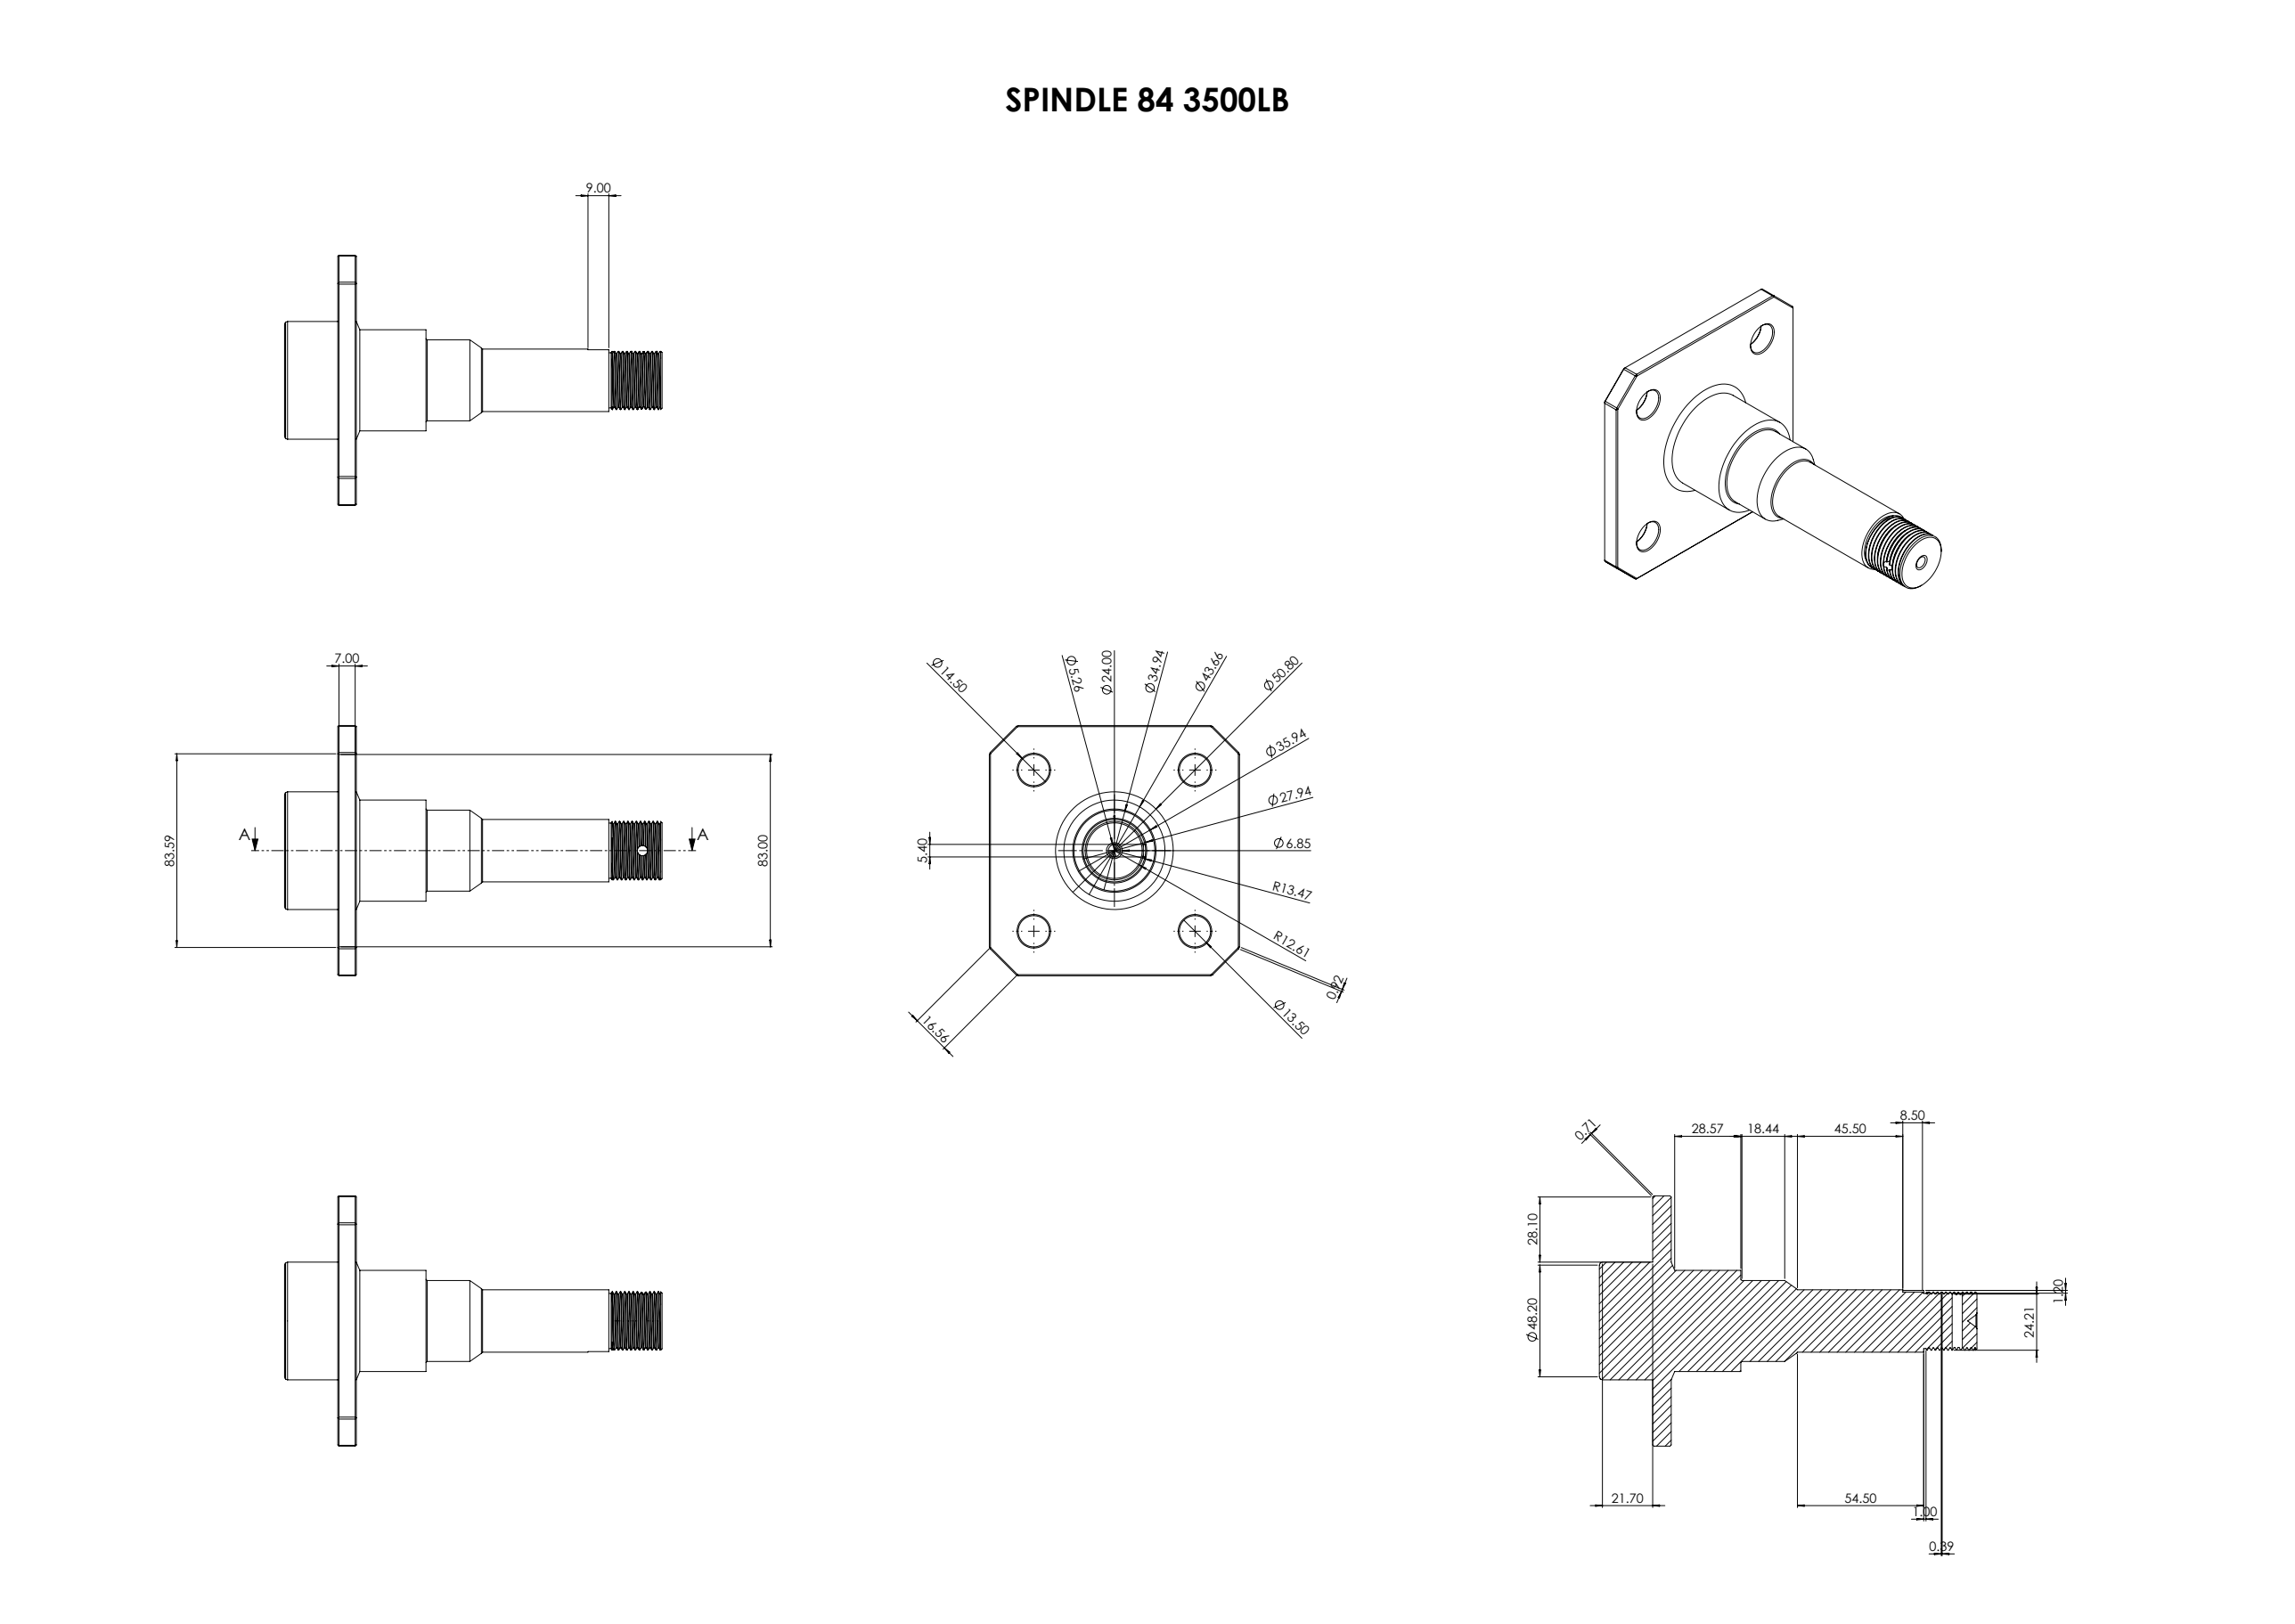
ISO-10303-21;
HEADER;
/* Generated by software containing ST-Developer
 * from STEP Tools, Inc. (www.steptools.com) 
 */

FILE_DESCRIPTION(
/* description */ (''),
/* implementation_level */ '2;1');

FILE_NAME(
/* name */ '10_Spindle_84_3500lb.step',
/* time_stamp */ '2026-10-25T01:26:34-07:00',
/* author */ (''),
/* organization */ (''),
/* preprocessor_version */ 'ST-DEVELOPER v20.2',
/* originating_system */ 'Autodesk Translation Framework v15.15.0.0',
/* authorisation */ '');

FILE_SCHEMA (('AUTOMOTIVE_DESIGN { 1 0 10303 214 3 1 1 }'));
ENDSEC;

DATA;
#10=MECHANICAL_DESIGN_GEOMETRIC_PRESENTATION_REPRESENTATION('',(#322),#71628);
#181=(
BOUNDED_CURVE()
B_SPLINE_CURVE(2,(#57816,#57817,#57818),.UNSPECIFIED.,.F.,.F.)
B_SPLINE_CURVE_WITH_KNOTS((3,3),(0.0552009552934231,0.395576151489963),
 .UNSPECIFIED.)
CURVE()
GEOMETRIC_REPRESENTATION_ITEM()
RATIONAL_B_SPLINE_CURVE((1.00343876873283,1.01256123126711,1.00343876873283))
REPRESENTATION_ITEM('')
);
#182=(
BOUNDED_CURVE()
B_SPLINE_CURVE(2,(#57942,#57943,#57944),.UNSPECIFIED.,.F.,.F.)
B_SPLINE_CURVE_WITH_KNOTS((3,3),(0.0550683626555145,0.394625977980432),
 .UNSPECIFIED.)
CURVE()
GEOMETRIC_REPRESENTATION_ITEM()
RATIONAL_B_SPLINE_CURVE((1.00343876873282,1.01256123126706,1.00343876873282))
REPRESENTATION_ITEM('')
);
#275=B_SPLINE_SURFACE_WITH_KNOTS('',3,3,((#53607,#53608,#53609,#53610,#53611,
#53612,#53613,#53614,#53615),(#53616,#53617,#53618,#53619,#53620,#53621,
#53622,#53623,#53624),(#53625,#53626,#53627,#53628,#53629,#53630,#53631,
#53632,#53633),(#53634,#53635,#53636,#53637,#53638,#53639,#53640,#53641,
#53642)),.UNSPECIFIED.,.F.,.F.,.F.,(4,4),(4,1,1,1,1,1,4),(0.,0.117317574699332),
(58.2563833255769,58.586820436873,59.2476946594652,59.5781317707613,60.2390059933534,
60.8998802159456,61.2303173272417),.UNSPECIFIED.);
#276=B_SPLINE_SURFACE_WITH_KNOTS('',3,3,((#53715,#53716,#53717,#53718,#53719,
#53720,#53721,#53722,#53723,#53724,#53725,#53726,#53727,#53728,#53729,#53730,
#53731,#53732,#53733,#53734,#53735,#53736,#53737,#53738,#53739,#53740,#53741,
#53742,#53743,#53744,#53745,#53746,#53747,#53748,#53749,#53750,#53751,#53752,
#53753,#53754,#53755,#53756,#53757,#53758,#53759,#53760,#53761),(#53762,
#53763,#53764,#53765,#53766,#53767,#53768,#53769,#53770,#53771,#53772,#53773,
#53774,#53775,#53776,#53777,#53778,#53779,#53780,#53781,#53782,#53783,#53784,
#53785,#53786,#53787,#53788,#53789,#53790,#53791,#53792,#53793,#53794,#53795,
#53796,#53797,#53798,#53799,#53800,#53801,#53802,#53803,#53804,#53805,#53806,
#53807,#53808),(#53809,#53810,#53811,#53812,#53813,#53814,#53815,#53816,
#53817,#53818,#53819,#53820,#53821,#53822,#53823,#53824,#53825,#53826,#53827,
#53828,#53829,#53830,#53831,#53832,#53833,#53834,#53835,#53836,#53837,#53838,
#53839,#53840,#53841,#53842,#53843,#53844,#53845,#53846,#53847,#53848,#53849,
#53850,#53851,#53852,#53853,#53854,#53855),(#53856,#53857,#53858,#53859,
#53860,#53861,#53862,#53863,#53864,#53865,#53866,#53867,#53868,#53869,#53870,
#53871,#53872,#53873,#53874,#53875,#53876,#53877,#53878,#53879,#53880,#53881,
#53882,#53883,#53884,#53885,#53886,#53887,#53888,#53889,#53890,#53891,#53892,
#53893,#53894,#53895,#53896,#53897,#53898,#53899,#53900,#53901,#53902)),
 .UNSPECIFIED.,.F.,.F.,.F.,(4,4),(4,1,1,1,1,1,1,1,1,1,1,1,1,1,1,1,1,1,1,
1,1,1,1,1,1,1,1,1,1,1,1,1,1,1,1,1,1,1,1,1,1,1,1,1,4),(0.,0.117317574699332),
(61.2845034392321,61.7747737335008,62.2650440277695,62.7553143220381,63.2455846163068,
63.7358549105755,64.2261252048442,64.7163954991129,65.2066657933815,65.6969360876502,
66.1872063819189,66.6774766761876,67.1677469704563,67.6580172647249,68.1482875589936,
68.6385578532623,69.128828147531,69.6190984417997,70.1093687360683,70.599639030337,
71.0899093246057,71.5801796188744,72.0704499131431,72.5607202074117,73.0509905016804,
73.5412607959491,74.0315310902178,74.5218013844865,75.0120716787551,75.5023419730238,
75.9926122672925,76.4828825615612,76.9731528558299,77.4634231500985,77.9536934443672,
78.4439637386359,78.9342340329046,79.4245043271733,79.9147746214419,80.4050449157106,
80.8953152099793,81.385585504248,81.8758557985167,82.3661260927854,82.856396387054),
 .UNSPECIFIED.);
#277=B_SPLINE_SURFACE_WITH_KNOTS('',3,3,((#54341,#54342,#54343,#54344,#54345,
#54346,#54347,#54348,#54349,#54350,#54351,#54352,#54353,#54354,#54355,#54356,
#54357,#54358,#54359,#54360,#54361,#54362,#54363,#54364,#54365,#54366,#54367,
#54368,#54369,#54370,#54371,#54372,#54373,#54374,#54375,#54376,#54377,#54378,
#54379,#54380,#54381,#54382,#54383,#54384,#54385,#54386,#54387,#54388,#54389,
#54390,#54391,#54392,#54393,#54394,#54395,#54396,#54397,#54398,#54399,#54400,
#54401,#54402,#54403,#54404,#54405,#54406,#54407,#54408,#54409,#54410,#54411,
#54412,#54413,#54414,#54415,#54416,#54417,#54418,#54419,#54420,#54421,#54422,
#54423,#54424,#54425),(#54426,#54427,#54428,#54429,#54430,#54431,#54432,
#54433,#54434,#54435,#54436,#54437,#54438,#54439,#54440,#54441,#54442,#54443,
#54444,#54445,#54446,#54447,#54448,#54449,#54450,#54451,#54452,#54453,#54454,
#54455,#54456,#54457,#54458,#54459,#54460,#54461,#54462,#54463,#54464,#54465,
#54466,#54467,#54468,#54469,#54470,#54471,#54472,#54473,#54474,#54475,#54476,
#54477,#54478,#54479,#54480,#54481,#54482,#54483,#54484,#54485,#54486,#54487,
#54488,#54489,#54490,#54491,#54492,#54493,#54494,#54495,#54496,#54497,#54498,
#54499,#54500,#54501,#54502,#54503,#54504,#54505,#54506,#54507,#54508,#54509,
#54510),(#54511,#54512,#54513,#54514,#54515,#54516,#54517,#54518,#54519,
#54520,#54521,#54522,#54523,#54524,#54525,#54526,#54527,#54528,#54529,#54530,
#54531,#54532,#54533,#54534,#54535,#54536,#54537,#54538,#54539,#54540,#54541,
#54542,#54543,#54544,#54545,#54546,#54547,#54548,#54549,#54550,#54551,#54552,
#54553,#54554,#54555,#54556,#54557,#54558,#54559,#54560,#54561,#54562,#54563,
#54564,#54565,#54566,#54567,#54568,#54569,#54570,#54571,#54572,#54573,#54574,
#54575,#54576,#54577,#54578,#54579,#54580,#54581,#54582,#54583,#54584,#54585,
#54586,#54587,#54588,#54589,#54590,#54591,#54592,#54593,#54594,#54595),
(#54596,#54597,#54598,#54599,#54600,#54601,#54602,#54603,#54604,#54605,
#54606,#54607,#54608,#54609,#54610,#54611,#54612,#54613,#54614,#54615,#54616,
#54617,#54618,#54619,#54620,#54621,#54622,#54623,#54624,#54625,#54626,#54627,
#54628,#54629,#54630,#54631,#54632,#54633,#54634,#54635,#54636,#54637,#54638,
#54639,#54640,#54641,#54642,#54643,#54644,#54645,#54646,#54647,#54648,#54649,
#54650,#54651,#54652,#54653,#54654,#54655,#54656,#54657,#54658,#54659,#54660,
#54661,#54662,#54663,#54664,#54665,#54666,#54667,#54668,#54669,#54670,#54671,
#54672,#54673,#54674,#54675,#54676,#54677,#54678,#54679,#54680)),
 .UNSPECIFIED.,.F.,.F.,.F.,(4,4),(4,1,1,1,1,1,1,1,1,1,1,1,1,1,1,1,1,1,1,
1,1,1,1,1,1,1,1,1,1,1,1,1,1,1,1,1,1,1,1,1,1,1,1,1,1,1,1,1,1,1,1,1,1,1,1,
1,1,1,1,1,1,1,1,1,1,1,1,1,1,1,1,1,1,1,1,1,1,1,1,1,1,1,4),(0.,0.117317574699332),
(8.304938233291,8.79653306474967,9.28812789620834,9.77972272766701,10.2713175591257,
10.7629123905843,11.254507222043,11.7461020535017,12.2376968849604,12.729291716419,
13.2208865478777,13.7124813793364,14.204076210795,14.6956710422537,15.1872658737124,
15.678860705171,16.1704555366297,16.6620503680884,17.153645199547,17.6452400310057,
18.1368348624644,18.628429693923,19.1200245253817,19.6116193568404,20.103214188299,
20.5948090197577,21.0864038512164,21.5779986826751,22.0695935141337,22.5611883455924,
23.0527831770511,23.5443780085097,24.0359728399684,24.5275676714271,25.0191625028857,
25.5107573343444,26.0023521658031,26.4939469972617,26.9855418287204,27.4771366601791,
27.9687314916377,28.4603263230964,28.9519211545551,29.4435159860138,29.9351108174724,
30.4267056489311,30.9183004803898,31.4098953118484,31.9014901433071,32.3930849747658,
32.8846798062244,33.3762746376831,33.8678694691418,34.3594643006004,34.8510591320591,
35.3426539635178,35.8342487949764,36.3258436264351,36.8174384578938,37.3090332893524,
37.8006281208111,38.2922229522698,38.7838177837285,39.2754126151871,39.7670074466458,
40.2586022781045,40.7501971095631,41.2417919410218,41.7333867724805,42.2249816039391,
42.7165764353978,43.2081712668565,43.6997660983151,44.1913609297738,44.6829557612325,
45.1745505926911,45.6661454241498,46.1577402556085,46.6493350870672,47.1409299185258,
47.6325247499845,48.1241195814432,48.6157144129018),.UNSPECIFIED.);
#278=B_SPLINE_SURFACE_WITH_KNOTS('',3,3,((#55387,#55388,#55389,#55390,#55391,
#55392,#55393,#55394,#55395),(#55396,#55397,#55398,#55399,#55400,#55401,
#55402,#55403,#55404),(#55405,#55406,#55407,#55408,#55409,#55410,#55411,
#55412,#55413),(#55414,#55415,#55416,#55417,#55418,#55419,#55420,#55421,
#55422)),.UNSPECIFIED.,.F.,.F.,.F.,(4,4),(4,1,1,1,1,1,4),(0.,0.117317574699332),
(48.7821842940486,49.4244050727166,49.7455154620506,50.0666258513846,50.7088466300525,
51.0299570193865,51.6721777980545),.UNSPECIFIED.);
#279=B_SPLINE_SURFACE_WITH_KNOTS('',3,3,((#55476,#55477,#55478,#55479,#55480,
#55481,#55482,#55483,#55484),(#55485,#55486,#55487,#55488,#55489,#55490,
#55491,#55492,#55493),(#55494,#55495,#55496,#55497,#55498,#55499,#55500,
#55501,#55502),(#55503,#55504,#55505,#55506,#55507,#55508,#55509,#55510,
#55511)),.UNSPECIFIED.,.F.,.F.,.F.,(4,4),(4,1,1,1,1,1,4),(0.,0.117317574699332),
(52.0050602882015,52.6272969542447,52.9384152872664,53.249533620288,53.8717702863312,
54.4940069523745,54.8051252853961),.UNSPECIFIED.);
#280=B_SPLINE_SURFACE_WITH_KNOTS('',3,3,((#55573,#55574,#55575,#55576,#55577,
#55578,#55579,#55580,#55581),(#55582,#55583,#55584,#55585,#55586,#55587,
#55588,#55589,#55590),(#55591,#55592,#55593,#55594,#55595,#55596,#55597,
#55598,#55599),(#55600,#55601,#55602,#55603,#55604,#55605,#55606,#55607,
#55608)),.UNSPECIFIED.,.F.,.F.,.F.,(4,4),(4,1,1,1,1,1,4),(0.,0.117317574699332),
(55.1490525302778,55.4633418551201,56.0919205048047,56.7204991544894,57.0347884793317,
57.349077804174,57.9776564538586),.UNSPECIFIED.);
#281=B_SPLINE_SURFACE_WITH_KNOTS('',3,3,((#55670,#55671,#55672,#55673,#55674,
#55675,#55676,#55677,#55678,#55679,#55680,#55681,#55682,#55683,#55684,#55685,
#55686,#55687,#55688,#55689,#55690,#55691,#55692,#55693,#55694,#55695,#55696,
#55697,#55698,#55699,#55700,#55701,#55702,#55703,#55704,#55705,#55706,#55707,
#55708,#55709,#55710,#55711,#55712,#55713,#55714,#55715,#55716),(#55717,
#55718,#55719,#55720,#55721,#55722,#55723,#55724,#55725,#55726,#55727,#55728,
#55729,#55730,#55731,#55732,#55733,#55734,#55735,#55736,#55737,#55738,#55739,
#55740,#55741,#55742,#55743,#55744,#55745,#55746,#55747,#55748,#55749,#55750,
#55751,#55752,#55753,#55754,#55755,#55756,#55757,#55758,#55759,#55760,#55761,
#55762,#55763),(#55764,#55765,#55766,#55767,#55768,#55769,#55770,#55771,
#55772,#55773,#55774,#55775,#55776,#55777,#55778,#55779,#55780,#55781,#55782,
#55783,#55784,#55785,#55786,#55787,#55788,#55789,#55790,#55791,#55792,#55793,
#55794,#55795,#55796,#55797,#55798,#55799,#55800,#55801,#55802,#55803,#55804,
#55805,#55806,#55807,#55808,#55809,#55810),(#55811,#55812,#55813,#55814,
#55815,#55816,#55817,#55818,#55819,#55820,#55821,#55822,#55823,#55824,#55825,
#55826,#55827,#55828,#55829,#55830,#55831,#55832,#55833,#55834,#55835,#55836,
#55837,#55838,#55839,#55840,#55841,#55842,#55843,#55844,#55845,#55846,#55847,
#55848,#55849,#55850,#55851,#55852,#55853,#55854,#55855,#55856,#55857)),
 .UNSPECIFIED.,.F.,.F.,.F.,(4,4),(4,1,1,1,1,1,1,1,1,1,1,1,1,1,1,1,1,1,1,
1,1,1,1,1,1,1,1,1,1,1,1,1,1,1,1,1,1,1,1,1,1,1,1,1,4),(0.,0.117317574699332),
(64.4256593907634,64.920671977511,65.4156845642586,65.9106971510062,66.4057097377538,
66.9007223245014,67.3957349112491,67.8907474979967,68.3857600847443,68.8807726714919,
69.3757852582395,69.8707978449871,70.3658104317347,70.8608230184823,71.3558356052299,
71.8508481919775,72.3458607787251,72.8408733654727,73.3358859522203,73.8308985389679,
74.3259111257155,74.8209237124631,75.3159362992107,75.8109488859583,76.3059614727059,
76.8009740594535,77.2959866462011,77.7909992329487,78.2860118196963,78.7810244064439,
79.2760369931915,79.7710495799391,80.2660621666867,80.7610747534343,81.2560873401819,
81.7510999269296,82.2461125136772,82.7411251004248,83.2361376871724,83.73115027392,
84.2261628606676,84.7211754474152,85.2161880341628,85.7112006209104,86.206213207658),
 .UNSPECIFIED.);
#282=B_SPLINE_SURFACE_WITH_KNOTS('',3,3,((#56291,#56292,#56293,#56294,#56295,
#56296,#56297,#56298,#56299),(#56300,#56301,#56302,#56303,#56304,#56305,
#56306,#56307,#56308),(#56309,#56310,#56311,#56312,#56313,#56314,#56315,
#56316,#56317),(#56318,#56319,#56320,#56321,#56322,#56323,#56324,#56325,
#56326)),.UNSPECIFIED.,.F.,.F.,.F.,(4,4),(4,1,1,1,1,1,4),(0.,0.117317574699332),
(61.413786866147,61.742287519182,62.399288825252,62.727789478287,63.384790784357,
64.041792090427,64.370292743462),.UNSPECIFIED.);
#283=B_SPLINE_SURFACE_WITH_KNOTS('',3,3,((#56383,#56384,#56385,#56386,#56387,
#56388,#56389,#56390,#56391),(#56392,#56393,#56394,#56395,#56396,#56397,
#56398,#56399,#56400),(#56401,#56402,#56403,#56404,#56405,#56406,#56407,
#56408,#56409),(#56410,#56411,#56412,#56413,#56414,#56415,#56416,#56417,
#56418)),.UNSPECIFIED.,.F.,.F.,.F.,(4,4),(4,1,1,1,1,1,4),(0.,0.117317574699332),
(58.294224706896,58.9183499948197,59.2304126387815,59.5424752827434,60.166600570667,
60.7907258585907,61.1027885025526),.UNSPECIFIED.);
#284=B_SPLINE_SURFACE_WITH_KNOTS('',3,3,((#56480,#56481,#56482,#56483,#56484,
#56485,#56486,#56487,#56488,#56489,#56490,#56491,#56492,#56493,#56494,#56495,
#56496,#56497,#56498,#56499,#56500,#56501,#56502,#56503,#56504,#56505,#56506,
#56507,#56508,#56509,#56510,#56511,#56512,#56513,#56514,#56515,#56516,#56517,
#56518,#56519,#56520,#56521,#56522,#56523,#56524,#56525,#56526,#56527,#56528,
#56529,#56530,#56531,#56532,#56533,#56534,#56535,#56536,#56537,#56538,#56539,
#56540,#56541,#56542,#56543,#56544,#56545,#56546,#56547,#56548,#56549,#56550,
#56551,#56552,#56553,#56554,#56555,#56556,#56557,#56558,#56559,#56560,#56561,
#56562,#56563,#56564),(#56565,#56566,#56567,#56568,#56569,#56570,#56571,
#56572,#56573,#56574,#56575,#56576,#56577,#56578,#56579,#56580,#56581,#56582,
#56583,#56584,#56585,#56586,#56587,#56588,#56589,#56590,#56591,#56592,#56593,
#56594,#56595,#56596,#56597,#56598,#56599,#56600,#56601,#56602,#56603,#56604,
#56605,#56606,#56607,#56608,#56609,#56610,#56611,#56612,#56613,#56614,#56615,
#56616,#56617,#56618,#56619,#56620,#56621,#56622,#56623,#56624,#56625,#56626,
#56627,#56628,#56629,#56630,#56631,#56632,#56633,#56634,#56635,#56636,#56637,
#56638,#56639,#56640,#56641,#56642,#56643,#56644,#56645,#56646,#56647,#56648,
#56649),(#56650,#56651,#56652,#56653,#56654,#56655,#56656,#56657,#56658,
#56659,#56660,#56661,#56662,#56663,#56664,#56665,#56666,#56667,#56668,#56669,
#56670,#56671,#56672,#56673,#56674,#56675,#56676,#56677,#56678,#56679,#56680,
#56681,#56682,#56683,#56684,#56685,#56686,#56687,#56688,#56689,#56690,#56691,
#56692,#56693,#56694,#56695,#56696,#56697,#56698,#56699,#56700,#56701,#56702,
#56703,#56704,#56705,#56706,#56707,#56708,#56709,#56710,#56711,#56712,#56713,
#56714,#56715,#56716,#56717,#56718,#56719,#56720,#56721,#56722,#56723,#56724,
#56725,#56726,#56727,#56728,#56729,#56730,#56731,#56732,#56733,#56734),
(#56735,#56736,#56737,#56738,#56739,#56740,#56741,#56742,#56743,#56744,
#56745,#56746,#56747,#56748,#56749,#56750,#56751,#56752,#56753,#56754,#56755,
#56756,#56757,#56758,#56759,#56760,#56761,#56762,#56763,#56764,#56765,#56766,
#56767,#56768,#56769,#56770,#56771,#56772,#56773,#56774,#56775,#56776,#56777,
#56778,#56779,#56780,#56781,#56782,#56783,#56784,#56785,#56786,#56787,#56788,
#56789,#56790,#56791,#56792,#56793,#56794,#56795,#56796,#56797,#56798,#56799,
#56800,#56801,#56802,#56803,#56804,#56805,#56806,#56807,#56808,#56809,#56810,
#56811,#56812,#56813,#56814,#56815,#56816,#56817,#56818,#56819)),
 .UNSPECIFIED.,.F.,.F.,.F.,(4,4),(4,1,1,1,1,1,1,1,1,1,1,1,1,1,1,1,1,1,1,
1,1,1,1,1,1,1,1,1,1,1,1,1,1,1,1,1,1,1,1,1,1,1,1,1,1,1,1,1,1,1,1,1,1,1,1,
1,1,1,1,1,1,1,1,1,1,1,1,1,1,1,1,1,1,1,1,1,1,1,1,1,1,1,4),(0.,0.117317574699332),
(11.654755053895,12.1440162165507,12.6332773792065,13.1225385418623,13.611799704518,
14.1010608671738,14.5903220298296,15.0795831924853,15.5688443551411,16.0581055177969,
16.5473666804527,17.0366278431084,17.5258890057642,18.01515016842,18.5044113310757,
18.9936724937315,19.4829336563873,19.972194819043,20.4614559816988,20.9507171443546,
21.4399783070103,21.9292394696661,22.4185006323219,22.9077617949777,23.3970229576334,
23.8862841202892,24.375545282945,24.8648064456007,25.3540676082565,25.8433287709123,
26.332589933568,26.8218510962238,27.3111122588796,27.8003734215353,28.2896345841911,
28.7788957468469,29.2681569095027,29.7574180721584,30.2466792348142,30.73594039747,
31.2252015601257,31.7144627227815,32.2037238854373,32.692985048093,33.1822462107488,
33.6715073734046,34.1607685360603,34.6500296987161,35.1392908613719,35.6285520240277,
36.1178131866834,36.6070743493392,37.096335511995,37.5855966746507,38.0748578373065,
38.5641189999623,39.053380162618,39.5426413252738,40.0319024879296,40.5211636505854,
41.0104248132411,41.4996859758969,41.9889471385527,42.4782083012084,42.9674694638642,
43.45673062652,43.9459917891757,44.4352529518315,44.9245141144873,45.413775277143,
45.9030364397988,46.3922976024546,46.8815587651103,47.3708199277661,47.8600810904219,
48.3493422530777,48.8386034157334,49.3278645783892,49.817125741045,50.3063869037007,
50.7956480663565,51.2849092290123,51.774170391668),.UNSPECIFIED.);
#285=B_SPLINE_SURFACE_WITH_KNOTS('',3,3,((#57528,#57529,#57530,#57531,#57532,
#57533,#57534,#57535,#57536),(#57537,#57538,#57539,#57540,#57541,#57542,
#57543,#57544,#57545),(#57546,#57547,#57548,#57549,#57550,#57551,#57552,
#57553,#57554),(#57555,#57556,#57557,#57558,#57559,#57560,#57561,#57562,
#57563)),.UNSPECIFIED.,.F.,.F.,.F.,(4,4),(4,1,1,1,1,1,4),(0.,0.117317574699332),
(51.9058023205642,52.230691972308,52.8804712757956,53.2053609275394,53.855140231027,
54.1800298827708,54.8298091862584),.UNSPECIFIED.);
#286=B_SPLINE_SURFACE_WITH_KNOTS('',3,3,((#57698,#57699,#57700,#57701,#57702,
#57703,#57704,#57705,#57706),(#57707,#57708,#57709,#57710,#57711,#57712,
#57713,#57714,#57715),(#57716,#57717,#57718,#57719,#57720,#57721,#57722,
#57723,#57724),(#57725,#57726,#57727,#57728,#57729,#57730,#57731,#57732,
#57733)),.UNSPECIFIED.,.F.,.F.,.F.,(4,4),(4,1,1,1,1,1,4),(0.,0.117317574699332),
(55.1300987113493,55.4429246232081,56.0685764469255,56.3814023587843,57.0070541825018,
57.3198800943605,57.945531918078),.UNSPECIFIED.);
#296=SHAPE_REPRESENTATION_RELATIONSHIP('SRR','None',#71684,#309);
#309=ADVANCED_BREP_SHAPE_REPRESENTATION('',(#335),#71616);
#322=STYLED_ITEM('',(#71804),#335);
#335=MANIFOLD_SOLID_BREP('Body1',#34209);
#357=B_SPLINE_CURVE_WITH_KNOTS('',3,(#52958,#52959,#52960,#52961,#52962,
#52963,#52964,#52965,#52966,#52967,#52968,#52969,#52970),.UNSPECIFIED.,
 .F.,.F.,(4,1,1,1,1,1,1,1,1,1,4),(47.1238898038469,47.3708199277661,47.8600810904219,
48.3493422530777,48.8386034157334,49.3278645783892,49.817125741045,50.3063869037007,
50.7956480663565,51.2849092290123,51.6964060964814),.UNSPECIFIED.);
#358=B_SPLINE_CURVE_WITH_KNOTS('',3,(#52972,#52973,#52974,#52975),
 .UNSPECIFIED.,.F.,.F.,(4,4),(0.11224113270863,0.157354351022216),
 .UNSPECIFIED.);
#359=B_SPLINE_CURVE_WITH_KNOTS('',3,(#52977,#52978,#52979,#52980,#52981,
#52982,#52983,#52984,#52985),.UNSPECIFIED.,.F.,.F.,(4,1,1,1,1,1,4),(48.7821842940486,
49.4244050727166,49.7455154620506,50.0666258513846,50.7088466300525,51.0299570193865,
51.6721777980545),.UNSPECIFIED.);
#360=B_SPLINE_CURVE_WITH_KNOTS('',3,(#52987,#52988,#52989,#52990,#52991,
#52992),.UNSPECIFIED.,.F.,.F.,(4,2,4),(0.997055295420078,1.08014136000988,
1.09793883659407),.UNSPECIFIED.);
#361=B_SPLINE_CURVE_WITH_KNOTS('',3,(#52994,#52995,#52996,#52997,#52998,
#52999),.UNSPECIFIED.,.F.,.F.,(4,2,4),(0.906540457062692,0.913969230830279,
0.997055295420078),.UNSPECIFIED.);
#362=B_SPLINE_CURVE_WITH_KNOTS('',3,(#53000,#53001,#53002,#53003,#53004,
#53005,#53006),.UNSPECIFIED.,.F.,.F.,(4,1,1,1,4),(47.1238898038469,47.1409299185258,
47.6325247499845,48.1241195814432,48.6157144129018),.UNSPECIFIED.);
#363=B_SPLINE_CURVE_WITH_KNOTS('',3,(#53011,#53012,#53013,#53014,#53015,
#53016,#53017,#53018,#53019,#53020,#53021,#53022,#53023,#53024,#53025,#53026,
#53027),.UNSPECIFIED.,.F.,.F.,(4,1,1,1,1,1,1,1,1,1,1,1,1,1,4),(40.8407044966673,
41.0104248132411,41.4996859758969,41.9889471385527,42.4782083012084,42.9674694638642,
43.45673062652,43.9459917891757,44.4352529518315,44.9245141144873,45.413775277143,
45.9030364397988,46.3922976024546,46.8815587651103,47.1238898038469),
 .UNSPECIFIED.);
#364=B_SPLINE_CURVE_WITH_KNOTS('',3,(#53028,#53029,#53030,#53031,#53032,
#53033,#53034,#53035,#53036,#53037,#53038,#53039,#53040,#53041,#53042,#53043),
 .UNSPECIFIED.,.F.,.F.,(4,1,1,1,1,1,1,1,1,1,1,1,1,4),(40.8407044966673,
41.2417919410218,41.7333867724805,42.2249816039391,42.7165764353978,43.2081712668565,
43.6997660983151,44.1913609297738,44.6829557612325,45.1745505926911,45.6661454241498,
46.1577402556085,46.6493350870672,47.1238898038469),.UNSPECIFIED.);
#365=B_SPLINE_CURVE_WITH_KNOTS('',3,(#53048,#53049,#53050,#53051,#53052,
#53053,#53054,#53055,#53056,#53057,#53058,#53059,#53060,#53061,#53062,#53063,
#53064),.UNSPECIFIED.,.F.,.F.,(4,1,1,1,1,1,1,1,1,1,1,1,1,1,4),(34.5575191894877,
34.6500296987161,35.1392908613719,35.6285520240277,36.1178131866834,36.6070743493392,
37.096335511995,37.5855966746507,38.0748578373065,38.5641189999623,39.053380162618,
39.5426413252738,40.0319024879296,40.5211636505854,40.8407044966673),
 .UNSPECIFIED.);
#366=B_SPLINE_CURVE_WITH_KNOTS('',3,(#53065,#53066,#53067,#53068,#53069,
#53070,#53071,#53072,#53073,#53074,#53075,#53076,#53077,#53078,#53079,#53080,
#53081),.UNSPECIFIED.,.F.,.F.,(4,1,1,1,1,1,1,1,1,1,1,1,1,1,4),(34.5575191894877,
34.8510591320591,35.3426539635178,35.8342487949764,36.3258436264351,36.8174384578938,
37.3090332893524,37.8006281208111,38.2922229522698,38.7838177837285,39.2754126151871,
39.7670074466458,40.2586022781045,40.7501971095631,40.8407044966673),
 .UNSPECIFIED.);
#367=B_SPLINE_CURVE_WITH_KNOTS('',3,(#53086,#53087,#53088,#53089,#53090,
#53091,#53092,#53093,#53094,#53095,#53096,#53097,#53098,#53099,#53100,#53101,
#53102),.UNSPECIFIED.,.F.,.F.,(4,1,1,1,1,1,1,1,1,1,1,1,1,1,4),(28.2743338823081,
28.2896345841911,28.7788957468469,29.2681569095027,29.7574180721584,30.2466792348142,
30.73594039747,31.2252015601257,31.7144627227815,32.2037238854373,32.692985048093,
33.1822462107488,33.6715073734046,34.1607685360603,34.5575191894877),
 .UNSPECIFIED.);
#368=B_SPLINE_CURVE_WITH_KNOTS('',3,(#53103,#53104,#53105,#53106,#53107,
#53108,#53109,#53110,#53111,#53112,#53113,#53114,#53115,#53116,#53117,#53118,
#53119),.UNSPECIFIED.,.F.,.F.,(4,1,1,1,1,1,1,1,1,1,1,1,1,1,4),(28.2743338823081,
28.4603263230964,28.9519211545551,29.4435159860138,29.9351108174724,30.4267056489311,
30.9183004803898,31.4098953118484,31.9014901433071,32.3930849747658,32.8846798062244,
33.3762746376831,33.8678694691418,34.3594643006004,34.5575191894877),
 .UNSPECIFIED.);
#369=B_SPLINE_CURVE_WITH_KNOTS('',3,(#53124,#53125,#53126,#53127,#53128,
#53129,#53130,#53131,#53132,#53133,#53134,#53135,#53136,#53137,#53138,#53139),
 .UNSPECIFIED.,.F.,.F.,(4,1,1,1,1,1,1,1,1,1,1,1,1,4),(21.9911485751285,
22.4185006323219,22.9077617949777,23.3970229576334,23.8862841202892,24.375545282945,
24.8648064456007,25.3540676082565,25.8433287709123,26.332589933568,26.8218510962238,
27.3111122588796,27.8003734215353,28.2743338823081),.UNSPECIFIED.);
#370=B_SPLINE_CURVE_WITH_KNOTS('',3,(#53140,#53141,#53142,#53143,#53144,
#53145,#53146,#53147,#53148,#53149,#53150,#53151,#53152,#53153,#53154,#53155,
#53156),.UNSPECIFIED.,.F.,.F.,(4,1,1,1,1,1,1,1,1,1,1,1,1,1,4),(21.9911485751285,
22.0695935141337,22.5611883455924,23.0527831770511,23.5443780085097,24.0359728399684,
24.5275676714271,25.0191625028857,25.5107573343444,26.0023521658031,26.4939469972617,
26.9855418287204,27.4771366601791,27.9687314916377,28.2743338823081),
 .UNSPECIFIED.);
#371=B_SPLINE_CURVE_WITH_KNOTS('',3,(#53161,#53162,#53163,#53164,#53165,
#53166,#53167,#53168,#53169,#53170,#53171,#53172,#53173,#53174,#53175,#53176,
#53177),.UNSPECIFIED.,.F.,.F.,(4,1,1,1,1,1,1,1,1,1,1,1,1,1,4),(15.707963267949,
16.0581055177969,16.5473666804527,17.0366278431084,17.5258890057642,18.01515016842,
18.5044113310757,18.9936724937315,19.4829336563873,19.972194819043,20.4614559816988,
20.9507171443546,21.4399783070103,21.9292394696661,21.9911485751285),
 .UNSPECIFIED.);
#372=B_SPLINE_CURVE_WITH_KNOTS('',3,(#53178,#53179,#53180,#53181,#53182,
#53183,#53184,#53185,#53186,#53187,#53188,#53189,#53190,#53191,#53192,#53193),
 .UNSPECIFIED.,.F.,.F.,(4,1,1,1,1,1,1,1,1,1,1,1,1,4),(15.7079632679489,
16.1704555366297,16.6620503680884,17.153645199547,17.6452400310057,18.1368348624644,
18.628429693923,19.1200245253817,19.6116193568404,20.103214188299,20.5948090197577,
21.0864038512164,21.5779986826751,21.9911485751285),.UNSPECIFIED.);
#373=B_SPLINE_CURVE_WITH_KNOTS('',3,(#53199,#53200,#53201,#53202,#53203,
#53204,#53205,#53206,#53207,#53208,#53209,#53210,#53211,#53212,#53213),
 .UNSPECIFIED.,.F.,.F.,(4,1,1,1,1,1,1,1,1,1,1,1,4),(78.5398163397448,78.7810244064439,
79.2760369931915,79.7710495799391,80.2660621666867,80.7610747534343,81.2560873401819,
81.7510999269296,82.2461125136772,82.7411251004248,83.2361376871724,83.73115027392,
84.1747579197157),.UNSPECIFIED.);
#374=B_SPLINE_CURVE_WITH_KNOTS('',3,(#53216,#53217,#53218,#53219,#53220,
#53221,#53222,#53223,#53224,#53225,#53226,#53227),.UNSPECIFIED.,.F.,.F.,
(4,1,1,1,1,1,1,1,1,4),(78.5398163397448,78.9342340329046,79.4245043271733,
79.9147746214419,80.4050449157106,80.8953152099793,81.385585504248,81.8758557985167,
82.3661260927854,82.856396387054),.UNSPECIFIED.);
#375=B_SPLINE_CURVE_WITH_KNOTS('',3,(#53232,#53233,#53234,#53235,#53236,
#53237,#53238,#53239,#53240,#53241,#53242,#53243,#53244,#53245,#53246,#53247,
#53248),.UNSPECIFIED.,.F.,.F.,(4,1,1,1,1,1,1,1,1,1,1,1,1,1,4),(72.2566310325653,
72.3458607787251,72.8408733654727,73.3358859522203,73.8308985389679,74.3259111257155,
74.8209237124631,75.3159362992107,75.8109488859583,76.3059614727059,76.8009740594535,
77.2959866462011,77.7909992329487,78.2860118196963,78.5398163397448),
 .UNSPECIFIED.);
#376=B_SPLINE_CURVE_WITH_KNOTS('',3,(#53249,#53250,#53251,#53252,#53253,
#53254,#53255,#53256,#53257,#53258,#53259,#53260,#53261,#53262,#53263,#53264,
#53265),.UNSPECIFIED.,.F.,.F.,(4,1,1,1,1,1,1,1,1,1,1,1,1,1,4),(72.2566310325653,
72.5607202074117,73.0509905016804,73.5412607959491,74.0315310902178,74.5218013844865,
75.0120716787551,75.5023419730238,75.9926122672925,76.4828825615612,76.9731528558299,
77.4634231500985,77.9536934443672,78.4439637386359,78.5398163397448),
 .UNSPECIFIED.);
#377=B_SPLINE_CURVE_WITH_KNOTS('',3,(#53270,#53271,#53272,#53273,#53274,
#53275,#53276,#53277,#53278,#53279,#53280,#53281,#53282,#53283,#53284,#53285),
 .UNSPECIFIED.,.F.,.F.,(4,1,1,1,1,1,1,1,1,1,1,1,1,4),(65.9734457253856,
66.4057097377538,66.9007223245014,67.3957349112491,67.8907474979967,68.3857600847443,
68.8807726714919,69.3757852582395,69.8707978449871,70.3658104317347,70.8608230184823,
71.3558356052299,71.8508481919775,72.2566310325653),.UNSPECIFIED.);
#378=B_SPLINE_CURVE_WITH_KNOTS('',3,(#53286,#53287,#53288,#53289,#53290,
#53291,#53292,#53293,#53294,#53295,#53296,#53297,#53298,#53299,#53300,#53301,
#53302),.UNSPECIFIED.,.F.,.F.,(4,1,1,1,1,1,1,1,1,1,1,1,1,1,4),(65.9734457253856,
66.1872063819189,66.6774766761876,67.1677469704563,67.6580172647249,68.1482875589936,
68.6385578532623,69.128828147531,69.6190984417997,70.1093687360683,70.599639030337,
71.0899093246057,71.5801796188744,72.0704499131431,72.2566310325653),
 .UNSPECIFIED.);
#379=B_SPLINE_CURVE_WITH_KNOTS('',3,(#53645,#53646,#53647,#53648,#53649,
#53650,#53651,#53652,#53653,#53654,#53655,#53656,#53657,#53658,#53659,#53660),
 .UNSPECIFIED.,.F.,.F.,(4,3,3,3,3,4),(0.,0.000595938657993939,0.0422635503527143,
0.0630916558022166,0.101044021572731,0.126729429815141),.UNSPECIFIED.);
#380=B_SPLINE_CURVE_WITH_KNOTS('',3,(#53662,#53663,#53664,#53665,#53666,
#53667,#53668,#53669,#53670),.UNSPECIFIED.,.F.,.F.,(4,1,1,1,1,1,4),(58.2972797775322,
58.586820436873,59.2476946594652,59.5781317707613,60.2390059933534,60.8998802159456,
61.1317270633727),.UNSPECIFIED.);
#381=B_SPLINE_CURVE_WITH_KNOTS('',3,(#53672,#53673,#53674,#53675,#53676,
#53677,#53678,#53679,#53680,#53681),.UNSPECIFIED.,.F.,.F.,(4,2,2,2,4),(0.000574071133364476,
0.000967589686564383,0.0339148109550191,0.0832234192490246,0.162484616113956),
 .UNSPECIFIED.);
#382=B_SPLINE_CURVE_WITH_KNOTS('',3,(#53683,#53684,#53685,#53686,#53687,
#53688,#53689,#53690,#53691,#53692,#53693,#53694,#53695),.UNSPECIFIED.,
 .F.,.F.,(4,3,3,3,4),(0.,0.00275985983460007,0.0770052601636086,0.109906700875405,
0.130628524523904),.UNSPECIFIED.);
#383=B_SPLINE_CURVE_WITH_KNOTS('',3,(#53696,#53697,#53698,#53699,#53700,
#53701,#53702,#53703,#53704,#53705,#53706,#53707,#53708,#53709,#53710,#53711,
#53712,#53713,#53714),.UNSPECIFIED.,.F.,.F.,(4,3,3,3,3,3,4),(49.9514450922859,
50.281882203582,50.9427564261742,51.2731935374703,51.9340677600624,52.5949419826546,
52.8217841885201),.UNSPECIFIED.);
#384=B_SPLINE_CURVE_WITH_KNOTS('',3,(#53905,#53906,#53907,#53908,#53909,
#53910,#53911,#53912,#53913,#53914,#53915,#53916,#53917,#53918,#53919,#53920,
#53921,#53922,#53923,#53924,#53925,#53926,#53927,#53928,#53929,#53930,#53931,
#53932,#53933,#53934,#53935,#53936,#53937,#53938,#53939,#53940,#53941,#53942,
#53943,#53944,#53945,#53946,#53947,#53948,#53949,#53950),.UNSPECIFIED.,
 .F.,.F.,(4,3,3,3,3,3,3,3,3,3,3,3,3,3,3,4),(0.,0.00275985982614405,0.0773717195497823,
0.109906700365477,0.16313770113851,0.167106859846252,0.168197417803669,
0.168838059532748,0.169391172021586,0.170064784109231,0.171335649429611,
0.178574548147706,0.187829968841971,0.233407245541387,0.305551783846953,
0.338436359320456),.UNSPECIFIED.);
#385=B_SPLINE_CURVE_WITH_KNOTS('',3,(#53952,#53953,#53954,#53955,#53956,
#53957,#53958,#53959,#53960,#53961,#53962,#53963,#53964,#53965,#53966,#53967,
#53968,#53969,#53970,#53971,#53972,#53973,#53974,#53975,#53976,#53977,#53978,
#53979,#53980,#53981,#53982,#53983,#53984,#53985,#53986,#53987,#53988,#53989,
#53990,#53991,#53992,#53993,#53994),.UNSPECIFIED.,.F.,.F.,(4,3,3,3,3,3,
3,3,3,3,3,3,3,3,4),(65.6568234492589,65.7265928569268,66.2168631511955,
66.7071334454641,67.1974037397328,67.6876740340015,68.1779443282702,68.6682146225388,
69.1584849168075,69.6487552110762,70.1390255053449,70.6292957996136,71.1195660938823,
71.6098363881509,71.6713401100588),.UNSPECIFIED.);
#386=B_SPLINE_CURVE_WITH_KNOTS('',3,(#53996,#53997,#53998,#53999,#54000,
#54001,#54002,#54003,#54004,#54005,#54006,#54007,#54008,#54009,#54010,#54011,
#54012,#54013,#54014,#54015,#54016,#54017,#54018,#54019,#54020,#54021,#54022,
#54023,#54024,#54025,#54026,#54027,#54028,#54029,#54030,#54031,#54032,#54033,
#54034,#54035,#54036,#54037,#54038,#54039,#54040,#54041),.UNSPECIFIED.,
 .F.,.F.,(4,3,3,3,3,3,3,3,3,3,3,3,3,3,3,4),(0.,0.00275985982151374,0.0771562456781327,
0.109906700101125,0.163137700733035,0.1671068594303,0.168197417389794,0.168838059129582,
0.169391171634666,0.170064783742003,0.17133564910631,0.178574548151433,
0.187829969232375,0.233407247858854,0.305703464500967,0.338436366447218),
 .UNSPECIFIED.);
#387=B_SPLINE_CURVE_WITH_KNOTS('',3,(#54043,#54044,#54045,#54046,#54047,
#54048,#54049,#54050,#54051,#54052,#54053,#54054,#54055,#54056,#54057,#54058,
#54059,#54060,#54061,#54062,#54063,#54064,#54065,#54066,#54067,#54068,#54069,
#54070,#54071,#54072,#54073,#54074,#54075,#54076,#54077,#54078,#54079,#54080,
#54081,#54082),.UNSPECIFIED.,.F.,.F.,(4,3,3,3,3,3,3,3,3,3,3,3,3,4),(59.3736381420792,
59.8433493257026,60.3336196199713,60.82388991424,61.3141602085087,61.8044305027773,
62.294700797046,62.7849710913147,63.2752413855834,63.7655116798521,64.2557819741207,
64.7460522683894,65.2363225626581,65.3881548028793),.UNSPECIFIED.);
#388=B_SPLINE_CURVE_WITH_KNOTS('',3,(#54084,#54085,#54086,#54087,#54088,
#54089,#54090,#54091,#54092,#54093,#54094,#54095,#54096,#54097,#54098,#54099,
#54100,#54101,#54102,#54103,#54104,#54105,#54106,#54107,#54108,#54109,#54110,
#54111,#54112,#54113,#54114,#54115,#54116,#54117,#54118,#54119,#54120,#54121,
#54122,#54123,#54124,#54125,#54126,#54127,#54128,#54129,#54130,#54131,#54132),
 .UNSPECIFIED.,.F.,.F.,(4,3,3,3,3,3,3,3,3,3,3,3,3,3,3,3,4),(0.,0.00275985983466315,
0.0768512497472772,0.109906700870624,0.163137701889579,0.167106860614449,
0.168197418582742,0.168838060333893,0.169391172850375,0.170064784950834,
0.171335650271267,0.178574549075021,0.187829969490077,0.233407245213584,
0.306223710050725,0.312212167181286,0.338436362006313),.UNSPECIFIED.);
#389=B_SPLINE_CURVE_WITH_KNOTS('',3,(#54134,#54135,#54136,#54137,#54138,
#54139,#54140,#54141,#54142,#54143,#54144,#54145,#54146,#54147,#54148,#54149,
#54150,#54151,#54152,#54153,#54154,#54155,#54156,#54157,#54158,#54159,#54160,
#54161,#54162,#54163,#54164,#54165,#54166,#54167,#54168,#54169,#54170,#54171,
#54172,#54173),.UNSPECIFIED.,.F.,.F.,(4,3,3,3,3,3,3,3,3,3,3,3,3,4),(53.0904528348997,
53.4698355002098,53.9601057944785,54.4503760887471,54.9406463830158,55.4309166772845,
55.9211869715532,56.4114572658219,56.9017275600905,57.3919978543592,57.8822681486279,
58.3725384428966,58.8628087371653,59.1049694956997),.UNSPECIFIED.);
#390=B_SPLINE_CURVE_WITH_KNOTS('',3,(#54175,#54176,#54177,#54178,#54179,
#54180,#54181,#54182,#54183,#54184),.UNSPECIFIED.,.F.,.F.,(4,3,3,4),(0.198401836072916,
0.23340724983945,0.304766656516156,0.338436371365031),.UNSPECIFIED.);
#391=B_SPLINE_CURVE_WITH_KNOTS('',3,(#54186,#54187,#54188,#54189,#54190,
#54191,#54192,#54193,#54194,#54195),.UNSPECIFIED.,.F.,.F.,(4,2,2,2,4),(0.,
0.00656666019327175,0.0703003168502551,0.107768285611947,0.160871499936812),
 .UNSPECIFIED.);
#392=B_SPLINE_CURVE_WITH_KNOTS('',3,(#54196,#54197,#54198,#54199,#54200,
#54201,#54202,#54203,#54204,#54205,#54206,#54207,#54208),.UNSPECIFIED.,
 .F.,.F.,(4,1,1,1,1,1,1,1,1,1,4),(61.3832284283791,61.7747737335008,62.2650440277695,
62.7553143220381,63.2455846163068,63.7358549105755,64.2261252048442,64.7163954991129,
65.2066657933815,65.6969360876502,65.9734457253856),.UNSPECIFIED.);
#393=B_SPLINE_CURVE_WITH_KNOTS('',3,(#54210,#54211,#54212,#54213,#54214,
#54215,#54216,#54217,#54218,#54219,#54220,#54221,#54222,#54223,#54224,#54225,
#54226,#54227,#54228,#54229,#54230,#54231,#54232,#54233,#54234,#54235,#54236,
#54237,#54238,#54239,#54240,#54241,#54242,#54243,#54244,#54245,#54246,#54247,
#54248,#54249,#54250,#54251,#54252,#54253,#54254,#54255,#54256,#54257,#54258,
#54259,#54260,#54261,#54262,#54263,#54264,#54265,#54266,#54267,#54268,#54269,
#54270,#54271,#54272,#54273,#54274,#54275,#54276,#54277,#54278,#54279,#54280,
#54281,#54282,#54283,#54284,#54285,#54286,#54287,#54288,#54289,#54290,#54291,
#54292,#54293,#54294,#54295,#54296,#54297,#54298,#54299,#54300,#54301,#54302,
#54303,#54304,#54305,#54306,#54307,#54308,#54309,#54310,#54311,#54312,#54313,
#54314,#54315,#54316,#54317,#54318,#54319,#54320,#54321,#54322,#54323,#54324,
#54325,#54326,#54327,#54328,#54329,#54330,#54331,#54332,#54333),
 .UNSPECIFIED.,.F.,.F.,(4,3,3,3,3,3,3,3,3,3,3,3,3,3,3,3,3,3,3,3,3,3,3,3,
3,3,3,3,3,3,3,3,3,3,3,3,3,3,3,3,3,4),(-2.4657711816956,-2.37711779550954,
-2.28851752377278,-2.22320398650821,-2.18602278417013,-2.17028473161443,
-2.15866200237192,-2.07068230873769,-1.98294419157819,-1.89589333530891,
-1.87402539857354,-1.86347823865937,-1.77633674922564,-1.76600922565624,
-1.67904910353692,-1.591716101066,-1.50460771625274,-1.41982386317424,-1.39830915580724,
-1.38520554468227,-1.29903699636726,-1.21307297743482,-1.16547230393873,
-1.07917498089865,-0.993139567163436,-0.941084428724779,-0.925274659028494,
-0.913998245978635,-0.828843082626024,-0.743624729749914,-0.659209653948047,
-0.576698459654186,-0.504611152197413,-0.473072955185075,-0.459906411912699,
-0.450573022198668,-0.366966623021441,-0.282778978986007,-0.198778607846025,
-0.115420401362767,-0.0335266982944923,0.),.UNSPECIFIED.);
#394=B_SPLINE_CURVE_WITH_KNOTS('',3,(#54334,#54335,#54336,#54337,#54338,
#54339,#54340),.UNSPECIFIED.,.F.,.F.,(4,3,4),(71.9400087564384,72.1001066824196,
72.5200028658207),.UNSPECIFIED.);
#395=B_SPLINE_CURVE_WITH_KNOTS('',3,(#54683,#54684,#54685,#54686,#54687,
#54688,#54689,#54690,#54691,#54692,#54693,#54694,#54695,#54696,#54697,#54698,
#54699,#54700,#54701,#54702,#54703,#54704,#54705,#54706,#54707,#54708,#54709,
#54710,#54711,#54712,#54713,#54714,#54715,#54716,#54717,#54718,#54719,#54720,
#54721,#54722,#54723,#54724,#54725,#54726,#54727,#54728),.UNSPECIFIED.,
 .F.,.F.,(4,3,3,3,3,3,3,3,3,3,3,3,3,3,3,4),(0.,0.00275985982436321,0.0772952705909694,
0.109906700261339,0.163137700981914,0.167106859688835,0.168197417644868,
0.168838059371253,0.169391171859311,0.170064783946173,0.171335649280755,
0.178574548125793,0.187829969035857,0.233407246747053,0.305622875587664,
0.338436362095157),.UNSPECIFIED.);
#396=B_SPLINE_CURVE_WITH_KNOTS('',3,(#54730,#54731,#54732,#54733,#54734,
#54735,#54736,#54737,#54738,#54739,#54740,#54741,#54742,#54743,#54744,#54745,
#54746,#54747,#54748),.UNSPECIFIED.,.F.,.F.,(4,3,3,3,3,3,4),(0.,0.491594831458664,
0.983189662917332,1.474784494376,1.96637932583467,2.45797415729334,2.55630173108341),
 .UNSPECIFIED.);
#397=B_SPLINE_CURVE_WITH_KNOTS('',3,(#54750,#54751,#54752,#54753,#54754,
#54755,#54756,#54757,#54758,#54759,#54760,#54761,#54762,#54763,#54764,#54765,
#54766,#54767,#54768,#54769,#54770,#54771,#54772,#54773,#54774,#54775,#54776,
#54777,#54778,#54779,#54780,#54781,#54782,#54783,#54784,#54785,#54786,#54787,
#54788,#54789,#54790,#54791,#54792,#54793,#54794,#54795,#54796,#54797,#54798,
#54799,#54800,#54801,#54802,#54803,#54804,#54805,#54806,#54807,#54808,#54809,
#54810,#54811,#54812,#54813,#54814,#54815,#54816,#54817,#54818,#54819,#54820,
#54821,#54822,#54823,#54824,#54825,#54826,#54827,#54828,#54829,#54830,#54831,
#54832,#54833,#54834,#54835,#54836,#54837,#54838,#54839,#54840,#54841,#54842,
#54843,#54844,#54845,#54846,#54847,#54848,#54849,#54850,#54851,#54852,#54853,
#54854,#54855,#54856,#54857,#54858,#54859,#54860,#54861,#54862,#54863,#54864,
#54865,#54866,#54867,#54868,#54869,#54870),.UNSPECIFIED.,.F.,.F.,(4,3,3,
3,3,3,3,3,3,3,3,3,3,3,3,3,3,3,3,3,3,3,3,3,3,3,3,3,3,3,3,3,3,3,3,3,3,3,3,
3,4),(-2.47011828786777,-2.39429498938945,-2.31085421816921,-2.2487987703988,
-2.21702958300785,-2.19665005734925,-2.18345847963518,-2.09925341052227,
-2.01449221995017,-1.92999116531367,-1.91521693514107,-1.90306118528872,
-1.81441063600599,-1.72993839179506,-1.64463244122103,-1.55899127324955,
-1.47459368269514,-1.44567397692449,-1.43778803581126,-1.35160714559026,
-1.264927968677,-1.22140091103189,-1.13509194280059,-1.04848479472449,-0.994484091434478,
-0.978663130413089,-0.969072712221302,-0.880924326267074,-0.793336817843973,
-0.704907993124182,-0.616479168404391,-0.539419272353842,-0.505705567831727,
-0.490288007695899,-0.482050594893607,-0.394957153060787,-0.306838265627068,
-0.218098308664458,-0.129586226722169,-0.0421749412600055,0.),
 .UNSPECIFIED.);
#398=B_SPLINE_CURVE_WITH_KNOTS('',3,(#54871,#54872,#54873,#54874,#54875,
#54876,#54877,#54878,#54879,#54880,#54881,#54882,#54883,#54884,#54885),
 .UNSPECIFIED.,.F.,.F.,(4,1,1,1,1,1,1,1,1,1,1,1,4),(10.3363935212333,10.7629123905843,
11.254507222043,11.7461020535017,12.2376968849604,12.729291716419,13.2208865478777,
13.7124813793364,14.204076210795,14.6956710422537,15.1872658737124,15.678860705171,
15.7079632679489),.UNSPECIFIED.);
#399=B_SPLINE_CURVE_WITH_KNOTS('',3,(#54887,#54888,#54889,#54890,#54891,
#54892),.UNSPECIFIED.,.F.,.F.,(4,2,4),(0.000204756358194638,0.0248404679347799,
0.148913229629469),.UNSPECIFIED.);
#400=B_SPLINE_CURVE_WITH_KNOTS('',3,(#54894,#54895,#54896,#54897),
 .UNSPECIFIED.,.F.,.F.,(4,4),(0.,0.00184861559299079),.UNSPECIFIED.);
#401=B_SPLINE_CURVE_WITH_KNOTS('',3,(#54899,#54900,#54901,#54902,#54903,
#54904,#54905,#54906,#54907,#54908,#54909,#54910,#54911,#54912,#54913,#54914,
#54915,#54916,#54917,#54918,#54919,#54920,#54921,#54922,#54923,#54924,#54925,
#54926,#54927,#54928,#54929,#54930,#54931,#54932,#54933,#54934,#54935,#54936,
#54937,#54938),.UNSPECIFIED.,.F.,.F.,(4,3,3,3,3,3,3,3,3,3,3,3,3,4),(34.240896913361,
34.4116382021068,34.9032330335655,35.3948278650241,35.8864226964828,36.3780175279415,
36.8696123594001,37.3612071908588,37.8528020223175,38.3443968537762,38.8359916852348,
39.3275865166935,39.8191813481521,40.255413574161),.UNSPECIFIED.);
#402=B_SPLINE_CURVE_WITH_KNOTS('',3,(#54940,#54941,#54942,#54943,#54944,
#54945,#54946,#54947,#54948,#54949,#54950,#54951,#54952,#54953,#54954,#54955,
#54956,#54957,#54958,#54959,#54960,#54961,#54962,#54963,#54964,#54965,#54966,
#54967,#54968,#54969,#54970,#54971,#54972,#54973,#54974,#54975,#54976,#54977,
#54978,#54979,#54980,#54981,#54982,#54983,#54984,#54985),.UNSPECIFIED.,
 .F.,.F.,(4,3,3,3,3,3,3,3,3,3,3,3,3,3,3,4),(0.,0.00275985982611835,0.0773912087755722,
0.109906700382361,0.163137701138107,0.167106859845295,0.168197417801363,
0.168838059529032,0.169391172014476,0.170064784081102,0.171335649356011,
0.178574547909555,0.187829967619597,0.233407240256718,0.305530899139838,
0.33843635522598),.UNSPECIFIED.);
#403=B_SPLINE_CURVE_WITH_KNOTS('',3,(#54987,#54988,#54989,#54990,#54991,
#54992,#54993,#54994,#54995,#54996,#54997,#54998,#54999,#55000,#55001,#55002,
#55003,#55004,#55005,#55006,#55007,#55008,#55009,#55010,#55011,#55012,#55013,
#55014,#55015,#55016,#55017,#55018,#55019,#55020,#55021,#55022,#55023,#55024,
#55025,#55026,#55027,#55028,#55029),.UNSPECIFIED.,.F.,.F.,(4,3,3,3,3,3,
3,3,3,3,3,3,3,3,4),(27.9577116061813,28.0209053931441,28.5125002246028,
29.0040950560614,29.4956898875201,29.9872847189788,30.4788795504374,30.9704743818961,
31.4620692133548,31.9536640448135,32.4452588762721,32.9368537077308,33.4284485391895,
33.9200433706481,33.9722282669813),.UNSPECIFIED.);
#404=B_SPLINE_CURVE_WITH_KNOTS('',3,(#55031,#55032,#55033,#55034,#55035,
#55036,#55037,#55038,#55039,#55040,#55041,#55042,#55043,#55044,#55045,#55046,
#55047,#55048,#55049,#55050,#55051,#55052,#55053,#55054,#55055,#55056,#55057,
#55058,#55059,#55060,#55061,#55062,#55063,#55064,#55065,#55066,#55067,#55068,
#55069,#55070,#55071,#55072,#55073,#55074,#55075,#55076),.UNSPECIFIED.,
 .F.,.F.,(4,3,3,3,3,3,3,3,3,3,3,3,3,3,3,4),(0.,0.00275985983231624,0.0771358287561839,
0.109906700741802,0.163137701683987,0.167106860406336,0.168197418376005,
0.168838060124296,0.169391172636416,0.170064784747918,0.171335650104608,
0.178574549108691,0.187829970005815,0.233407247867916,0.30571251857187,
0.338436366489491),.UNSPECIFIED.);
#405=B_SPLINE_CURVE_WITH_KNOTS('',3,(#55078,#55079,#55080,#55081,#55082,
#55083,#55084,#55085,#55086,#55087,#55088,#55089,#55090,#55091,#55092,#55093,
#55094,#55095,#55096,#55097,#55098,#55099,#55100,#55101,#55102,#55103,#55104,
#55105,#55106,#55107,#55108,#55109,#55110,#55111,#55112,#55113,#55114,#55115,
#55116,#55117),.UNSPECIFIED.,.F.,.F.,(4,3,3,3,3,3,3,3,3,3,3,3,3,4),(21.6745262990017,
22.1217674156401,22.6133622470988,23.1049570785574,23.5965519100161,24.0881467414748,
24.5797415729334,25.0713364043921,25.5629312358508,26.0545260673094,26.5461208987681,
27.0377157302268,27.5293105616854,27.6890429598018),.UNSPECIFIED.);
#406=B_SPLINE_CURVE_WITH_KNOTS('',3,(#55119,#55120,#55121,#55122,#55123,
#55124,#55125,#55126,#55127,#55128,#55129,#55130,#55131,#55132,#55133,#55134,
#55135,#55136,#55137,#55138,#55139,#55140,#55141,#55142,#55143,#55144,#55145,
#55146,#55147,#55148,#55149,#55150,#55151,#55152,#55153,#55154,#55155,#55156,
#55157,#55158,#55159,#55160,#55161,#55162,#55163,#55164),.UNSPECIFIED.,
 .F.,.F.,(4,3,3,3,3,3,3,3,3,3,3,3,3,3,3,4),(0.,0.00275985982612918,0.0767519898615825,
0.109906700366968,0.16313770113734,0.167106859849563,0.168197417798545,
0.168838059528161,0.169391172050885,0.170064784160668,0.171335649470964,
0.178574548234285,0.187829968981913,0.233407245948613,0.282033220718275,
0.338436360379489),.UNSPECIFIED.);
#407=B_SPLINE_CURVE_WITH_KNOTS('',3,(#55166,#55167,#55168,#55169,#55170,
#55171,#55172,#55173,#55174,#55175,#55176,#55177,#55178,#55179,#55180,#55181,
#55182,#55183,#55184,#55185,#55186,#55187,#55188,#55189,#55190,#55191,#55192,
#55193,#55194,#55195,#55196,#55197,#55198,#55199,#55200,#55201,#55202,#55203,
#55204,#55205),.UNSPECIFIED.,.F.,.F.,(4,3,3,3,3,3,3,3,3,3,3,3,3,4),(15.3913409918222,
15.7310346066774,16.2226294381361,16.7142242695947,17.2058191010534,17.6974139325121,
18.1890087639707,18.6806035954294,19.1721984268881,19.6637932583467,20.1553880898054,
20.6469829212641,21.1385777527227,21.4058576526223),.UNSPECIFIED.);
#408=B_SPLINE_CURVE_WITH_KNOTS('',3,(#55207,#55208,#55209,#55210,#55211,
#55212,#55213,#55214,#55215,#55216,#55217,#55218,#55219,#55220,#55221,#55222,
#55223,#55224,#55225,#55226,#55227,#55228,#55229,#55230,#55231,#55232,#55233,
#55234,#55235,#55236,#55237,#55238,#55239,#55240,#55241,#55242,#55243,#55244,
#55245,#55246,#55247,#55248,#55249,#55250,#55251,#55252,#55253,#55254,#55255),
 .UNSPECIFIED.,.F.,.F.,(4,3,3,3,3,3,3,3,3,3,3,3,3,3,3,3,4),(0.,0.00275985983348124,
0.0762148369746939,0.109906700802838,0.147108383127543,0.163137701785669,
0.167106860511849,0.168197418475418,0.168838060209463,0.169391172706176,
0.170064784805486,0.17133565015834,0.178574549091358,0.187829970095521,
0.233407248291307,0.304987043084035,0.338436364998264),.UNSPECIFIED.);
#409=B_SPLINE_CURVE_WITH_KNOTS('',3,(#55257,#55258,#55259,#55260,#55261,
#55262,#55263,#55264,#55265,#55266,#55267,#55268,#55269,#55270,#55271,#55272,
#55273,#55274,#55275,#55276,#55277,#55278,#55279,#55280,#55281,#55282,#55283,
#55284,#55285,#55286,#55287,#55288,#55289,#55290,#55291,#55292,#55293,#55294,
#55295,#55296),.UNSPECIFIED.,.F.,.F.,(4,3,3,3,3,3,3,3,3,3,3,3,3,4),(9.10815568464253,
9.3403017977147,9.83189662917337,10.323491460632,10.8150862920907,11.3066811235494,
11.798275955008,12.2898707864667,12.7814656179254,13.273060449384,13.7646552808427,
14.2562501123014,14.7478449437601,15.1226723454426),.UNSPECIFIED.);
#410=B_SPLINE_CURVE_WITH_KNOTS('',3,(#55298,#55299,#55300,#55301,#55302,
#55303,#55304,#55305,#55306,#55307,#55308,#55309,#55310,#55311,#55312,#55313,
#55314,#55315,#55316,#55317,#55318,#55319,#55320,#55321,#55322,#55323,#55324,
#55325,#55326,#55327,#55328,#55329,#55330,#55331,#55332,#55333,#55334,#55335,
#55336,#55337,#55338,#55339,#55340,#55341,#55342,#55343,#55344,#55345,#55346),
 .UNSPECIFIED.,.F.,.F.,(4,3,3,3,3,3,3,3,3,3,3,3,3,3,3,3,4),(0.,0.00275985982495649,
0.0117382940614391,0.0866092230060178,0.10990670029821,0.163137701034397,
0.167106859741717,0.168197417701499,0.16883805943631,0.169391171934133,
0.170064784030677,0.171335649369872,0.178574548176285,0.187829968961567,
0.233407246130877,0.305372769891771,0.338436361290398),.UNSPECIFIED.);
#411=B_SPLINE_CURVE_WITH_KNOTS('',3,(#55347,#55348,#55349,#55350,#55351,
#55352,#55353,#55354,#55355,#55356,#55357,#55358,#55359,#55360,#55361,#55362,
#55363,#55364,#55365,#55366,#55367,#55368,#55369,#55370,#55371,#55372,#55373,
#55374,#55375,#55376,#55377,#55378,#55379,#55380,#55381,#55382,#55383,#55384,
#55385,#55386),.UNSPECIFIED.,.F.,.F.,(4,3,3,3,3,3,3,3,3,3,3,3,3,4),(2.82497037746304,
2.94956898875201,3.44116382021067,3.93275865166934,4.42435348312801,4.91594831458668,
5.40754314604535,5.89913797750402,6.39073280896269,6.88232764042136,7.37392247188002,
7.86551730333869,8.35711213479736,8.8394870382631),.UNSPECIFIED.);
#412=B_SPLINE_CURVE_WITH_KNOTS('',3,(#55424,#55425,#55426,#55427,#55428,
#55429,#55430,#55431,#55432,#55433,#55434,#55435,#55436),.UNSPECIFIED.,
 .F.,.F.,(4,3,3,3,4),(0.,0.037446429103661,0.0586081614907165,0.0940217092267908,
0.11745568348674),.UNSPECIFIED.);
#413=B_SPLINE_CURVE_WITH_KNOTS('',3,(#55438,#55439,#55440,#55441,#55442,
#55443,#55444,#55445,#55446,#55447,#55448,#55449,#55450,#55451,#55452,#55453,
#55454,#55455,#55456),.UNSPECIFIED.,.F.,.F.,(4,3,3,3,3,3,4),(40.5278112792784,
41.1194668394256,41.4405772287596,41.7616876180936,42.4039083967615,42.7250187860955,
43.3613098903777),.UNSPECIFIED.);
#414=B_SPLINE_CURVE_WITH_KNOTS('',3,(#55457,#55458,#55459,#55460,#55461,
#55462,#55463,#55464,#55465,#55466,#55467,#55468,#55469,#55470,#55471,#55472,
#55473,#55474,#55475),.UNSPECIFIED.,.F.,.F.,(4,3,3,3,3,3,4),(0.,0.00617385261260148,
0.0296247466034154,0.0555909177237707,0.0757825634092935,0.10848938045471,
0.133283104059319),.UNSPECIFIED.);
#415=B_SPLINE_CURVE_WITH_KNOTS('',3,(#55514,#55515,#55516,#55517,#55518,
#55519,#55520,#55521,#55522,#55523,#55524,#55525,#55526),.UNSPECIFIED.,
 .F.,.F.,(4,3,3,3,4),(0.,0.0429420950889889,0.0600161086838339,0.10053591690027,
0.119365066230604),.UNSPECIFIED.);
#416=B_SPLINE_CURVE_WITH_KNOTS('',3,(#55528,#55529,#55530,#55531,#55532,
#55533,#55534,#55535,#55536,#55537,#55538,#55539,#55540,#55541,#55542,#55543,
#55544,#55545,#55546),.UNSPECIFIED.,.F.,.F.,(4,3,3,3,3,3,4),(43.7031624395564,
44.3223587209537,44.6334770539754,44.944595386997,45.5668320530402,46.1890687190835,
46.5001870521051),.UNSPECIFIED.);
#417=B_SPLINE_CURVE_WITH_KNOTS('',3,(#55548,#55549,#55550,#55551,#55552,
#55553,#55554,#55555,#55556,#55557,#55558,#55559,#55560,#55561,#55562,#55563),
 .UNSPECIFIED.,.F.,.F.,(4,3,3,3,3,4),(0.,0.000528350741057718,0.0356313944030074,
0.05930235574727,0.0966015584375564,0.117357984280487),.UNSPECIFIED.);
#418=B_SPLINE_CURVE_WITH_KNOTS('',3,(#55564,#55565,#55566,#55567,#55568,
#55569,#55570,#55571,#55572),.UNSPECIFIED.,.F.,.F.,(4,1,1,1,1,1,4),(52.0050602882015,
52.6272969542447,52.9384152872664,53.249533620288,53.8717702863312,54.4940069523745,
54.7879760688686),.UNSPECIFIED.);
#419=B_SPLINE_CURVE_WITH_KNOTS('',3,(#55611,#55612,#55613,#55614,#55615,
#55616,#55617,#55618,#55619,#55620,#55621,#55622,#55623,#55624,#55625,#55626),
 .UNSPECIFIED.,.F.,.F.,(4,3,3,3,3,4),(0.,0.000603782874981952,0.0414065099753013,
0.0599624018758385,0.103177307014501,0.119350753234639),.UNSPECIFIED.);
#420=B_SPLINE_CURVE_WITH_KNOTS('',3,(#55628,#55629,#55630,#55631,#55632,
#55633,#55634,#55635,#55636),.UNSPECIFIED.,.F.,.F.,(4,1,1,1,1,1,4),(55.168486169442,
55.4633418551201,56.0919205048047,56.7204991544894,57.0347884793317,57.349077804174,
57.9383886020288),.UNSPECIFIED.);
#421=B_SPLINE_CURVE_WITH_KNOTS('',3,(#55638,#55639,#55640,#55641,#55642,
#55643,#55644,#55645,#55646,#55647,#55648,#55649,#55650),.UNSPECIFIED.,
 .F.,.F.,(4,3,3,3,4),(0.,0.0383618973007027,0.0643956823821936,0.106213551033925,
0.126965609850118),.UNSPECIFIED.);
#422=B_SPLINE_CURVE_WITH_KNOTS('',3,(#55651,#55652,#55653,#55654,#55655,
#55656,#55657,#55658,#55659,#55660,#55661,#55662,#55663,#55664,#55665,#55666,
#55667,#55668,#55669),.UNSPECIFIED.,.F.,.F.,(4,3,3,3,3,3,4),(46.8441142969868,
47.1584036218291,47.7869822715137,48.4155609211983,48.7298502460407,49.044139570883,
49.6727182205676),.UNSPECIFIED.);
#423=B_SPLINE_CURVE_WITH_KNOTS('',3,(#55860,#55861,#55862,#55863,#55864,
#55865,#55866,#55867,#55868,#55869,#55870,#55871,#55872,#55873,#55874,#55875,
#55876,#55877,#55878,#55879,#55880,#55881,#55882,#55883,#55884,#55885,#55886,
#55887,#55888,#55889,#55890,#55891,#55892,#55893,#55894,#55895,#55896,#55897,
#55898,#55899,#55900,#55901,#55902,#55903,#55904,#55905),.UNSPECIFIED.,
 .F.,.F.,(4,3,3,3,3,3,3,3,3,3,3,3,3,3,3,4),(0.,0.00275985982602131,0.0774481870978171,
0.109906700355626,0.163137701127091,0.167106859837268,0.168197417788825,
0.168838059519517,0.169391172034677,0.170064784150426,0.171335649507718,
0.178574548452424,0.187829969840206,0.233407249547609,0.305452969896819,
0.338436364727379),.UNSPECIFIED.);
#424=B_SPLINE_CURVE_WITH_KNOTS('',3,(#55907,#55908,#55909,#55910,#55911,
#55912,#55913,#55914,#55915,#55916,#55917,#55918,#55919,#55920,#55921,#55922,
#55923,#55924,#55925,#55926,#55927,#55928,#55929,#55930,#55931,#55932,#55933,
#55934,#55935,#55936,#55937,#55938,#55939,#55940,#55941,#55942,#55943,#55944,
#55945,#55946),.UNSPECIFIED.,.F.,.F.,(4,3,3,3,3,3,3,3,3,3,3,3,3,4),(-74.551458153763,
-74.0564455670154,-73.5614329802678,-73.0664203935202,-72.5714078067726,
-72.076395220025,-71.5813826332774,-71.0863700465298,-70.5913574597822,
-70.0963448730346,-69.601332286287,-69.1063196995394,-68.6113071127918,
-68.5901919358345),.UNSPECIFIED.);
#425=B_SPLINE_CURVE_WITH_KNOTS('',3,(#55947,#55948,#55949,#55950,#55951,
#55952,#55953,#55954,#55955,#55956,#55957,#55958,#55959,#55960,#55961,#55962,
#55963,#55964,#55965,#55966,#55967,#55968,#55969,#55970,#55971,#55972,#55973,
#55974,#55975,#55976,#55977,#55978,#55979,#55980,#55981,#55982,#55983,#55984,
#55985,#55986,#55987,#55988,#55989,#55990,#55991,#55992,#55993,#55994,#55995,
#55996,#55997,#55998,#55999,#56000,#56001,#56002,#56003,#56004,#56005,#56006,
#56007,#56008,#56009,#56010,#56011,#56012,#56013,#56014,#56015,#56016,#56017,
#56018,#56019,#56020,#56021,#56022,#56023,#56024,#56025,#56026,#56027,#56028,
#56029,#56030,#56031,#56032,#56033,#56034,#56035,#56036,#56037,#56038,#56039,
#56040,#56041,#56042,#56043,#56044,#56045,#56046,#56047,#56048,#56049,#56050,
#56051,#56052,#56053,#56054,#56055,#56056,#56057,#56058,#56059,#56060,#56061,
#56062,#56063,#56064,#56065,#56066,#56067,#56068,#56069,#56070),
 .UNSPECIFIED.,.F.,.F.,(4,3,3,3,3,3,3,3,3,3,3,3,3,3,3,3,3,3,3,3,3,3,3,3,
3,3,3,3,3,3,3,3,3,3,3,3,3,3,3,3,3,4),(-2.47011828786777,-2.41024950183313,
-2.32691774162747,-2.2429717964809,-2.20769641248666,-2.19373056076968,
-2.18265358177193,-2.09840120325056,-2.0136380142207,-1.92915370148376,
-1.91349624184333,-1.90340003136624,-1.82664733476972,-1.74228691319791,
-1.65704413290003,-1.57140550422496,-1.48598895300347,-1.45395774629541,
-1.44439537040528,-1.43517678553118,-1.34896088996718,-1.2622812294094,
-1.22973929933899,-1.1434685919942,-1.05685735056476,-1.00234107811919,
-0.97705394199646,-0.963473476685488,-0.876380514947321,-0.788767505252353,
-0.701239870826566,-0.620727171000232,-0.543136274625203,-0.509190257461128,
-0.49537754808107,-0.482348253819253,-0.395240424237199,-0.307110366650991,
-0.21836748424028,-0.129858392843112,-0.0424592967429643,0.),
 .UNSPECIFIED.);
#426=B_SPLINE_CURVE_WITH_KNOTS('',3,(#56072,#56073,#56074,#56075,#56076,
#56077,#56078),.UNSPECIFIED.,.F.,.F.,(4,1,1,1,4),(64.4256593907634,64.920671977511,
65.4156845642586,65.9106971510062,65.9734457253856),.UNSPECIFIED.);
#427=B_SPLINE_CURVE_WITH_KNOTS('',3,(#56080,#56081,#56082,#56083,#56084,
#56085,#56086,#56087,#56088,#56089),.UNSPECIFIED.,.F.,.F.,(4,2,2,2,4),(0.,
0.000413391377648547,0.0678668660539045,0.107676089687835,0.167694447832979),
 .UNSPECIFIED.);
#428=B_SPLINE_CURVE_WITH_KNOTS('',3,(#56091,#56092,#56093,#56094,#56095,
#56096,#56097,#56098,#56099,#56100,#56101,#56102,#56103,#56104,#56105,#56106,
#56107,#56108,#56109,#56110,#56111,#56112),.UNSPECIFIED.,.F.,.F.,(4,3,3,
3,3,3,3,4),(-55.7551526750958,-55.7409798573541,-55.2459672706065,-54.7509546838589,
-54.2559420971113,-53.7609295103637,-53.2659169236161,-52.8657784087353),
 .UNSPECIFIED.);
#429=B_SPLINE_CURVE_WITH_KNOTS('',3,(#56114,#56115,#56116,#56117,#56118,
#56119,#56120,#56121,#56122,#56123,#56124,#56125,#56126,#56127,#56128,#56129,
#56130,#56131,#56132,#56133,#56134,#56135,#56136,#56137,#56138,#56139,#56140,
#56141,#56142,#56143,#56144,#56145,#56146,#56147,#56148,#56149,#56150,#56151,
#56152,#56153,#56154,#56155,#56156,#56157,#56158,#56159),.UNSPECIFIED.,
 .F.,.F.,(4,3,3,3,3,3,3,3,3,3,3,3,3,3,3,4),(0.,0.00275985982145796,0.0769740122567431,
0.109906700085914,0.163137700726612,0.167106859425189,0.168197417377174,
0.168838059113662,0.16939117163383,0.170064783759705,0.171335649155779,
0.178574548370381,0.187829970155368,0.233407251759405,0.305760949417455,
0.338436370550636),.UNSPECIFIED.);
#430=B_SPLINE_CURVE_WITH_KNOTS('',3,(#56161,#56162,#56163,#56164,#56165,
#56166,#56167,#56168,#56169,#56170,#56171,#56172,#56173,#56174,#56175,#56176,
#56177,#56178,#56179,#56180,#56181,#56182,#56183,#56184,#56185,#56186,#56187,
#56188,#56189,#56190,#56191,#56192,#56193,#56194,#56195,#56196,#56197,#56198,
#56199,#56200),.UNSPECIFIED.,.F.,.F.,(4,3,3,3,3,3,3,3,3,3,3,3,3,4),(-62.0383379822753,
-61.6811308983253,-61.1861183115777,-60.6911057248301,-60.1960931380825,
-59.7010805513349,-59.2060679645873,-58.7110553778397,-58.2160427910921,
-57.7210302043445,-57.2260176175969,-56.7310050308493,-56.2359924441017,
-56.0238213214754),.UNSPECIFIED.);
#431=B_SPLINE_CURVE_WITH_KNOTS('',3,(#56202,#56203,#56204,#56205,#56206,
#56207,#56208,#56209,#56210,#56211,#56212,#56213,#56214,#56215,#56216,#56217,
#56218,#56219,#56220,#56221,#56222,#56223,#56224,#56225,#56226,#56227,#56228,
#56229,#56230,#56231,#56232,#56233,#56234,#56235,#56236,#56237,#56238,#56239,
#56240,#56241,#56242,#56243,#56244,#56245,#56246,#56247,#56248,#56249,#56250),
 .UNSPECIFIED.,.F.,.F.,(4,3,3,3,3,3,3,3,3,3,3,3,3,3,3,3,4),(0.,0.00275985982151005,
0.0762872625369273,0.109906700097837,0.163137700732282,0.164734489152777,
0.167106859431402,0.168197417392199,0.168838059132773,0.169391171638563,
0.170064783750812,0.17133564913502,0.178574548241108,0.187829969458916,
0.233407248703376,0.304919373849625,0.338436367941764),.UNSPECIFIED.);
#432=B_SPLINE_CURVE_WITH_KNOTS('',3,(#56251,#56252,#56253,#56254,#56255,
#56256,#56257,#56258,#56259,#56260,#56261,#56262,#56263,#56264,#56265,#56266,
#56267,#56268,#56269,#56270,#56271,#56272,#56273,#56274,#56275,#56276,#56277,
#56278,#56279,#56280,#56281,#56282,#56283,#56284,#56285,#56286,#56287,#56288,
#56289,#56290),.UNSPECIFIED.,.F.,.F.,(4,3,3,3,3,3,3,3,3,3,3,3,3,4),(-68.321523289455,
-68.1162945260442,-67.6212819392966,-67.126269352549,-66.6312567658014,
-66.1362441790538,-65.6412315923062,-65.1462190055586,-64.651206418811,
-64.1561938320634,-63.6611812453157,-63.1661686585681,-62.6711560718205,
-62.3070066286549),.UNSPECIFIED.);
#433=B_SPLINE_CURVE_WITH_KNOTS('',3,(#56329,#56330,#56331,#56332,#56333,
#56334,#56335,#56336,#56337,#56338,#56339,#56340,#56341,#56342,#56343,#56344),
 .UNSPECIFIED.,.F.,.F.,(4,3,3,3,3,4),(0.,0.000524175925068961,0.0370091730147864,
0.0592526903266393,0.094159836272508,0.118128821372448),.UNSPECIFIED.);
#434=B_SPLINE_CURVE_WITH_KNOTS('',3,(#56346,#56347,#56348,#56349,#56350,
#56351,#56352,#56353,#56354,#56355,#56356,#56357,#56358,#56359,#56360,#56361,
#56362,#56363,#56364),.UNSPECIFIED.,.F.,.F.,(4,3,3,3,3,3,4),(-52.6241835979417,
-52.387037036532,-51.730035730462,-51.073034424392,-50.744533771357,-50.087532465287,
-49.7715547347365),.UNSPECIFIED.);
#435=B_SPLINE_CURVE_WITH_KNOTS('',3,(#56366,#56367,#56368,#56369,#56370,
#56371,#56372,#56373),.UNSPECIFIED.,.F.,.F.,(4,2,2,4),(0.,0.0343081782947535,
0.0828883632862996,0.165726765447382),.UNSPECIFIED.);
#436=B_SPLINE_CURVE_WITH_KNOTS('',3,(#56374,#56375,#56376,#56377,#56378,
#56379,#56380,#56381,#56382),.UNSPECIFIED.,.F.,.F.,(4,1,1,1,1,1,4),(61.413786866147,
61.742287519182,62.399288825252,62.727789478287,63.384790784357,64.041792090427,
64.370292743462),.UNSPECIFIED.);
#437=B_SPLINE_CURVE_WITH_KNOTS('',3,(#56421,#56422,#56423,#56424,#56425,
#56426,#56427,#56428,#56429,#56430,#56431,#56432,#56433,#56434,#56435,#56436),
 .UNSPECIFIED.,.F.,.F.,(4,3,3,3,3,4),(0.,0.000559897176802773,0.042322412952373,
0.0600025715731581,0.0991684809679751,0.118377563451883),.UNSPECIFIED.);
#438=B_SPLINE_CURVE_WITH_KNOTS('',3,(#56438,#56439,#56440,#56441,#56442,
#56443,#56444,#56445,#56446,#56447,#56448,#56449,#56450,#56451,#56452,#56453,
#56454,#56455,#56456),.UNSPECIFIED.,.F.,.F.,(4,3,3,3,3,3,4),(-49.4385230424123,
-49.1359708046958,-48.5118455167721,-47.8877202288484,-47.5756575848866,
-47.2635949409247,-46.639469653001),.UNSPECIFIED.);
#439=B_SPLINE_CURVE_WITH_KNOTS('',3,(#56458,#56459,#56460,#56461,#56462,
#56463,#56464,#56465,#56466,#56467,#56468,#56469,#56470),.UNSPECIFIED.,
 .F.,.F.,(4,3,3,3,4),(0.,0.0344844180980609,0.0592774715655555,0.0955221408315289,
0.117941444539697),.UNSPECIFIED.);
#440=B_SPLINE_CURVE_WITH_KNOTS('',3,(#56471,#56472,#56473,#56474,#56475,
#56476,#56477,#56478,#56479),.UNSPECIFIED.,.F.,.F.,(4,1,1,1,1,1,4),(58.3068143978534,
58.9183499948197,59.2304126387815,59.5424752827434,60.166600570667,60.7907258585907,
61.1027885025526),.UNSPECIFIED.);
#441=B_SPLINE_CURVE_WITH_KNOTS('',3,(#56822,#56823,#56824,#56825,#56826,
#56827,#56828,#56829,#56830,#56831,#56832,#56833,#56834,#56835,#56836,#56837,
#56838,#56839,#56840,#56841,#56842,#56843,#56844,#56845,#56846,#56847,#56848,
#56849,#56850,#56851,#56852,#56853,#56854,#56855,#56856,#56857,#56858,#56859,
#56860,#56861,#56862,#56863,#56864,#56865,#56866,#56867),.UNSPECIFIED.,
 .F.,.F.,(4,3,3,3,3,3,3,3,3,3,3,3,3,3,3,4),(0.,0.00275985983228642,0.077257938139478,
0.109906700732534,0.163137701680564,0.167106860403426,0.168197418365421,
0.168838060104028,0.169391172613466,0.170064784717482,0.171335650058926,
0.178574549011496,0.187829969760767,0.233407246964211,0.305648570218663,
0.338436365203866),.UNSPECIFIED.);
#442=B_SPLINE_CURVE_WITH_KNOTS('',3,(#56869,#56870,#56871,#56872,#56873,
#56874,#56875,#56876,#56877,#56878,#56879,#56880,#56881,#56882,#56883,#56884,
#56885,#56886,#56887,#56888,#56889,#56890,#56891,#56892,#56893,#56894,#56895,
#56896,#56897,#56898,#56899,#56900,#56901,#56902,#56903,#56904,#56905,#56906,
#56907,#56908,#56909,#56910,#56911),.UNSPECIFIED.,.F.,.F.,(4,3,3,3,3,3,
3,3,3,3,3,3,3,3,4),(-11.7728555248387,-11.7422679037385,-11.2530067410827,
-10.7637455784269,-10.2744844157712,-9.78522325311539,-9.29596209045961,
-8.80670092780385,-8.31743976514808,-7.82817860249231,-7.33891743983654,
-6.84965627718077,-6.360395114525,-5.87113395186923,-5.75833886403865),
 .UNSPECIFIED.);
#443=B_SPLINE_CURVE_WITH_KNOTS('',3,(#56913,#56914,#56915,#56916,#56917,
#56918,#56919,#56920,#56921,#56922,#56923,#56924,#56925,#56926,#56927,#56928,
#56929,#56930,#56931,#56932,#56933,#56934,#56935,#56936,#56937,#56938,#56939,
#56940,#56941,#56942,#56943,#56944,#56945,#56946,#56947,#56948,#56949,#56950,
#56951,#56952,#56953,#56954,#56955,#56956,#56957,#56958),.UNSPECIFIED.,
 .F.,.F.,(4,3,3,3,3,3,3,3,3,3,3,3,3,3,3,4),(0.,0.00275985982376174,0.0770370771830512,
0.109906700228133,0.163137700929448,0.167106859635108,0.168197417591288,
0.168838059324371,0.169391171829,0.170064783926107,0.171335649248441,0.178574548066871,
0.187829968616436,0.233407244865315,0.30574397986754,0.338436361285487),
 .UNSPECIFIED.);
#444=B_SPLINE_CURVE_WITH_KNOTS('',3,(#56960,#56961,#56962,#56963,#56964,
#56965,#56966,#56967,#56968,#56969,#56970,#56971,#56972,#56973,#56974,#56975,
#56976,#56977,#56978,#56979,#56980,#56981,#56982,#56983,#56984,#56985,#56986,
#56987,#56988,#56989,#56990,#56991,#56992,#56993,#56994,#56995,#56996,#56997,
#56998,#56999),.UNSPECIFIED.,.F.,.F.,(4,3,3,3,3,3,3,3,3,3,3,3,3,4),(-18.0560408320183,
-17.6134018556077,-17.1241406929519,-16.6348795302962,-16.1456183676404,
-15.6563572049846,-15.1670960423288,-14.6778348796731,-14.1885737170173,
-13.6993125543615,-13.2100513917058,-12.72079022905,-12.2315290663942,-12.0415241712181),
 .UNSPECIFIED.);
#445=B_SPLINE_CURVE_WITH_KNOTS('',3,(#57001,#57002,#57003,#57004,#57005,
#57006,#57007,#57008,#57009,#57010,#57011,#57012,#57013,#57014,#57015,#57016,
#57017,#57018,#57019,#57020,#57021,#57022,#57023,#57024,#57025,#57026,#57027,
#57028,#57029,#57030,#57031,#57032,#57033,#57034,#57035,#57036,#57037,#57038,
#57039,#57040,#57041,#57042,#57043,#57044,#57045,#57046),.UNSPECIFIED.,
 .F.,.F.,(4,3,3,3,3,3,3,3,3,3,3,3,3,3,3,4),(0.,0.00275985983113353,0.0767461432217819,
0.10990670066103,0.163137701579206,0.167106860299809,0.168197418254294,
0.168838059995389,0.169391172533029,0.17006478467472,0.171335650088616,
0.178574549335223,0.187829970571773,0.233407250081592,0.279164911505272,
0.338436372145432),.UNSPECIFIED.);
#446=B_SPLINE_CURVE_WITH_KNOTS('',3,(#57048,#57049,#57050,#57051,#57052,
#57053,#57054,#57055,#57056,#57057,#57058,#57059,#57060,#57061,#57062,#57063,
#57064,#57065,#57066,#57067,#57068,#57069,#57070,#57071,#57072,#57073,#57074,
#57075,#57076,#57077,#57078,#57079,#57080,#57081,#57082,#57083,#57084,#57085,
#57086,#57087),.UNSPECIFIED.,.F.,.F.,(4,3,3,3,3,3,3,3,3,3,3,3,3,4),(-24.3392261391979,
-23.9737969701327,-23.4845358074769,-22.9952746448212,-22.5060134821654,
-22.0167523195096,-21.5274911568539,-21.0382299941981,-20.5489688315423,
-20.0597076688865,-19.5704465062308,-19.081185343575,-18.5919241809192,
-18.3247094783978),.UNSPECIFIED.);
#447=B_SPLINE_CURVE_WITH_KNOTS('',3,(#57089,#57090,#57091,#57092,#57093,
#57094,#57095,#57096,#57097,#57098,#57099,#57100,#57101,#57102,#57103,#57104,
#57105,#57106,#57107,#57108,#57109,#57110,#57111,#57112,#57113,#57114,#57115,
#57116,#57117,#57118,#57119,#57120,#57121,#57122,#57123,#57124,#57125,#57126,
#57127,#57128,#57129,#57130,#57131,#57132,#57133,#57134,#57135,#57136,#57137),
 .UNSPECIFIED.,.F.,.F.,(4,3,3,3,3,3,3,3,3,3,3,3,3,3,3,3,4),(0.,0.00275985982375089,
0.0763759506442948,0.109906700228139,0.163137700928605,0.167106859632871,
0.168197417593916,0.168838059333146,0.169391171837645,0.170064783944139,
0.171335649305587,0.17857454832124,0.182207199497083,0.18782996934018,0.233407247686735,
0.304865724045757,0.338436365949266),.UNSPECIFIED.);
#448=B_SPLINE_CURVE_WITH_KNOTS('',3,(#57139,#57140,#57141,#57142,#57143,
#57144,#57145,#57146,#57147,#57148,#57149,#57150,#57151,#57152,#57153,#57154,
#57155,#57156,#57157,#57158,#57159,#57160,#57161,#57162,#57163,#57164,#57165,
#57166,#57167,#57168,#57169,#57170,#57171,#57172,#57173,#57174,#57175,#57176,
#57177,#57178),.UNSPECIFIED.,.F.,.F.,(4,3,3,3,3,3,3,3,3,3,3,3,3,4),(-30.6224114463774,
-30.3341920846577,-29.8449309220019,-29.3556697593462,-28.8664085966904,
-28.3771474340346,-27.8878862713788,-27.3986251087231,-26.9093639460673,
-26.4201027834115,-25.9308416207558,-25.4415804581,-24.9523192954442,-24.6078947855774),
 .UNSPECIFIED.);
#449=B_SPLINE_CURVE_WITH_KNOTS('',3,(#57180,#57181,#57182,#57183,#57184,
#57185,#57186,#57187,#57188,#57189,#57190,#57191,#57192,#57193,#57194,#57195,
#57196,#57197,#57198,#57199,#57200,#57201,#57202,#57203,#57204,#57205,#57206,
#57207,#57208,#57209,#57210,#57211,#57212,#57213,#57214,#57215,#57216,#57217,
#57218,#57219,#57220,#57221,#57222,#57223,#57224,#57225,#57226,#57227,#57228),
 .UNSPECIFIED.,.F.,.F.,(4,3,3,3,3,3,3,3,3,3,3,3,3,3,3,3,4),(0.,0.00275985982375613,
0.0756134546611658,0.0855438259912015,0.10990670022032,0.163137700928118,
0.167106859633686,0.168197417590077,0.168838059326623,0.169391171839922,
0.170064783940488,0.171335649227684,0.178574547859423,0.187829968945836,
0.233407247069485,0.305184663799026,0.338436357196743),.UNSPECIFIED.);
#450=B_SPLINE_CURVE_WITH_KNOTS('',3,(#57230,#57231,#57232,#57233,#57234,
#57235,#57236,#57237,#57238,#57239,#57240,#57241,#57242,#57243,#57244,#57245,
#57246,#57247,#57248,#57249,#57250,#57251,#57252,#57253,#57254,#57255,#57256,
#57257,#57258,#57259,#57260,#57261,#57262,#57263,#57264,#57265,#57266,#57267,
#57268,#57269),.UNSPECIFIED.,.F.,.F.,(4,3,3,3,3,3,3,3,3,3,3,3,3,4),(-36.905596753557,
-36.6945871991827,-36.2053260365269,-35.7160648738711,-35.2268037112154,
-34.7375425485596,-34.2482813859039,-33.7590202232481,-33.2697590605923,
-32.7804978979365,-32.2912367352808,-31.801975572625,-31.3127144099692,
-30.8910800927569),.UNSPECIFIED.);
#451=B_SPLINE_CURVE_WITH_KNOTS('',3,(#57271,#57272,#57273,#57274,#57275,
#57276,#57277,#57278,#57279,#57280,#57281,#57282,#57283,#57284,#57285,#57286,
#57287,#57288,#57289,#57290,#57291,#57292,#57293,#57294,#57295,#57296,#57297,
#57298,#57299,#57300,#57301,#57302,#57303,#57304,#57305,#57306,#57307,#57308,
#57309,#57310,#57311,#57312,#57313,#57314,#57315,#57316),.UNSPECIFIED.,
 .F.,.F.,(4,3,3,3,3,3,3,3,3,3,3,3,3,3,3,4),(0.,0.00275985982374703,0.0774602223847068,
0.109906700228556,0.163137700928317,0.167106859634754,0.168197417583678,
0.168838059317443,0.169391171848623,0.170064783974852,0.171335649325392,
0.178574548289135,0.187829969380545,0.233407247950148,0.305428214865697,
0.338436364853883),.UNSPECIFIED.);
#452=B_SPLINE_CURVE_WITH_KNOTS('',3,(#57318,#57319,#57320,#57321,#57322,
#57323,#57324,#57325,#57326,#57327,#57328,#57329,#57330,#57331,#57332,#57333,
#57334,#57335,#57336,#57337,#57338,#57339),.UNSPECIFIED.,.F.,.F.,(4,3,3,
3,3,3,3,4),(-40.1194153377731,-39.6301541751173,-39.1408930124615,-38.6516318498058,
-38.16237068715,-37.6731095244942,-37.1838483618385,-37.1742653999366),
 .UNSPECIFIED.);
#453=B_SPLINE_CURVE_WITH_KNOTS('',3,(#57340,#57341,#57342,#57343,#57344,
#57345,#57346,#57347,#57348,#57349,#57350,#57351,#57352,#57353,#57354,#57355,
#57356,#57357,#57358,#57359,#57360,#57361),.UNSPECIFIED.,.F.,.F.,(4,3,3,
3,3,3,3,4),(0.,0.0298454239823248,0.0587107917683048,0.0694364850727102,
0.0931059490162252,0.116200547796362,0.13859691269707,0.149774774907473),
 .UNSPECIFIED.);
#454=B_SPLINE_CURVE_WITH_KNOTS('',3,(#57363,#57364,#57365,#57366,#57367,
#57368,#57369,#57370,#57371,#57372,#57373,#57374),.UNSPECIFIED.,.F.,.F.,
(4,1,1,1,1,1,1,1,1,4),(11.654755053895,12.1440162165507,12.6332773792065,
13.1225385418623,13.611799704518,14.1010608671738,14.5903220298296,15.0795831924853,
15.5688443551411,15.707963267949),.UNSPECIFIED.);
#455=B_SPLINE_CURVE_WITH_KNOTS('',3,(#57376,#57377,#57378,#57379,#57380,
#57381,#57382,#57383,#57384,#57385,#57386,#57387,#57388,#57389,#57390,#57391,
#57392,#57393,#57394,#57395,#57396,#57397,#57398,#57399,#57400,#57401,#57402,
#57403,#57404,#57405,#57406,#57407,#57408,#57409,#57410,#57411,#57412,#57413,
#57414,#57415,#57416,#57417,#57418,#57419,#57420,#57421,#57422,#57423,#57424,
#57425,#57426,#57427,#57428,#57429,#57430,#57431,#57432,#57433,#57434,#57435,
#57436,#57437,#57438,#57439,#57440,#57441,#57442,#57443,#57444,#57445,#57446,
#57447,#57448,#57449,#57450,#57451,#57452,#57453,#57454,#57455,#57456,#57457,
#57458,#57459,#57460,#57461,#57462,#57463,#57464,#57465,#57466,#57467,#57468,
#57469,#57470,#57471,#57472,#57473,#57474,#57475,#57476,#57477,#57478,#57479,
#57480,#57481,#57482,#57483,#57484,#57485,#57486,#57487,#57488,#57489,#57490,
#57491,#57492,#57493,#57494,#57495,#57496,#57497,#57498,#57499,#57500,#57501,
#57502),.UNSPECIFIED.,.F.,.F.,(4,3,3,3,3,3,3,3,3,3,3,3,3,3,3,3,3,3,3,3,
3,3,3,3,3,3,3,3,3,3,3,3,3,3,3,3,3,3,3,3,3,3,4),(-2.4657711816956,-2.37742988198504,
-2.37203686248739,-2.2834262203604,-2.21828108582746,-2.18798524934555,
-2.16783026643965,-2.15520023029036,-2.06721376735589,-1.9794908344413,
-1.8924658234541,-1.87064293008793,-1.86055558238173,-1.77341354772103,
-1.76226514409688,-1.67528516349454,-1.58795101178645,-1.50086017635826,
-1.4164004091096,-1.3970664196555,-1.385204327045,-1.29903625463541,-1.21307140372724,
-1.16302110736361,-1.07672492900881,-0.990705158543006,-0.938804325301365,
-0.925019860062695,-0.913972265813138,-0.828818892685938,-0.743601294890201,
-0.659189663034413,-0.575498492609885,-0.503561181033649,-0.472088607219046,
-0.460708940919763,-0.450070986721853,-0.366465695615636,-0.282278701507383,
-0.198277355611721,-0.114917112729238,-0.0330178077316585,0.),
 .UNSPECIFIED.);
#456=B_SPLINE_CURVE_WITH_KNOTS('',3,(#57503,#57504,#57505,#57506,#57507,
#57508,#57509,#57510,#57511,#57512,#57513,#57514,#57515,#57516,#57517,#57518,
#57519,#57520,#57521,#57522,#57523,#57524,#57525,#57526,#57527),
 .UNSPECIFIED.,.F.,.F.,(4,3,3,3,3,3,3,3,4),(-5.48967021765908,-5.38187278921346,
-4.89261162655769,-4.40335046390192,-3.91408930124615,-3.42482813859038,
-2.93556697593462,-2.44630581327885,-2.03145528794232),.UNSPECIFIED.);
#457=B_SPLINE_CURVE_WITH_KNOTS('',3,(#57566,#57567,#57568,#57569,#57570,
#57571,#57572,#57573,#57574,#57575,#57576,#57577,#57578),.UNSPECIFIED.,
 .F.,.F.,(4,3,3,3,4),(0.,0.0431803782595757,0.0615400944013658,0.102677518916927,
0.124427909767835),.UNSPECIFIED.);
#458=B_SPLINE_CURVE_WITH_KNOTS('',3,(#57580,#57581,#57582,#57583,#57584,
#57585,#57586,#57587,#57588),.UNSPECIFIED.,.F.,.F.,(4,1,1,1,1,1,4),(51.9824652652652,
52.230691972308,52.8804712757956,53.2053609275394,53.855140231027,54.1800298827708,
54.7942738648993),.UNSPECIFIED.);
#459=B_SPLINE_CURVE_WITH_KNOTS('',3,(#57590,#57591,#57592,#57593,#57594,
#57595,#57596,#57597,#57598,#57599,#57600,#57601,#57602,#57603,#57604,#57605,
#57606,#57607,#57608,#57609,#57610,#57611),.UNSPECIFIED.,.F.,.F.,(4,3,3,
3,3,3,3,4),(0.,0.000338425381540912,0.0224866539540187,0.045452247155042,
0.0654166068739022,0.0935951529420607,0.122883934914188,0.150189106809355),
 .UNSPECIFIED.);
#460=B_SPLINE_CURVE_WITH_KNOTS('',3,(#57612,#57613,#57614,#57615,#57616,
#57617,#57618,#57619,#57620,#57621,#57622,#57623,#57624,#57625,#57626,#57627,
#57628,#57629,#57630),.UNSPECIFIED.,.F.,.F.,(4,3,3,3,3,3,4),(-43.1750541323635,
-42.5252748288759,-42.2003851771321,-41.5506058736444,-41.2257162219006,
-40.575936918413,-40.2510472666692),.UNSPECIFIED.);
#461=B_SPLINE_CURVE_WITH_KNOTS('',3,(#57632,#57633,#57634,#57635,#57636,
#57637),.UNSPECIFIED.,.F.,.F.,(4,2,4),(0.134768241793669,0.16617963596043,
0.185292243031058),.UNSPECIFIED.);
#462=B_SPLINE_CURVE_WITH_KNOTS('',3,(#57638,#57639,#57640,#57641,#57642,
#57643),.UNSPECIFIED.,.F.,.F.,(4,2,4),(0.970784459515729,0.997055295420078,
1.03386954271643),.UNSPECIFIED.);
#463=B_SPLINE_CURVE_WITH_KNOTS('',3,(#57647,#57648,#57649,#57650),
 .UNSPECIFIED.,.F.,.F.,(4,4),(0.705578480917695,0.742911382707452),
 .UNSPECIFIED.);
#464=B_SPLINE_CURVE_WITH_KNOTS('',3,(#57651,#57652,#57653,#57654,#57655,
#57656),.UNSPECIFIED.,.F.,.F.,(4,2,4),(0.490224693667975,0.498523894319622,
0.54050457124268),.UNSPECIFIED.);
#465=B_SPLINE_CURVE_WITH_KNOTS('',3,(#57658,#57659,#57660,#57661),
 .UNSPECIFIED.,.F.,.F.,(4,4),(0.686256720735745,0.723216288120665),
 .UNSPECIFIED.);
#466=B_SPLINE_CURVE_WITH_KNOTS('',3,(#57662,#57663,#57664,#57665),
 .UNSPECIFIED.,.F.,.F.,(4,4),(0.518163743605581,0.562900565143627),
 .UNSPECIFIED.);
#467=B_SPLINE_CURVE_WITH_KNOTS('',3,(#57668,#57669,#57670,#57671),
 .UNSPECIFIED.,.F.,.F.,(4,4),(1.28135134421279,1.31862990715387),
 .UNSPECIFIED.);
#468=B_SPLINE_CURVE_WITH_KNOTS('',3,(#57673,#57674,#57675,#57676,#57677,
#57678,#57679,#57680,#57681),.UNSPECIFIED.,.F.,.F.,(4,1,1,1,1,1,4),(55.1638586060211,
55.4429246232081,56.0685764469255,56.3814023587843,57.0070541825018,57.3198800943605,
57.9305195965772),.UNSPECIFIED.);
#469=B_SPLINE_CURVE_WITH_KNOTS('',3,(#57682,#57683,#57684,#57685),
 .UNSPECIFIED.,.F.,.F.,(4,4),(1.26160163394232,1.29910180138512),
 .UNSPECIFIED.);
#470=B_SPLINE_CURVE_WITH_KNOTS('',3,(#57735,#57736,#57737,#57738,#57739,
#57740,#57741,#57742,#57743,#57744,#57745,#57746,#57747,#57748,#57749,#57750),
 .UNSPECIFIED.,.F.,.F.,(4,3,3,3,3,4),(0.,0.000515694897373992,0.0418024345464061,
0.0635027671358636,0.106468605792955,0.124601478701958),.UNSPECIFIED.);
#471=B_SPLINE_CURVE_WITH_KNOTS('',3,(#57752,#57753,#57754,#57755,#57756,
#57757,#57758,#57759,#57760,#57761,#57762,#57763,#57764,#57765,#57766,#57767,
#57768,#57769,#57770),.UNSPECIFIED.,.F.,.F.,(4,3,3,3,3,3,4),(-46.290776864183,
-45.6651250404655,-45.3522991286068,-44.7266473048893,-44.4138213930306,
-43.7881695693131,-43.4753436574544),.UNSPECIFIED.);
#472=B_SPLINE_CURVE_WITH_KNOTS('',3,(#57771,#57772,#57773,#57774,#57775,
#57776,#57777,#57778,#57779,#57780,#57781,#57782,#57783),.UNSPECIFIED.,
 .F.,.F.,(4,3,3,3,4),(0.,0.0393665545192843,0.0589812601558904,0.101040205845147,
0.118470175365851),.UNSPECIFIED.);
#473=B_SPLINE_CURVE_WITH_KNOTS('',3,(#57826,#57827,#57828,#57829,#57830,
#57831),.UNSPECIFIED.,.F.,.F.,(4,2,4),(0.805938743676149,0.830541752976356,
0.840481356535727),.UNSPECIFIED.);
#474=B_SPLINE_CURVE_WITH_KNOTS('',3,(#57838,#57839,#57840,#57841),
 .UNSPECIFIED.,.F.,.F.,(4,4),(1.16287000320261,1.19712104343039),
 .UNSPECIFIED.);
#475=B_SPLINE_CURVE_WITH_KNOTS('',3,(#57842,#57843,#57844,#57845),
 .UNSPECIFIED.,.F.,.F.,(4,4),(-0.0717727639817645,-0.0462671248394357),
 .UNSPECIFIED.);
#476=B_SPLINE_CURVE_WITH_KNOTS('',3,(#57855,#57856,#57857,#57858,#57859,
#57860),.UNSPECIFIED.,.F.,.F.,(4,2,4),(0.332215634323022,0.415268209319378,
0.418708545872871),.UNSPECIFIED.);
#477=B_SPLINE_CURVE_WITH_KNOTS('',3,(#57861,#57862,#57863,#57864),
 .UNSPECIFIED.,.F.,.F.,(4,4),(0.255235312149345,0.332215634323022),
 .UNSPECIFIED.);
#478=B_SPLINE_CURVE_WITH_KNOTS('',3,(#57865,#57866,#57867,#57868),
 .UNSPECIFIED.,.F.,.F.,(4,4),(0.517942109132407,0.546042694596367),
 .UNSPECIFIED.);
#479=B_SPLINE_CURVE_WITH_KNOTS('',3,(#57870,#57871,#57872,#57873),
 .UNSPECIFIED.,.F.,.F.,(4,4),(0.701030951378668,0.726642077695294),
 .UNSPECIFIED.);
#480=B_SPLINE_CURVE_WITH_KNOTS('',3,(#57874,#57875,#57876,#57877),
 .UNSPECIFIED.,.F.,.F.,(4,4),(0.621839088202796,0.647297338681728),
 .UNSPECIFIED.);
#481=B_SPLINE_CURVE_WITH_KNOTS('',3,(#57879,#57880,#57881,#57882),
 .UNSPECIFIED.,.F.,.F.,(4,4),(0.0269607932098941,0.052218921738027),
 .UNSPECIFIED.);
#482=B_SPLINE_CURVE_WITH_KNOTS('',3,(#57884,#57885,#57886,#57887),
 .UNSPECIFIED.,.F.,.F.,(4,4),(0.108777077446072,0.139263533037876),
 .UNSPECIFIED.);
#1221=FACE_BOUND('',#6593,.T.);
#1222=FACE_BOUND('',#6631,.T.);
#1223=FACE_BOUND('',#6632,.T.);
#1224=FACE_BOUND('',#6633,.T.);
#1225=FACE_BOUND('',#6634,.T.);
#1226=FACE_BOUND('',#6635,.T.);
#1227=FACE_BOUND('',#6645,.T.);
#1228=FACE_BOUND('',#6646,.T.);
#1229=FACE_BOUND('',#6647,.T.);
#1230=FACE_BOUND('',#6648,.T.);
#1231=FACE_BOUND('',#6649,.T.);
#1232=FACE_BOUND('',#6712,.T.);
#1233=FACE_BOUND('',#6722,.T.);
#2527=PLANE('',#36181);
#2528=PLANE('',#36183);
#2529=PLANE('',#36184);
#2530=PLANE('',#36185);
#2531=PLANE('',#36186);
#2532=PLANE('',#36187);
#2533=PLANE('',#36188);
#2534=PLANE('',#36189);
#2535=PLANE('',#36190);
#2536=PLANE('',#36191);
#2537=PLANE('',#36192);
#2538=PLANE('',#36193);
#2539=PLANE('',#36194);
#2540=PLANE('',#36195);
#2541=PLANE('',#36196);
#2542=PLANE('',#36197);
#2543=PLANE('',#36198);
#2544=PLANE('',#36199);
#2545=PLANE('',#36200);
#2546=PLANE('',#36201);
#2547=PLANE('',#36202);
#2548=PLANE('',#36203);
#2549=PLANE('',#36204);
#2550=PLANE('',#36205);
#2551=PLANE('',#36206);
#2552=PLANE('',#36207);
#2553=PLANE('',#36208);
#2554=PLANE('',#36209);
#2555=PLANE('',#36210);
#2556=PLANE('',#36211);
#2557=PLANE('',#36212);
#2558=PLANE('',#36213);
#2559=PLANE('',#36214);
#2560=PLANE('',#36215);
#2561=PLANE('',#36216);
#2562=PLANE('',#36217);
#2563=PLANE('',#36221);
#2564=PLANE('',#36242);
#2565=PLANE('',#36250);
#2566=PLANE('',#36251);
#2567=PLANE('',#36252);
#2568=PLANE('',#36253);
#2569=PLANE('',#36254);
#2570=PLANE('',#36255);
#2571=PLANE('',#36267);
#2572=PLANE('',#36274);
#2573=PLANE('',#36277);
#2574=PLANE('',#36281);
#2575=PLANE('',#36283);
#2576=PLANE('',#36284);
#2577=PLANE('',#36285);
#2578=PLANE('',#36286);
#2579=PLANE('',#36287);
#2580=PLANE('',#36288);
#2581=PLANE('',#36289);
#2582=PLANE('',#36290);
#2583=PLANE('',#36291);
#2584=PLANE('',#36292);
#2585=PLANE('',#36316);
#2586=PLANE('',#36326);
#2587=PLANE('',#36328);
#2588=PLANE('',#36332);
#2589=PLANE('',#36333);
#2590=PLANE('',#36339);
#3017=CYLINDRICAL_SURFACE('',#36167,11.59764);
#3018=CYLINDRICAL_SURFACE('',#36168,11.59764);
#3019=CYLINDRICAL_SURFACE('',#36169,11.59764);
#3020=CYLINDRICAL_SURFACE('',#36170,11.59764);
#3021=CYLINDRICAL_SURFACE('',#36171,11.59764);
#3022=CYLINDRICAL_SURFACE('',#36172,11.59764);
#3023=CYLINDRICAL_SURFACE('',#36173,11.59764);
#3024=CYLINDRICAL_SURFACE('',#36175,11.59764);
#3025=CYLINDRICAL_SURFACE('',#36176,11.59764);
#3026=CYLINDRICAL_SURFACE('',#36226,6.75);
#3027=CYLINDRICAL_SURFACE('',#36230,6.75);
#3028=CYLINDRICAL_SURFACE('',#36234,6.75);
#3029=CYLINDRICAL_SURFACE('',#36238,6.75);
#3030=CYLINDRICAL_SURFACE('',#36264,25.4);
#3031=CYLINDRICAL_SURFACE('',#36268,11.59764);
#3032=CYLINDRICAL_SURFACE('',#36269,11.59764);
#3033=CYLINDRICAL_SURFACE('',#36271,11.59764);
#3034=CYLINDRICAL_SURFACE('',#36272,11.59764);
#3035=CYLINDRICAL_SURFACE('',#36273,11.59764);
#3036=CYLINDRICAL_SURFACE('',#36294,12.61364);
#3037=CYLINDRICAL_SURFACE('',#36295,12.61364);
#3038=CYLINDRICAL_SURFACE('',#36296,12.61364);
#3039=CYLINDRICAL_SURFACE('',#36297,12.61364);
#3040=CYLINDRICAL_SURFACE('',#36299,12.61364);
#3041=CYLINDRICAL_SURFACE('',#36301,12.61364);
#3042=CYLINDRICAL_SURFACE('',#36302,12.61364);
#3043=CYLINDRICAL_SURFACE('',#36303,12.61364);
#3044=CYLINDRICAL_SURFACE('',#36304,12.61364);
#3045=CYLINDRICAL_SURFACE('',#36305,12.61364);
#3046=CYLINDRICAL_SURFACE('',#36306,12.61364);
#3047=CYLINDRICAL_SURFACE('',#36307,12.61364);
#3048=CYLINDRICAL_SURFACE('',#36309,12.61364);
#3049=CYLINDRICAL_SURFACE('',#36310,12.61364);
#3050=CYLINDRICAL_SURFACE('',#36311,2.20000000000001);
#3051=CYLINDRICAL_SURFACE('',#36314,21.8313);
#3052=CYLINDRICAL_SURFACE('',#36320,17.47);
#3053=CYLINDRICAL_SURFACE('',#36329,13.47);
#3054=CYLINDRICAL_SURFACE('',#36335,11.9);
#3055=CYLINDRICAL_SURFACE('',#36340,12.61364);
#4395=FACE_OUTER_BOUND('',#6581,.T.);
#4396=FACE_OUTER_BOUND('',#6582,.T.);
#4397=FACE_OUTER_BOUND('',#6583,.T.);
#4398=FACE_OUTER_BOUND('',#6584,.T.);
#4399=FACE_OUTER_BOUND('',#6585,.T.);
#4400=FACE_OUTER_BOUND('',#6586,.T.);
#4401=FACE_OUTER_BOUND('',#6587,.T.);
#4402=FACE_OUTER_BOUND('',#6588,.T.);
#4403=FACE_OUTER_BOUND('',#6589,.T.);
#4404=FACE_OUTER_BOUND('',#6590,.T.);
#4405=FACE_OUTER_BOUND('',#6591,.T.);
#4406=FACE_OUTER_BOUND('',#6592,.T.);
#4407=FACE_OUTER_BOUND('',#6594,.T.);
#4408=FACE_OUTER_BOUND('',#6595,.T.);
#4409=FACE_OUTER_BOUND('',#6596,.T.);
#4410=FACE_OUTER_BOUND('',#6597,.T.);
#4411=FACE_OUTER_BOUND('',#6598,.T.);
#4412=FACE_OUTER_BOUND('',#6599,.T.);
#4413=FACE_OUTER_BOUND('',#6600,.T.);
#4414=FACE_OUTER_BOUND('',#6601,.T.);
#4415=FACE_OUTER_BOUND('',#6602,.T.);
#4416=FACE_OUTER_BOUND('',#6603,.T.);
#4417=FACE_OUTER_BOUND('',#6604,.T.);
#4418=FACE_OUTER_BOUND('',#6605,.T.);
#4419=FACE_OUTER_BOUND('',#6606,.T.);
#4420=FACE_OUTER_BOUND('',#6607,.T.);
#4421=FACE_OUTER_BOUND('',#6608,.T.);
#4422=FACE_OUTER_BOUND('',#6609,.T.);
#4423=FACE_OUTER_BOUND('',#6610,.T.);
#4424=FACE_OUTER_BOUND('',#6611,.T.);
#4425=FACE_OUTER_BOUND('',#6612,.T.);
#4426=FACE_OUTER_BOUND('',#6613,.T.);
#4427=FACE_OUTER_BOUND('',#6614,.T.);
#4428=FACE_OUTER_BOUND('',#6615,.T.);
#4429=FACE_OUTER_BOUND('',#6616,.T.);
#4430=FACE_OUTER_BOUND('',#6617,.T.);
#4431=FACE_OUTER_BOUND('',#6618,.T.);
#4432=FACE_OUTER_BOUND('',#6619,.T.);
#4433=FACE_OUTER_BOUND('',#6620,.T.);
#4434=FACE_OUTER_BOUND('',#6621,.T.);
#4435=FACE_OUTER_BOUND('',#6622,.T.);
#4436=FACE_OUTER_BOUND('',#6623,.T.);
#4437=FACE_OUTER_BOUND('',#6624,.T.);
#4438=FACE_OUTER_BOUND('',#6625,.T.);
#4439=FACE_OUTER_BOUND('',#6626,.T.);
#4440=FACE_OUTER_BOUND('',#6627,.T.);
#4441=FACE_OUTER_BOUND('',#6628,.T.);
#4442=FACE_OUTER_BOUND('',#6629,.T.);
#4443=FACE_OUTER_BOUND('',#6630,.T.);
#4444=FACE_OUTER_BOUND('',#6636,.T.);
#4445=FACE_OUTER_BOUND('',#6637,.T.);
#4446=FACE_OUTER_BOUND('',#6638,.T.);
#4447=FACE_OUTER_BOUND('',#6639,.T.);
#4448=FACE_OUTER_BOUND('',#6640,.T.);
#4449=FACE_OUTER_BOUND('',#6641,.T.);
#4450=FACE_OUTER_BOUND('',#6642,.T.);
#4451=FACE_OUTER_BOUND('',#6643,.T.);
#4452=FACE_OUTER_BOUND('',#6644,.T.);
#4453=FACE_OUTER_BOUND('',#6650,.T.);
#4454=FACE_OUTER_BOUND('',#6651,.T.);
#4455=FACE_OUTER_BOUND('',#6652,.T.);
#4456=FACE_OUTER_BOUND('',#6653,.T.);
#4457=FACE_OUTER_BOUND('',#6654,.T.);
#4458=FACE_OUTER_BOUND('',#6655,.T.);
#4459=FACE_OUTER_BOUND('',#6656,.T.);
#4460=FACE_OUTER_BOUND('',#6657,.T.);
#4461=FACE_OUTER_BOUND('',#6658,.T.);
#4462=FACE_OUTER_BOUND('',#6659,.T.);
#4463=FACE_OUTER_BOUND('',#6660,.T.);
#4464=FACE_OUTER_BOUND('',#6661,.T.);
#4465=FACE_OUTER_BOUND('',#6662,.T.);
#4466=FACE_OUTER_BOUND('',#6663,.T.);
#4467=FACE_OUTER_BOUND('',#6664,.T.);
#4468=FACE_OUTER_BOUND('',#6665,.T.);
#4469=FACE_OUTER_BOUND('',#6666,.T.);
#4470=FACE_OUTER_BOUND('',#6667,.T.);
#4471=FACE_OUTER_BOUND('',#6668,.T.);
#4472=FACE_OUTER_BOUND('',#6669,.T.);
#4473=FACE_OUTER_BOUND('',#6670,.T.);
#4474=FACE_OUTER_BOUND('',#6671,.T.);
#4475=FACE_OUTER_BOUND('',#6672,.T.);
#4476=FACE_OUTER_BOUND('',#6673,.T.);
#4477=FACE_OUTER_BOUND('',#6674,.T.);
#4478=FACE_OUTER_BOUND('',#6675,.T.);
#4479=FACE_OUTER_BOUND('',#6676,.T.);
#4480=FACE_OUTER_BOUND('',#6677,.T.);
#4481=FACE_OUTER_BOUND('',#6678,.T.);
#4482=FACE_OUTER_BOUND('',#6679,.T.);
#4483=FACE_OUTER_BOUND('',#6680,.T.);
#4484=FACE_OUTER_BOUND('',#6681,.T.);
#4485=FACE_OUTER_BOUND('',#6682,.T.);
#4486=FACE_OUTER_BOUND('',#6683,.T.);
#4487=FACE_OUTER_BOUND('',#6684,.T.);
#4488=FACE_OUTER_BOUND('',#6685,.T.);
#4489=FACE_OUTER_BOUND('',#6686,.T.);
#4490=FACE_OUTER_BOUND('',#6687,.T.);
#4491=FACE_OUTER_BOUND('',#6688,.T.);
#4492=FACE_OUTER_BOUND('',#6689,.T.);
#4493=FACE_OUTER_BOUND('',#6690,.T.);
#4494=FACE_OUTER_BOUND('',#6691,.T.);
#4495=FACE_OUTER_BOUND('',#6692,.T.);
#4496=FACE_OUTER_BOUND('',#6693,.T.);
#4497=FACE_OUTER_BOUND('',#6694,.T.);
#4498=FACE_OUTER_BOUND('',#6695,.T.);
#4499=FACE_OUTER_BOUND('',#6696,.T.);
#4500=FACE_OUTER_BOUND('',#6697,.T.);
#4501=FACE_OUTER_BOUND('',#6698,.T.);
#4502=FACE_OUTER_BOUND('',#6699,.T.);
#4503=FACE_OUTER_BOUND('',#6700,.T.);
#4504=FACE_OUTER_BOUND('',#6701,.T.);
#4505=FACE_OUTER_BOUND('',#6702,.T.);
#4506=FACE_OUTER_BOUND('',#6703,.T.);
#4507=FACE_OUTER_BOUND('',#6704,.T.);
#4508=FACE_OUTER_BOUND('',#6705,.T.);
#4509=FACE_OUTER_BOUND('',#6706,.T.);
#4510=FACE_OUTER_BOUND('',#6707,.T.);
#4511=FACE_OUTER_BOUND('',#6708,.T.);
#4512=FACE_OUTER_BOUND('',#6709,.T.);
#4513=FACE_OUTER_BOUND('',#6710,.T.);
#4514=FACE_OUTER_BOUND('',#6711,.T.);
#4515=FACE_OUTER_BOUND('',#6713,.T.);
#4516=FACE_OUTER_BOUND('',#6714,.T.);
#4517=FACE_OUTER_BOUND('',#6715,.T.);
#4518=FACE_OUTER_BOUND('',#6716,.T.);
#4519=FACE_OUTER_BOUND('',#6717,.T.);
#4520=FACE_OUTER_BOUND('',#6718,.T.);
#4521=FACE_OUTER_BOUND('',#6719,.T.);
#4522=FACE_OUTER_BOUND('',#6720,.T.);
#4523=FACE_OUTER_BOUND('',#6721,.T.);
#4524=FACE_OUTER_BOUND('',#6723,.T.);
#4525=FACE_OUTER_BOUND('',#6724,.T.);
#4526=FACE_OUTER_BOUND('',#6725,.T.);
#4527=FACE_OUTER_BOUND('',#6726,.T.);
#4528=FACE_OUTER_BOUND('',#6727,.T.);
#6581=EDGE_LOOP('',(#27814,#27815,#27816,#27817,#27818,#27819,#27820));
#6582=EDGE_LOOP('',(#27821,#27822,#27823,#27824));
#6583=EDGE_LOOP('',(#27825,#27826,#27827,#27828));
#6584=EDGE_LOOP('',(#27829,#27830,#27831,#27832));
#6585=EDGE_LOOP('',(#27833,#27834,#27835,#27836));
#6586=EDGE_LOOP('',(#27837,#27838,#27839,#27840));
#6587=EDGE_LOOP('',(#27841,#27842,#27843,#27844));
#6588=EDGE_LOOP('',(#27845,#27846,#27847,#27848));
#6589=EDGE_LOOP('',(#27849,#27850,#27851,#27852));
#6590=EDGE_LOOP('',(#27853,#27854,#27855,#27856));
#6591=EDGE_LOOP('',(#27857,#27858,#27859));
#6592=EDGE_LOOP('',(#27860));
#6593=EDGE_LOOP('',(#27861));
#6594=EDGE_LOOP('',(#27862,#27863,#27864,#27865));
#6595=EDGE_LOOP('',(#27866,#27867,#27868,#27869));
#6596=EDGE_LOOP('',(#27870,#27871,#27872,#27873,#27874,#27875));
#6597=EDGE_LOOP('',(#27876,#27877,#27878,#27879));
#6598=EDGE_LOOP('',(#27880,#27881,#27882,#27883,#27884));
#6599=EDGE_LOOP('',(#27885,#27886,#27887,#27888,#27889,#27890));
#6600=EDGE_LOOP('',(#27891,#27892,#27893));
#6601=EDGE_LOOP('',(#27894,#27895,#27896,#27897,#27898));
#6602=EDGE_LOOP('',(#27899,#27900,#27901,#27902,#27903));
#6603=EDGE_LOOP('',(#27904,#27905,#27906));
#6604=EDGE_LOOP('',(#27907,#27908,#27909,#27910,#27911));
#6605=EDGE_LOOP('',(#27912,#27913,#27914,#27915));
#6606=EDGE_LOOP('',(#27916,#27917,#27918));
#6607=EDGE_LOOP('',(#27919,#27920,#27921,#27922,#27923));
#6608=EDGE_LOOP('',(#27924,#27925,#27926,#27927));
#6609=EDGE_LOOP('',(#27928,#27929,#27930));
#6610=EDGE_LOOP('',(#27931,#27932,#27933,#27934,#27935));
#6611=EDGE_LOOP('',(#27936,#27937,#27938,#27939));
#6612=EDGE_LOOP('',(#27940,#27941,#27942));
#6613=EDGE_LOOP('',(#27943,#27944,#27945,#27946,#27947));
#6614=EDGE_LOOP('',(#27948,#27949,#27950,#27951));
#6615=EDGE_LOOP('',(#27952,#27953,#27954));
#6616=EDGE_LOOP('',(#27955,#27956,#27957,#27958,#27959));
#6617=EDGE_LOOP('',(#27960,#27961,#27962,#27963));
#6618=EDGE_LOOP('',(#27964,#27965,#27966,#27967,#27968));
#6619=EDGE_LOOP('',(#27969,#27970,#27971,#27972,#27973,#27974));
#6620=EDGE_LOOP('',(#27975,#27976,#27977,#27978));
#6621=EDGE_LOOP('',(#27979,#27980,#27981,#27982,#27983,#27984));
#6622=EDGE_LOOP('',(#27985,#27986,#27987,#27988));
#6623=EDGE_LOOP('',(#27989,#27990,#27991,#27992,#27993,#27994));
#6624=EDGE_LOOP('',(#27995,#27996,#27997,#27998));
#6625=EDGE_LOOP('',(#27999,#28000,#28001,#28002,#28003,#28004));
#6626=EDGE_LOOP('',(#28005,#28006,#28007,#28008,#28009));
#6627=EDGE_LOOP('',(#28010,#28011,#28012,#28013));
#6628=EDGE_LOOP('',(#28014,#28015,#28016,#28017,#28018));
#6629=EDGE_LOOP('',(#28019,#28020,#28021,#28022));
#6630=EDGE_LOOP('',(#28023,#28024,#28025,#28026,#28027,#28028,#28029,#28030));
#6631=EDGE_LOOP('',(#28031));
#6632=EDGE_LOOP('',(#28032));
#6633=EDGE_LOOP('',(#28033));
#6634=EDGE_LOOP('',(#28034));
#6635=EDGE_LOOP('',(#28035));
#6636=EDGE_LOOP('',(#28036,#28037,#28038,#28039));
#6637=EDGE_LOOP('',(#28040,#28041,#28042,#28043));
#6638=EDGE_LOOP('',(#28044,#28045,#28046,#28047));
#6639=EDGE_LOOP('',(#28048,#28049,#28050,#28051));
#6640=EDGE_LOOP('',(#28052,#28053,#28054,#28055));
#6641=EDGE_LOOP('',(#28056,#28057,#28058,#28059));
#6642=EDGE_LOOP('',(#28060,#28061,#28062,#28063));
#6643=EDGE_LOOP('',(#28064,#28065,#28066,#28067));
#6644=EDGE_LOOP('',(#28068,#28069,#28070,#28071,#28072,#28073,#28074,#28075));
#6645=EDGE_LOOP('',(#28076));
#6646=EDGE_LOOP('',(#28077));
#6647=EDGE_LOOP('',(#28078));
#6648=EDGE_LOOP('',(#28079));
#6649=EDGE_LOOP('',(#28080));
#6650=EDGE_LOOP('',(#28081,#28082,#28083,#28084));
#6651=EDGE_LOOP('',(#28085,#28086,#28087,#28088));
#6652=EDGE_LOOP('',(#28089,#28090,#28091,#28092));
#6653=EDGE_LOOP('',(#28093,#28094,#28095,#28096,#28097,#28098));
#6654=EDGE_LOOP('',(#28099,#28100,#28101));
#6655=EDGE_LOOP('',(#28102,#28103,#28104,#28105,#28106,#28107));
#6656=EDGE_LOOP('',(#28108,#28109,#28110,#28111));
#6657=EDGE_LOOP('',(#28112,#28113,#28114,#28115));
#6658=EDGE_LOOP('',(#28116,#28117,#28118,#28119));
#6659=EDGE_LOOP('',(#28120,#28121,#28122,#28123,#28124,#28125));
#6660=EDGE_LOOP('',(#28126,#28127,#28128,#28129,#28130,#28131));
#6661=EDGE_LOOP('',(#28132,#28133,#28134,#28135,#28136));
#6662=EDGE_LOOP('',(#28137,#28138,#28139,#28140,#28141));
#6663=EDGE_LOOP('',(#28142));
#6664=EDGE_LOOP('',(#28143,#28144,#28145,#28146,#28147));
#6665=EDGE_LOOP('',(#28148,#28149,#28150,#28151,#28152,#28153,#28154,#28155,
#28156,#28157,#28158,#28159,#28160,#28161));
#6666=EDGE_LOOP('',(#28162,#28163,#28164,#28165,#28166,#28167,#28168,#28169,
#28170,#28171,#28172,#28173,#28174,#28175,#28176,#28177,#28178,#28179,#28180,
#28181,#28182,#28183,#28184));
#6667=EDGE_LOOP('',(#28185,#28186,#28187,#28188));
#6668=EDGE_LOOP('',(#28189,#28190,#28191,#28192));
#6669=EDGE_LOOP('',(#28193,#28194,#28195,#28196));
#6670=EDGE_LOOP('',(#28197,#28198,#28199,#28200,#28201,#28202,#28203,#28204,
#28205,#28206,#28207,#28208,#28209));
#6671=EDGE_LOOP('',(#28210,#28211,#28212,#28213));
#6672=EDGE_LOOP('',(#28214,#28215,#28216,#28217));
#6673=EDGE_LOOP('',(#28218,#28219,#28220,#28221,#28222,#28223,#28224,#28225,
#28226,#28227,#28228,#28229,#28230,#28231,#28232,#28233,#28234,#28235,#28236,
#28237,#28238,#28239));
#6674=EDGE_LOOP('',(#28240,#28241,#28242,#28243));
#6675=EDGE_LOOP('',(#28244,#28245,#28246,#28247,#28248,#28249));
#6676=EDGE_LOOP('',(#28250,#28251,#28252,#28253));
#6677=EDGE_LOOP('',(#28254,#28255,#28256,#28257));
#6678=EDGE_LOOP('',(#28258,#28259,#28260,#28261));
#6679=EDGE_LOOP('',(#28262,#28263,#28264,#28265));
#6680=EDGE_LOOP('',(#28266,#28267,#28268,#28269,#28270));
#6681=EDGE_LOOP('',(#28271,#28272,#28273,#28274,#28275,#28276,#28277));
#6682=EDGE_LOOP('',(#28278,#28279,#28280,#28281));
#6683=EDGE_LOOP('',(#28282,#28283,#28284));
#6684=EDGE_LOOP('',(#28285,#28286,#28287,#28288));
#6685=EDGE_LOOP('',(#28289,#28290,#28291,#28292));
#6686=EDGE_LOOP('',(#28293,#28294,#28295,#28296));
#6687=EDGE_LOOP('',(#28297,#28298,#28299,#28300));
#6688=EDGE_LOOP('',(#28301,#28302,#28303,#28304));
#6689=EDGE_LOOP('',(#28305,#28306,#28307,#28308));
#6690=EDGE_LOOP('',(#28309,#28310,#28311,#28312));
#6691=EDGE_LOOP('',(#28313,#28314,#28315,#28316));
#6692=EDGE_LOOP('',(#28317,#28318,#28319,#28320));
#6693=EDGE_LOOP('',(#28321,#28322,#28323,#28324,#28325,#28326));
#6694=EDGE_LOOP('',(#28327,#28328,#28329,#28330));
#6695=EDGE_LOOP('',(#28331,#28332,#28333,#28334));
#6696=EDGE_LOOP('',(#28335,#28336,#28337,#28338));
#6697=EDGE_LOOP('',(#28339,#28340,#28341,#28342,#28343));
#6698=EDGE_LOOP('',(#28344,#28345,#28346));
#6699=EDGE_LOOP('',(#28347,#28348,#28349,#28350));
#6700=EDGE_LOOP('',(#28351,#28352,#28353,#28354));
#6701=EDGE_LOOP('',(#28355,#28356,#28357,#28358));
#6702=EDGE_LOOP('',(#28359,#28360,#28361,#28362));
#6703=EDGE_LOOP('',(#28363,#28364,#28365,#28366));
#6704=EDGE_LOOP('',(#28367,#28368,#28369,#28370));
#6705=EDGE_LOOP('',(#28371,#28372,#28373,#28374));
#6706=EDGE_LOOP('',(#28375,#28376,#28377,#28378,#28379,#28380,#28381,#28382));
#6707=EDGE_LOOP('',(#28383,#28384,#28385,#28386));
#6708=EDGE_LOOP('',(#28387,#28388,#28389,#28390,#28391,#28392,#28393,#28394,
#28395,#28396,#28397,#28398,#28399,#28400,#28401,#28402,#28403,#28404,#28405,
#28406,#28407,#28408,#28409,#28410,#28411,#28412,#28413,#28414,#28415,#28416,
#28417,#28418,#28419,#28420,#28421,#28422,#28423,#28424,#28425,#28426,#28427,
#28428,#28429,#28430,#28431));
#6709=EDGE_LOOP('',(#28432,#28433,#28434,#28435));
#6710=EDGE_LOOP('',(#28436,#28437,#28438,#28439));
#6711=EDGE_LOOP('',(#28440));
#6712=EDGE_LOOP('',(#28441));
#6713=EDGE_LOOP('',(#28442,#28443,#28444,#28445));
#6714=EDGE_LOOP('',(#28446,#28447,#28448,#28449));
#6715=EDGE_LOOP('',(#28450,#28451,#28452,#28453));
#6716=EDGE_LOOP('',(#28454,#28455,#28456,#28457));
#6717=EDGE_LOOP('',(#28458,#28459,#28460,#28461));
#6718=EDGE_LOOP('',(#28462,#28463,#28464,#28465,#28466));
#6719=EDGE_LOOP('',(#28467,#28468,#28469,#28470,#28471,#28472,#28473,#28474));
#6720=EDGE_LOOP('',(#28475,#28476,#28477,#28478,#28479));
#6721=EDGE_LOOP('',(#28480,#28481,#28482,#28483,#28484));
#6722=EDGE_LOOP('',(#28485));
#6723=EDGE_LOOP('',(#28486,#28487,#28488,#28489));
#6724=EDGE_LOOP('',(#28490,#28491,#28492,#28493,#28494,#28495,#28496,#28497));
#6725=EDGE_LOOP('',(#28498,#28499,#28500,#28501,#28502,#28503,#28504,#28505));
#6726=EDGE_LOOP('',(#28506,#28507));
#6727=EDGE_LOOP('',(#28508,#28509,#28510,#28511));
#9749=LINE('',#52956,#12799);
#9750=LINE('',#53010,#12800);
#9751=LINE('',#53047,#12801);
#9752=LINE('',#53085,#12802);
#9753=LINE('',#53123,#12803);
#9754=LINE('',#53160,#12804);
#9755=LINE('',#53197,#12805);
#9756=LINE('',#53231,#12806);
#9757=LINE('',#53269,#12807);
#9758=LINE('',#53307,#12808);
#9759=LINE('',#53311,#12809);
#9760=LINE('',#53318,#12810);
#9761=LINE('',#53320,#12811);
#9762=LINE('',#53322,#12812);
#9763=LINE('',#53323,#12813);
#9764=LINE('',#53326,#12814);
#9765=LINE('',#53328,#12815);
#9766=LINE('',#53329,#12816);
#9767=LINE('',#53333,#12817);
#9768=LINE('',#53335,#12818);
#9769=LINE('',#53337,#12819);
#9770=LINE('',#53339,#12820);
#9771=LINE('',#53341,#12821);
#9772=LINE('',#53342,#12822);
#9773=LINE('',#53345,#12823);
#9774=LINE('',#53347,#12824);
#9775=LINE('',#53348,#12825);
#9776=LINE('',#53351,#12826);
#9777=LINE('',#53353,#12827);
#9778=LINE('',#53354,#12828);
#9779=LINE('',#53357,#12829);
#9780=LINE('',#53359,#12830);
#9781=LINE('',#53361,#12831);
#9782=LINE('',#53362,#12832);
#9783=LINE('',#53366,#12833);
#9784=LINE('',#53368,#12834);
#9785=LINE('',#53369,#12835);
#9786=LINE('',#53371,#12836);
#9787=LINE('',#53373,#12837);
#9788=LINE('',#53374,#12838);
#9789=LINE('',#53377,#12839);
#9790=LINE('',#53378,#12840);
#9791=LINE('',#53379,#12841);
#9792=LINE('',#53383,#12842);
#9793=LINE('',#53385,#12843);
#9794=LINE('',#53386,#12844);
#9795=LINE('',#53390,#12845);
#9796=LINE('',#53391,#12846);
#9797=LINE('',#53393,#12847);
#9798=LINE('',#53394,#12848);
#9799=LINE('',#53396,#12849);
#9800=LINE('',#53397,#12850);
#9801=LINE('',#53401,#12851);
#9802=LINE('',#53403,#12852);
#9803=LINE('',#53404,#12853);
#9804=LINE('',#53408,#12854);
#9805=LINE('',#53409,#12855);
#9806=LINE('',#53411,#12856);
#9807=LINE('',#53412,#12857);
#9808=LINE('',#53414,#12858);
#9809=LINE('',#53415,#12859);
#9810=LINE('',#53419,#12860);
#9811=LINE('',#53421,#12861);
#9812=LINE('',#53422,#12862);
#9813=LINE('',#53426,#12863);
#9814=LINE('',#53427,#12864);
#9815=LINE('',#53429,#12865);
#9816=LINE('',#53430,#12866);
#9817=LINE('',#53432,#12867);
#9818=LINE('',#53433,#12868);
#9819=LINE('',#53437,#12869);
#9820=LINE('',#53439,#12870);
#9821=LINE('',#53440,#12871);
#9822=LINE('',#53444,#12872);
#9823=LINE('',#53445,#12873);
#9824=LINE('',#53447,#12874);
#9825=LINE('',#53448,#12875);
#9826=LINE('',#53450,#12876);
#9827=LINE('',#53451,#12877);
#9828=LINE('',#53455,#12878);
#9829=LINE('',#53457,#12879);
#9830=LINE('',#53458,#12880);
#9831=LINE('',#53462,#12881);
#9832=LINE('',#53463,#12882);
#9833=LINE('',#53465,#12883);
#9834=LINE('',#53466,#12884);
#9835=LINE('',#53468,#12885);
#9836=LINE('',#53469,#12886);
#9837=LINE('',#53473,#12887);
#9838=LINE('',#53474,#12888);
#9839=LINE('',#53476,#12889);
#9840=LINE('',#53477,#12890);
#9841=LINE('',#53480,#12891);
#9842=LINE('',#53482,#12892);
#9843=LINE('',#53483,#12893);
#9844=LINE('',#53484,#12894);
#9845=LINE('',#53486,#12895);
#9846=LINE('',#53489,#12896);
#9847=LINE('',#53490,#12897);
#9848=LINE('',#53492,#12898);
#9849=LINE('',#53495,#12899);
#9850=LINE('',#53496,#12900);
#9851=LINE('',#53498,#12901);
#9852=LINE('',#53501,#12902);
#9853=LINE('',#53502,#12903);
#9854=LINE('',#53505,#12904);
#9855=LINE('',#53506,#12905);
#9856=LINE('',#53507,#12906);
#9857=LINE('',#53509,#12907);
#9858=LINE('',#53511,#12908);
#9859=LINE('',#53512,#12909);
#9860=LINE('',#53517,#12910);
#9861=LINE('',#53520,#12911);
#9862=LINE('',#53532,#12912);
#9863=LINE('',#53535,#12913);
#9864=LINE('',#53540,#12914);
#9865=LINE('',#53543,#12915);
#9866=LINE('',#53548,#12916);
#9867=LINE('',#53551,#12917);
#9868=LINE('',#53556,#12918);
#9869=LINE('',#53560,#12919);
#9870=LINE('',#53562,#12920);
#9871=LINE('',#53572,#12921);
#9872=LINE('',#53574,#12922);
#9873=LINE('',#53576,#12923);
#9874=LINE('',#53578,#12924);
#9875=LINE('',#53590,#12925);
#9876=LINE('',#53596,#12926);
#9877=LINE('',#53601,#12927);
#9878=LINE('',#53604,#12928);
#9879=LINE('',#57693,#12929);
#9880=LINE('',#57787,#12930);
#9881=LINE('',#57789,#12931);
#9882=LINE('',#57790,#12932);
#9883=LINE('',#57792,#12933);
#9884=LINE('',#57793,#12934);
#9885=LINE('',#57795,#12935);
#9886=LINE('',#57796,#12936);
#9887=LINE('',#57798,#12937);
#9888=LINE('',#57799,#12938);
#9889=LINE('',#57801,#12939);
#9890=LINE('',#57802,#12940);
#9891=LINE('',#57804,#12941);
#9892=LINE('',#57805,#12942);
#9893=LINE('',#57807,#12943);
#9894=LINE('',#57808,#12944);
#9895=LINE('',#57810,#12945);
#9896=LINE('',#57811,#12946);
#9897=LINE('',#57814,#12947);
#9898=LINE('',#57819,#12948);
#9899=LINE('',#57822,#12949);
#9900=LINE('',#57823,#12950);
#9901=LINE('',#57883,#12951);
#9902=LINE('',#57891,#12952);
#9903=LINE('',#57895,#12953);
#9904=LINE('',#57902,#12954);
#9905=LINE('',#57906,#12955);
#9906=LINE('',#57910,#12956);
#9907=LINE('',#57914,#12957);
#9908=LINE('',#57919,#12958);
#9909=LINE('',#57920,#12959);
#9910=LINE('',#57923,#12960);
#9911=LINE('',#57924,#12961);
#9912=LINE('',#57927,#12962);
#9913=LINE('',#57930,#12963);
#9914=LINE('',#57933,#12964);
#9915=LINE('',#57940,#12965);
#9916=LINE('',#57945,#12966);
#9917=LINE('',#57947,#12967);
#12799=VECTOR('',#43482,11.59764);
#12800=VECTOR('',#43485,11.59764);
#12801=VECTOR('',#43488,11.59764);
#12802=VECTOR('',#43491,11.59764);
#12803=VECTOR('',#43494,11.59764);
#12804=VECTOR('',#43497,11.59764);
#12805=VECTOR('',#43500,11.59764);
#12806=VECTOR('',#43505,11.59764);
#12807=VECTOR('',#43508,11.59764);
#12808=VECTOR('',#43513,3.02920176969664);
#12809=VECTOR('',#43518,1.5);
#12810=VECTOR('',#43525,10.);
#12811=VECTOR('',#43526,10.);
#12812=VECTOR('',#43527,10.);
#12813=VECTOR('',#43528,10.);
#12814=VECTOR('',#43531,10.);
#12815=VECTOR('',#43532,10.);
#12816=VECTOR('',#43533,10.);
#12817=VECTOR('',#43536,10.);
#12818=VECTOR('',#43537,10.);
#12819=VECTOR('',#43538,10.);
#12820=VECTOR('',#43539,10.);
#12821=VECTOR('',#43540,10.);
#12822=VECTOR('',#43541,10.);
#12823=VECTOR('',#43544,10.);
#12824=VECTOR('',#43545,10.);
#12825=VECTOR('',#43546,10.);
#12826=VECTOR('',#43549,10.);
#12827=VECTOR('',#43550,10.);
#12828=VECTOR('',#43551,10.);
#12829=VECTOR('',#43554,10.);
#12830=VECTOR('',#43555,10.);
#12831=VECTOR('',#43556,10.);
#12832=VECTOR('',#43557,10.);
#12833=VECTOR('',#43560,10.);
#12834=VECTOR('',#43561,10.);
#12835=VECTOR('',#43562,10.);
#12836=VECTOR('',#43565,10.);
#12837=VECTOR('',#43566,10.);
#12838=VECTOR('',#43567,10.);
#12839=VECTOR('',#43570,10.);
#12840=VECTOR('',#43571,10.);
#12841=VECTOR('',#43572,10.);
#12842=VECTOR('',#43575,10.);
#12843=VECTOR('',#43576,10.);
#12844=VECTOR('',#43577,10.);
#12845=VECTOR('',#43580,10.);
#12846=VECTOR('',#43581,10.);
#12847=VECTOR('',#43582,10.);
#12848=VECTOR('',#43583,10.);
#12849=VECTOR('',#43586,10.);
#12850=VECTOR('',#43587,10.);
#12851=VECTOR('',#43590,10.);
#12852=VECTOR('',#43591,10.);
#12853=VECTOR('',#43592,10.);
#12854=VECTOR('',#43595,10.);
#12855=VECTOR('',#43596,10.);
#12856=VECTOR('',#43597,10.);
#12857=VECTOR('',#43598,10.);
#12858=VECTOR('',#43601,10.);
#12859=VECTOR('',#43602,10.);
#12860=VECTOR('',#43605,10.);
#12861=VECTOR('',#43606,10.);
#12862=VECTOR('',#43607,10.);
#12863=VECTOR('',#43610,10.);
#12864=VECTOR('',#43611,10.);
#12865=VECTOR('',#43612,10.);
#12866=VECTOR('',#43613,10.);
#12867=VECTOR('',#43616,10.);
#12868=VECTOR('',#43617,10.);
#12869=VECTOR('',#43620,10.);
#12870=VECTOR('',#43621,10.);
#12871=VECTOR('',#43622,10.);
#12872=VECTOR('',#43625,10.);
#12873=VECTOR('',#43626,10.);
#12874=VECTOR('',#43627,10.);
#12875=VECTOR('',#43628,10.);
#12876=VECTOR('',#43631,10.);
#12877=VECTOR('',#43632,10.);
#12878=VECTOR('',#43635,10.);
#12879=VECTOR('',#43636,10.);
#12880=VECTOR('',#43637,10.);
#12881=VECTOR('',#43640,10.);
#12882=VECTOR('',#43641,10.);
#12883=VECTOR('',#43642,10.);
#12884=VECTOR('',#43643,10.);
#12885=VECTOR('',#43646,10.);
#12886=VECTOR('',#43647,10.);
#12887=VECTOR('',#43650,10.);
#12888=VECTOR('',#43651,10.);
#12889=VECTOR('',#43652,10.);
#12890=VECTOR('',#43653,10.);
#12891=VECTOR('',#43656,10.);
#12892=VECTOR('',#43657,10.);
#12893=VECTOR('',#43658,10.);
#12894=VECTOR('',#43659,10.);
#12895=VECTOR('',#43662,10.);
#12896=VECTOR('',#43665,10.);
#12897=VECTOR('',#43666,10.);
#12898=VECTOR('',#43669,10.);
#12899=VECTOR('',#43672,10.);
#12900=VECTOR('',#43673,10.);
#12901=VECTOR('',#43676,10.);
#12902=VECTOR('',#43679,10.);
#12903=VECTOR('',#43680,10.);
#12904=VECTOR('',#43683,10.);
#12905=VECTOR('',#43684,10.);
#12906=VECTOR('',#43685,10.);
#12907=VECTOR('',#43688,10.);
#12908=VECTOR('',#43691,10.);
#12909=VECTOR('',#43692,10.);
#12910=VECTOR('',#43697,7.);
#12911=VECTOR('',#43702,10.);
#12912=VECTOR('',#43715,6.75);
#12913=VECTOR('',#43718,7.);
#12914=VECTOR('',#43725,6.75);
#12915=VECTOR('',#43728,7.);
#12916=VECTOR('',#43735,6.75);
#12917=VECTOR('',#43738,7.);
#12918=VECTOR('',#43745,6.75);
#12919=VECTOR('',#43750,7.);
#12920=VECTOR('',#43753,10.);
#12921=VECTOR('',#43764,7.);
#12922=VECTOR('',#43767,7.);
#12923=VECTOR('',#43770,7.);
#12924=VECTOR('',#43773,10.);
#12925=VECTOR('',#43790,25.2232233047034);
#12926=VECTOR('',#43797,25.);
#12927=VECTOR('',#43804,25.4);
#12928=VECTOR('',#43807,24.5267766952966);
#12929=VECTOR('',#43832,10.);
#12930=VECTOR('',#43843,10.);
#12931=VECTOR('',#43846,10.);
#12932=VECTOR('',#43847,10.);
#12933=VECTOR('',#43850,10.);
#12934=VECTOR('',#43851,10.);
#12935=VECTOR('',#43854,10.);
#12936=VECTOR('',#43855,10.);
#12937=VECTOR('',#43858,10.);
#12938=VECTOR('',#43859,10.);
#12939=VECTOR('',#43862,10.);
#12940=VECTOR('',#43863,10.);
#12941=VECTOR('',#43866,10.);
#12942=VECTOR('',#43867,10.);
#12943=VECTOR('',#43870,10.);
#12944=VECTOR('',#43871,10.);
#12945=VECTOR('',#43874,10.);
#12946=VECTOR('',#43875,10.);
#12947=VECTOR('',#43878,10.);
#12948=VECTOR('',#43879,10.);
#12949=VECTOR('',#43884,10.);
#12950=VECTOR('',#43885,10.);
#12951=VECTOR('',#43922,2.20000000000001);
#12952=VECTOR('',#43927,23.61565);
#12953=VECTOR('',#43932,21.8313);
#12954=VECTOR('',#43941,17.72);
#12955=VECTOR('',#43946,17.47);
#12956=VECTOR('',#43951,15.72);
#12957=VECTOR('',#43956,13.72);
#12958=VECTOR('',#43961,10.);
#12959=VECTOR('',#43962,10.);
#12960=VECTOR('',#43965,10.);
#12961=VECTOR('',#43966,10.);
#12962=VECTOR('',#43969,10.);
#12963=VECTOR('',#43972,13.47);
#12964=VECTOR('',#43977,10.);
#12965=VECTOR('',#43986,11.9);
#12966=VECTOR('',#43989,12.3);
#12967=VECTOR('',#43992,12.35);
#13889=CIRCLE('',#36174,11.59764);
#13890=CIRCLE('',#36178,3.4268292682927);
#13891=CIRCLE('',#36179,2.63157427110059);
#13892=CIRCLE('',#36182,12.);
#13893=CIRCLE('',#36219,7.25);
#13894=CIRCLE('',#36220,6.75);
#13895=CIRCLE('',#36222,7.25);
#13896=CIRCLE('',#36223,7.25);
#13897=CIRCLE('',#36224,25.4);
#13898=CIRCLE('',#36225,7.25);
#13899=CIRCLE('',#36227,6.75);
#13900=CIRCLE('',#36229,6.75);
#13901=CIRCLE('',#36231,6.75);
#13902=CIRCLE('',#36233,6.75);
#13903=CIRCLE('',#36235,6.75);
#13904=CIRCLE('',#36237,6.75);
#13905=CIRCLE('',#36239,6.75);
#13906=CIRCLE('',#36241,7.25);
#13907=CIRCLE('',#36243,7.25);
#13908=CIRCLE('',#36244,7.25);
#13909=CIRCLE('',#36245,25.4);
#13910=CIRCLE('',#36246,7.25);
#13911=CIRCLE('',#36257,25.4);
#13912=CIRCLE('',#36258,25.4);
#13913=CIRCLE('',#36259,25.0464466094067);
#13914=CIRCLE('',#36260,25.0464466094067);
#13915=CIRCLE('',#36262,24.9535533905933);
#13916=CIRCLE('',#36263,24.9535533905933);
#13917=CIRCLE('',#36266,24.1);
#13918=CIRCLE('',#36270,11.59764);
#13919=CIRCLE('',#36275,12.61364);
#13920=CIRCLE('',#36276,12.61364);
#13921=CIRCLE('',#36278,12.61364);
#13922=CIRCLE('',#36279,12.61364);
#13923=CIRCLE('',#36280,12.61364);
#13924=CIRCLE('',#36282,2.20000000000001);
#13925=CIRCLE('',#36293,2.20000000000001);
#13926=CIRCLE('',#36298,12.61364);
#13927=CIRCLE('',#36300,12.61364);
#13928=CIRCLE('',#36308,12.61364);
#13929=CIRCLE('',#36313,21.8313);
#13930=CIRCLE('',#36315,21.8313);
#13931=CIRCLE('',#36317,17.97);
#13932=CIRCLE('',#36319,17.47);
#13933=CIRCLE('',#36321,17.47);
#13934=CIRCLE('',#36323,13.97);
#13935=CIRCLE('',#36325,13.47);
#13936=CIRCLE('',#36327,13.47);
#13937=CIRCLE('',#36330,13.47);
#13938=CIRCLE('',#36331,13.47);
#13939=CIRCLE('',#36334,11.9);
#13940=CIRCLE('',#36336,11.9);
#16125=VERTEX_POINT('',#52954);
#16126=VERTEX_POINT('',#52955);
#16127=VERTEX_POINT('',#52957);
#16128=VERTEX_POINT('',#52971);
#16129=VERTEX_POINT('',#52976);
#16130=VERTEX_POINT('',#52986);
#16131=VERTEX_POINT('',#52993);
#16132=VERTEX_POINT('',#53008);
#16133=VERTEX_POINT('',#53009);
#16134=VERTEX_POINT('',#53045);
#16135=VERTEX_POINT('',#53046);
#16136=VERTEX_POINT('',#53083);
#16137=VERTEX_POINT('',#53084);
#16138=VERTEX_POINT('',#53121);
#16139=VERTEX_POINT('',#53122);
#16140=VERTEX_POINT('',#53158);
#16141=VERTEX_POINT('',#53159);
#16142=VERTEX_POINT('',#53195);
#16143=VERTEX_POINT('',#53196);
#16144=VERTEX_POINT('',#53198);
#16145=VERTEX_POINT('',#53214);
#16146=VERTEX_POINT('',#53229);
#16147=VERTEX_POINT('',#53230);
#16148=VERTEX_POINT('',#53267);
#16149=VERTEX_POINT('',#53268);
#16150=VERTEX_POINT('',#53304);
#16151=VERTEX_POINT('',#53306);
#16152=VERTEX_POINT('',#53310);
#16153=VERTEX_POINT('',#53313);
#16154=VERTEX_POINT('',#53316);
#16155=VERTEX_POINT('',#53317);
#16156=VERTEX_POINT('',#53319);
#16157=VERTEX_POINT('',#53321);
#16158=VERTEX_POINT('',#53325);
#16159=VERTEX_POINT('',#53327);
#16160=VERTEX_POINT('',#53331);
#16161=VERTEX_POINT('',#53332);
#16162=VERTEX_POINT('',#53334);
#16163=VERTEX_POINT('',#53336);
#16164=VERTEX_POINT('',#53338);
#16165=VERTEX_POINT('',#53340);
#16166=VERTEX_POINT('',#53344);
#16167=VERTEX_POINT('',#53346);
#16168=VERTEX_POINT('',#53350);
#16169=VERTEX_POINT('',#53352);
#16170=VERTEX_POINT('',#53356);
#16171=VERTEX_POINT('',#53358);
#16172=VERTEX_POINT('',#53360);
#16173=VERTEX_POINT('',#53364);
#16174=VERTEX_POINT('',#53365);
#16175=VERTEX_POINT('',#53367);
#16176=VERTEX_POINT('',#53372);
#16177=VERTEX_POINT('',#53376);
#16178=VERTEX_POINT('',#53381);
#16179=VERTEX_POINT('',#53382);
#16180=VERTEX_POINT('',#53384);
#16181=VERTEX_POINT('',#53388);
#16182=VERTEX_POINT('',#53389);
#16183=VERTEX_POINT('',#53392);
#16184=VERTEX_POINT('',#53399);
#16185=VERTEX_POINT('',#53400);
#16186=VERTEX_POINT('',#53402);
#16187=VERTEX_POINT('',#53406);
#16188=VERTEX_POINT('',#53407);
#16189=VERTEX_POINT('',#53410);
#16190=VERTEX_POINT('',#53417);
#16191=VERTEX_POINT('',#53418);
#16192=VERTEX_POINT('',#53420);
#16193=VERTEX_POINT('',#53424);
#16194=VERTEX_POINT('',#53425);
#16195=VERTEX_POINT('',#53428);
#16196=VERTEX_POINT('',#53435);
#16197=VERTEX_POINT('',#53436);
#16198=VERTEX_POINT('',#53438);
#16199=VERTEX_POINT('',#53442);
#16200=VERTEX_POINT('',#53443);
#16201=VERTEX_POINT('',#53446);
#16202=VERTEX_POINT('',#53453);
#16203=VERTEX_POINT('',#53454);
#16204=VERTEX_POINT('',#53456);
#16205=VERTEX_POINT('',#53460);
#16206=VERTEX_POINT('',#53461);
#16207=VERTEX_POINT('',#53464);
#16208=VERTEX_POINT('',#53471);
#16209=VERTEX_POINT('',#53472);
#16210=VERTEX_POINT('',#53475);
#16211=VERTEX_POINT('',#53479);
#16212=VERTEX_POINT('',#53481);
#16213=VERTEX_POINT('',#53488);
#16214=VERTEX_POINT('',#53494);
#16215=VERTEX_POINT('',#53500);
#16216=VERTEX_POINT('',#53504);
#16217=VERTEX_POINT('',#53514);
#16218=VERTEX_POINT('',#53516);
#16219=VERTEX_POINT('',#53521);
#16220=VERTEX_POINT('',#53523);
#16221=VERTEX_POINT('',#53525);
#16222=VERTEX_POINT('',#53527);
#16223=VERTEX_POINT('',#53530);
#16224=VERTEX_POINT('',#53534);
#16225=VERTEX_POINT('',#53538);
#16226=VERTEX_POINT('',#53542);
#16227=VERTEX_POINT('',#53546);
#16228=VERTEX_POINT('',#53550);
#16229=VERTEX_POINT('',#53554);
#16230=VERTEX_POINT('',#53558);
#16231=VERTEX_POINT('',#53563);
#16232=VERTEX_POINT('',#53565);
#16233=VERTEX_POINT('',#53567);
#16234=VERTEX_POINT('',#53569);
#16235=VERTEX_POINT('',#53585);
#16236=VERTEX_POINT('',#53586);
#16237=VERTEX_POINT('',#53589);
#16238=VERTEX_POINT('',#53591);
#16239=VERTEX_POINT('',#53595);
#16240=VERTEX_POINT('',#53597);
#16241=VERTEX_POINT('',#53603);
#16242=VERTEX_POINT('',#53643);
#16243=VERTEX_POINT('',#53644);
#16244=VERTEX_POINT('',#53661);
#16245=VERTEX_POINT('',#53671);
#16246=VERTEX_POINT('',#53682);
#16247=VERTEX_POINT('',#53903);
#16248=VERTEX_POINT('',#53904);
#16249=VERTEX_POINT('',#53951);
#16250=VERTEX_POINT('',#53995);
#16251=VERTEX_POINT('',#54042);
#16252=VERTEX_POINT('',#54083);
#16253=VERTEX_POINT('',#54133);
#16254=VERTEX_POINT('',#54174);
#16255=VERTEX_POINT('',#54185);
#16256=VERTEX_POINT('',#54209);
#16257=VERTEX_POINT('',#54681);
#16258=VERTEX_POINT('',#54682);
#16259=VERTEX_POINT('',#54729);
#16260=VERTEX_POINT('',#54749);
#16261=VERTEX_POINT('',#54886);
#16262=VERTEX_POINT('',#54893);
#16263=VERTEX_POINT('',#54898);
#16264=VERTEX_POINT('',#54939);
#16265=VERTEX_POINT('',#54986);
#16266=VERTEX_POINT('',#55030);
#16267=VERTEX_POINT('',#55077);
#16268=VERTEX_POINT('',#55118);
#16269=VERTEX_POINT('',#55165);
#16270=VERTEX_POINT('',#55206);
#16271=VERTEX_POINT('',#55256);
#16272=VERTEX_POINT('',#55297);
#16273=VERTEX_POINT('',#55423);
#16274=VERTEX_POINT('',#55437);
#16275=VERTEX_POINT('',#55512);
#16276=VERTEX_POINT('',#55513);
#16277=VERTEX_POINT('',#55527);
#16278=VERTEX_POINT('',#55547);
#16279=VERTEX_POINT('',#55609);
#16280=VERTEX_POINT('',#55610);
#16281=VERTEX_POINT('',#55627);
#16282=VERTEX_POINT('',#55637);
#16283=VERTEX_POINT('',#55858);
#16284=VERTEX_POINT('',#55859);
#16285=VERTEX_POINT('',#55906);
#16286=VERTEX_POINT('',#56071);
#16287=VERTEX_POINT('',#56079);
#16288=VERTEX_POINT('',#56090);
#16289=VERTEX_POINT('',#56113);
#16290=VERTEX_POINT('',#56160);
#16291=VERTEX_POINT('',#56201);
#16292=VERTEX_POINT('',#56327);
#16293=VERTEX_POINT('',#56328);
#16294=VERTEX_POINT('',#56345);
#16295=VERTEX_POINT('',#56365);
#16296=VERTEX_POINT('',#56419);
#16297=VERTEX_POINT('',#56420);
#16298=VERTEX_POINT('',#56437);
#16299=VERTEX_POINT('',#56457);
#16300=VERTEX_POINT('',#56820);
#16301=VERTEX_POINT('',#56821);
#16302=VERTEX_POINT('',#56868);
#16303=VERTEX_POINT('',#56912);
#16304=VERTEX_POINT('',#56959);
#16305=VERTEX_POINT('',#57000);
#16306=VERTEX_POINT('',#57047);
#16307=VERTEX_POINT('',#57088);
#16308=VERTEX_POINT('',#57138);
#16309=VERTEX_POINT('',#57179);
#16310=VERTEX_POINT('',#57229);
#16311=VERTEX_POINT('',#57270);
#16312=VERTEX_POINT('',#57317);
#16313=VERTEX_POINT('',#57362);
#16314=VERTEX_POINT('',#57375);
#16315=VERTEX_POINT('',#57564);
#16316=VERTEX_POINT('',#57565);
#16317=VERTEX_POINT('',#57579);
#16318=VERTEX_POINT('',#57589);
#16319=VERTEX_POINT('',#57667);
#16320=VERTEX_POINT('',#57672);
#16321=VERTEX_POINT('',#57687);
#16322=VERTEX_POINT('',#57691);
#16323=VERTEX_POINT('',#57692);
#16324=VERTEX_POINT('',#57695);
#16325=VERTEX_POINT('',#57734);
#16326=VERTEX_POINT('',#57751);
#16327=VERTEX_POINT('',#57785);
#16328=VERTEX_POINT('',#57813);
#16329=VERTEX_POINT('',#57815);
#16330=VERTEX_POINT('',#57854);
#16331=VERTEX_POINT('',#57889);
#16332=VERTEX_POINT('',#57893);
#16333=VERTEX_POINT('',#57897);
#16334=VERTEX_POINT('',#57900);
#16335=VERTEX_POINT('',#57904);
#16336=VERTEX_POINT('',#57908);
#16337=VERTEX_POINT('',#57912);
#16338=VERTEX_POINT('',#57916);
#16339=VERTEX_POINT('',#57917);
#16340=VERTEX_POINT('',#57922);
#16341=VERTEX_POINT('',#57926);
#16342=VERTEX_POINT('',#57928);
#16343=VERTEX_POINT('',#57935);
#16344=VERTEX_POINT('',#57938);
#20221=EDGE_CURVE('',#16125,#16126,#9749,.T.);
#20222=EDGE_CURVE('',#16125,#16127,#357,.T.);
#20223=EDGE_CURVE('',#16128,#16127,#358,.T.);
#20224=EDGE_CURVE('',#16129,#16128,#359,.T.);
#20225=EDGE_CURVE('',#16130,#16129,#360,.T.);
#20226=EDGE_CURVE('',#16131,#16130,#361,.T.);
#20227=EDGE_CURVE('',#16126,#16131,#362,.T.);
#20228=EDGE_CURVE('',#16132,#16133,#9750,.T.);
#20229=EDGE_CURVE('',#16132,#16125,#363,.T.);
#20230=EDGE_CURVE('',#16133,#16126,#364,.T.);
#20231=EDGE_CURVE('',#16134,#16135,#9751,.T.);
#20232=EDGE_CURVE('',#16134,#16132,#365,.T.);
#20233=EDGE_CURVE('',#16135,#16133,#366,.T.);
#20234=EDGE_CURVE('',#16136,#16137,#9752,.T.);
#20235=EDGE_CURVE('',#16136,#16134,#367,.T.);
#20236=EDGE_CURVE('',#16137,#16135,#368,.T.);
#20237=EDGE_CURVE('',#16138,#16139,#9753,.T.);
#20238=EDGE_CURVE('',#16138,#16136,#369,.T.);
#20239=EDGE_CURVE('',#16139,#16137,#370,.T.);
#20240=EDGE_CURVE('',#16140,#16141,#9754,.T.);
#20241=EDGE_CURVE('',#16140,#16138,#371,.T.);
#20242=EDGE_CURVE('',#16141,#16139,#372,.T.);
#20243=EDGE_CURVE('',#16142,#16143,#9755,.T.);
#20244=EDGE_CURVE('',#16142,#16144,#373,.T.);
#20245=EDGE_CURVE('',#16145,#16144,#13889,.T.);
#20246=EDGE_CURVE('',#16143,#16145,#374,.T.);
#20247=EDGE_CURVE('',#16146,#16147,#9756,.T.);
#20248=EDGE_CURVE('',#16146,#16142,#375,.T.);
#20249=EDGE_CURVE('',#16147,#16143,#376,.T.);
#20250=EDGE_CURVE('',#16148,#16149,#9757,.T.);
#20251=EDGE_CURVE('',#16148,#16146,#377,.T.);
#20252=EDGE_CURVE('',#16149,#16147,#378,.T.);
#20253=EDGE_CURVE('',#16150,#16150,#13890,.T.);
#20254=EDGE_CURVE('',#16150,#16151,#9758,.T.);
#20255=EDGE_CURVE('',#16151,#16151,#13891,.T.);
#20256=EDGE_CURVE('',#16152,#16151,#9759,.T.);
#20257=EDGE_CURVE('',#16153,#16153,#13892,.T.);
#20258=EDGE_CURVE('',#16154,#16155,#9760,.F.);
#20259=EDGE_CURVE('',#16155,#16156,#9761,.T.);
#20260=EDGE_CURVE('',#16156,#16157,#9762,.F.);
#20261=EDGE_CURVE('',#16157,#16154,#9763,.T.);
#20262=EDGE_CURVE('',#16155,#16158,#9764,.T.);
#20263=EDGE_CURVE('',#16158,#16159,#9765,.T.);
#20264=EDGE_CURVE('',#16156,#16159,#9766,.T.);
#20265=EDGE_CURVE('',#16160,#16161,#9767,.T.);
#20266=EDGE_CURVE('',#16161,#16162,#9768,.T.);
#20267=EDGE_CURVE('',#16162,#16163,#9769,.T.);
#20268=EDGE_CURVE('',#16163,#16164,#9770,.T.);
#20269=EDGE_CURVE('',#16164,#16165,#9771,.T.);
#20270=EDGE_CURVE('',#16165,#16160,#9772,.T.);
#20271=EDGE_CURVE('',#16166,#16164,#9773,.T.);
#20272=EDGE_CURVE('',#16167,#16166,#9774,.T.);
#20273=EDGE_CURVE('',#16165,#16167,#9775,.T.);
#20274=EDGE_CURVE('',#16168,#16163,#9776,.T.);
#20275=EDGE_CURVE('',#16168,#16169,#9777,.T.);
#20276=EDGE_CURVE('',#16169,#16166,#9778,.T.);
#20277=EDGE_CURVE('',#16162,#16170,#9779,.T.);
#20278=EDGE_CURVE('',#16171,#16170,#9780,.T.);
#20279=EDGE_CURVE('',#16172,#16171,#9781,.T.);
#20280=EDGE_CURVE('',#16172,#16168,#9782,.T.);
#20281=EDGE_CURVE('',#16173,#16174,#9783,.T.);
#20282=EDGE_CURVE('',#16175,#16173,#9784,.T.);
#20283=EDGE_CURVE('',#16174,#16175,#9785,.T.);
#20284=EDGE_CURVE('',#16170,#16175,#9786,.T.);
#20285=EDGE_CURVE('',#16173,#16176,#9787,.T.);
#20286=EDGE_CURVE('',#16176,#16171,#9788,.T.);
#20287=EDGE_CURVE('',#16160,#16177,#9789,.T.);
#20288=EDGE_CURVE('',#16177,#16174,#9790,.T.);
#20289=EDGE_CURVE('',#16175,#16161,#9791,.T.);
#20290=EDGE_CURVE('',#16178,#16179,#9792,.T.);
#20291=EDGE_CURVE('',#16180,#16178,#9793,.T.);
#20292=EDGE_CURVE('',#16179,#16180,#9794,.T.);
#20293=EDGE_CURVE('',#16181,#16182,#9795,.T.);
#20294=EDGE_CURVE('',#16182,#16180,#9796,.T.);
#20295=EDGE_CURVE('',#16178,#16183,#9797,.T.);
#20296=EDGE_CURVE('',#16183,#16181,#9798,.T.);
#20297=EDGE_CURVE('',#16174,#16179,#9799,.T.);
#20298=EDGE_CURVE('',#16180,#16173,#9800,.T.);
#20299=EDGE_CURVE('',#16184,#16185,#9801,.T.);
#20300=EDGE_CURVE('',#16186,#16184,#9802,.T.);
#20301=EDGE_CURVE('',#16185,#16186,#9803,.T.);
#20302=EDGE_CURVE('',#16187,#16188,#9804,.T.);
#20303=EDGE_CURVE('',#16188,#16186,#9805,.T.);
#20304=EDGE_CURVE('',#16184,#16189,#9806,.T.);
#20305=EDGE_CURVE('',#16189,#16187,#9807,.T.);
#20306=EDGE_CURVE('',#16179,#16185,#9808,.T.);
#20307=EDGE_CURVE('',#16186,#16178,#9809,.T.);
#20308=EDGE_CURVE('',#16190,#16191,#9810,.T.);
#20309=EDGE_CURVE('',#16192,#16190,#9811,.T.);
#20310=EDGE_CURVE('',#16191,#16192,#9812,.T.);
#20311=EDGE_CURVE('',#16193,#16194,#9813,.T.);
#20312=EDGE_CURVE('',#16194,#16192,#9814,.T.);
#20313=EDGE_CURVE('',#16190,#16195,#9815,.T.);
#20314=EDGE_CURVE('',#16195,#16193,#9816,.T.);
#20315=EDGE_CURVE('',#16185,#16191,#9817,.T.);
#20316=EDGE_CURVE('',#16192,#16184,#9818,.T.);
#20317=EDGE_CURVE('',#16196,#16197,#9819,.T.);
#20318=EDGE_CURVE('',#16198,#16196,#9820,.T.);
#20319=EDGE_CURVE('',#16197,#16198,#9821,.T.);
#20320=EDGE_CURVE('',#16199,#16200,#9822,.T.);
#20321=EDGE_CURVE('',#16200,#16198,#9823,.T.);
#20322=EDGE_CURVE('',#16196,#16201,#9824,.T.);
#20323=EDGE_CURVE('',#16201,#16199,#9825,.T.);
#20324=EDGE_CURVE('',#16191,#16197,#9826,.T.);
#20325=EDGE_CURVE('',#16198,#16190,#9827,.T.);
#20326=EDGE_CURVE('',#16202,#16203,#9828,.T.);
#20327=EDGE_CURVE('',#16204,#16202,#9829,.T.);
#20328=EDGE_CURVE('',#16203,#16204,#9830,.T.);
#20329=EDGE_CURVE('',#16205,#16206,#9831,.T.);
#20330=EDGE_CURVE('',#16206,#16204,#9832,.T.);
#20331=EDGE_CURVE('',#16202,#16207,#9833,.T.);
#20332=EDGE_CURVE('',#16207,#16205,#9834,.T.);
#20333=EDGE_CURVE('',#16197,#16203,#9835,.T.);
#20334=EDGE_CURVE('',#16204,#16196,#9836,.T.);
#20335=EDGE_CURVE('',#16208,#16209,#9837,.T.);
#20336=EDGE_CURVE('',#16209,#16202,#9838,.T.);
#20337=EDGE_CURVE('',#16203,#16210,#9839,.T.);
#20338=EDGE_CURVE('',#16210,#16208,#9840,.T.);
#20339=EDGE_CURVE('',#16211,#16187,#9841,.T.);
#20340=EDGE_CURVE('',#16211,#16212,#9842,.T.);
#20341=EDGE_CURVE('',#16212,#16181,#9843,.T.);
#20342=EDGE_CURVE('',#16183,#16188,#9844,.T.);
#20343=EDGE_CURVE('',#16189,#16194,#9845,.T.);
#20344=EDGE_CURVE('',#16213,#16193,#9846,.T.);
#20345=EDGE_CURVE('',#16213,#16211,#9847,.T.);
#20346=EDGE_CURVE('',#16195,#16200,#9848,.T.);
#20347=EDGE_CURVE('',#16214,#16199,#9849,.T.);
#20348=EDGE_CURVE('',#16214,#16213,#9850,.T.);
#20349=EDGE_CURVE('',#16201,#16206,#9851,.T.);
#20350=EDGE_CURVE('',#16215,#16205,#9852,.T.);
#20351=EDGE_CURVE('',#16215,#16214,#9853,.T.);
#20352=EDGE_CURVE('',#16207,#16216,#9854,.T.);
#20353=EDGE_CURVE('',#16216,#16169,#9855,.T.);
#20354=EDGE_CURVE('',#16169,#16215,#9856,.T.);
#20355=EDGE_CURVE('',#16216,#16209,#9857,.T.);
#20356=EDGE_CURVE('',#16208,#16167,#9858,.T.);
#20357=EDGE_CURVE('',#16166,#16216,#9859,.T.);
#20358=EDGE_CURVE('',#16217,#16217,#13893,.T.);
#20359=EDGE_CURVE('',#16217,#16218,#9860,.T.);
#20360=EDGE_CURVE('',#16218,#16218,#13894,.T.);
#20361=EDGE_CURVE('',#16210,#16177,#9861,.T.);
#20362=EDGE_CURVE('',#16219,#16219,#13895,.T.);
#20363=EDGE_CURVE('',#16220,#16220,#13896,.T.);
#20364=EDGE_CURVE('',#16221,#16221,#13897,.T.);
#20365=EDGE_CURVE('',#16222,#16222,#13898,.T.);
#20366=EDGE_CURVE('',#16223,#16223,#13899,.T.);
#20367=EDGE_CURVE('',#16223,#16218,#9862,.T.);
#20368=EDGE_CURVE('',#16219,#16224,#9863,.T.);
#20369=EDGE_CURVE('',#16224,#16224,#13900,.T.);
#20370=EDGE_CURVE('',#16225,#16225,#13901,.T.);
#20371=EDGE_CURVE('',#16225,#16224,#9864,.T.);
#20372=EDGE_CURVE('',#16222,#16226,#9865,.T.);
#20373=EDGE_CURVE('',#16226,#16226,#13902,.T.);
#20374=EDGE_CURVE('',#16227,#16227,#13903,.T.);
#20375=EDGE_CURVE('',#16227,#16226,#9866,.T.);
#20376=EDGE_CURVE('',#16220,#16228,#9867,.T.);
#20377=EDGE_CURVE('',#16228,#16228,#13904,.T.);
#20378=EDGE_CURVE('',#16229,#16229,#13905,.T.);
#20379=EDGE_CURVE('',#16229,#16228,#9868,.T.);
#20380=EDGE_CURVE('',#16230,#16230,#13906,.T.);
#20381=EDGE_CURVE('',#16230,#16229,#9869,.T.);
#20382=EDGE_CURVE('',#16212,#16172,#9870,.T.);
#20383=EDGE_CURVE('',#16231,#16231,#13907,.T.);
#20384=EDGE_CURVE('',#16232,#16232,#13908,.T.);
#20385=EDGE_CURVE('',#16233,#16233,#13909,.T.);
#20386=EDGE_CURVE('',#16234,#16234,#13910,.T.);
#20387=EDGE_CURVE('',#16231,#16227,#9871,.T.);
#20388=EDGE_CURVE('',#16234,#16225,#9872,.T.);
#20389=EDGE_CURVE('',#16232,#16223,#9873,.T.);
#20390=EDGE_CURVE('',#16176,#16182,#9874,.T.);
#20391=EDGE_CURVE('',#16235,#16236,#13911,.T.);
#20392=EDGE_CURVE('',#16236,#16235,#13912,.T.);
#20393=EDGE_CURVE('',#16235,#16237,#9875,.T.);
#20394=EDGE_CURVE('',#16237,#16238,#13913,.T.);
#20395=EDGE_CURVE('',#16238,#16237,#13914,.T.);
#20396=EDGE_CURVE('',#16238,#16239,#9876,.T.);
#20397=EDGE_CURVE('',#16240,#16239,#13915,.T.);
#20398=EDGE_CURVE('',#16239,#16240,#13916,.T.);
#20399=EDGE_CURVE('',#16233,#16236,#9877,.T.);
#20400=EDGE_CURVE('',#16240,#16241,#9878,.T.);
#20401=EDGE_CURVE('',#16241,#16241,#13917,.T.);
#20402=EDGE_CURVE('',#16242,#16243,#379,.T.);
#20403=EDGE_CURVE('',#16242,#16244,#380,.T.);
#20404=EDGE_CURVE('',#16245,#16244,#381,.T.);
#20405=EDGE_CURVE('',#16246,#16245,#382,.T.);
#20406=EDGE_CURVE('',#16243,#16246,#383,.T.);
#20407=EDGE_CURVE('',#16247,#16248,#384,.T.);
#20408=EDGE_CURVE('',#16249,#16247,#385,.T.);
#20409=EDGE_CURVE('',#16250,#16249,#386,.T.);
#20410=EDGE_CURVE('',#16251,#16250,#387,.T.);
#20411=EDGE_CURVE('',#16252,#16251,#388,.T.);
#20412=EDGE_CURVE('',#16253,#16252,#389,.T.);
#20413=EDGE_CURVE('',#16254,#16253,#390,.T.);
#20414=EDGE_CURVE('',#16255,#16254,#391,.T.);
#20415=EDGE_CURVE('',#16255,#16149,#392,.T.);
#20416=EDGE_CURVE('',#16256,#16145,#393,.T.);
#20417=EDGE_CURVE('',#16248,#16256,#394,.T.);
#20418=EDGE_CURVE('',#16257,#16258,#395,.T.);
#20419=EDGE_CURVE('',#16259,#16257,#396,.T.);
#20420=EDGE_CURVE('',#16260,#16259,#397,.T.);
#20421=EDGE_CURVE('',#16260,#16141,#398,.T.);
#20422=EDGE_CURVE('',#16261,#16131,#399,.T.);
#20423=EDGE_CURVE('',#16262,#16261,#400,.T.);
#20424=EDGE_CURVE('',#16263,#16262,#401,.T.);
#20425=EDGE_CURVE('',#16264,#16263,#402,.T.);
#20426=EDGE_CURVE('',#16265,#16264,#403,.T.);
#20427=EDGE_CURVE('',#16266,#16265,#404,.T.);
#20428=EDGE_CURVE('',#16267,#16266,#405,.T.);
#20429=EDGE_CURVE('',#16268,#16267,#406,.T.);
#20430=EDGE_CURVE('',#16269,#16268,#407,.T.);
#20431=EDGE_CURVE('',#16270,#16269,#408,.T.);
#20432=EDGE_CURVE('',#16271,#16270,#409,.T.);
#20433=EDGE_CURVE('',#16272,#16271,#410,.T.);
#20434=EDGE_CURVE('',#16258,#16272,#411,.T.);
#20435=EDGE_CURVE('',#16273,#16128,#412,.T.);
#20436=EDGE_CURVE('',#16274,#16273,#413,.T.);
#20437=EDGE_CURVE('',#16129,#16274,#414,.T.);
#20438=EDGE_CURVE('',#16275,#16276,#415,.T.);
#20439=EDGE_CURVE('',#16277,#16275,#416,.T.);
#20440=EDGE_CURVE('',#16278,#16277,#417,.T.);
#20441=EDGE_CURVE('',#16278,#16276,#418,.T.);
#20442=EDGE_CURVE('',#16279,#16280,#419,.T.);
#20443=EDGE_CURVE('',#16279,#16281,#420,.T.);
#20444=EDGE_CURVE('',#16282,#16281,#421,.T.);
#20445=EDGE_CURVE('',#16280,#16282,#422,.T.);
#20446=EDGE_CURVE('',#16283,#16284,#423,.T.);
#20447=EDGE_CURVE('',#16285,#16283,#424,.T.);
#20448=EDGE_CURVE('',#16144,#16285,#425,.T.);
#20449=EDGE_CURVE('',#16286,#16148,#426,.T.);
#20450=EDGE_CURVE('',#16287,#16286,#427,.T.);
#20451=EDGE_CURVE('',#16288,#16287,#428,.T.);
#20452=EDGE_CURVE('',#16289,#16288,#429,.T.);
#20453=EDGE_CURVE('',#16290,#16289,#430,.T.);
#20454=EDGE_CURVE('',#16291,#16290,#431,.T.);
#20455=EDGE_CURVE('',#16284,#16291,#432,.T.);
#20456=EDGE_CURVE('',#16292,#16293,#433,.T.);
#20457=EDGE_CURVE('',#16294,#16292,#434,.T.);
#20458=EDGE_CURVE('',#16295,#16294,#435,.T.);
#20459=EDGE_CURVE('',#16293,#16295,#436,.T.);
#20460=EDGE_CURVE('',#16296,#16297,#437,.T.);
#20461=EDGE_CURVE('',#16298,#16296,#438,.T.);
#20462=EDGE_CURVE('',#16299,#16298,#439,.T.);
#20463=EDGE_CURVE('',#16297,#16299,#440,.T.);
#20464=EDGE_CURVE('',#16300,#16301,#441,.T.);
#20465=EDGE_CURVE('',#16302,#16300,#442,.T.);
#20466=EDGE_CURVE('',#16303,#16302,#443,.T.);
#20467=EDGE_CURVE('',#16304,#16303,#444,.T.);
#20468=EDGE_CURVE('',#16305,#16304,#445,.T.);
#20469=EDGE_CURVE('',#16306,#16305,#446,.T.);
#20470=EDGE_CURVE('',#16307,#16306,#447,.T.);
#20471=EDGE_CURVE('',#16308,#16307,#448,.T.);
#20472=EDGE_CURVE('',#16309,#16308,#449,.T.);
#20473=EDGE_CURVE('',#16310,#16309,#450,.T.);
#20474=EDGE_CURVE('',#16311,#16310,#451,.T.);
#20475=EDGE_CURVE('',#16312,#16311,#452,.T.);
#20476=EDGE_CURVE('',#16127,#16312,#453,.T.);
#20477=EDGE_CURVE('',#16313,#16140,#454,.T.);
#20478=EDGE_CURVE('',#16314,#16313,#455,.T.);
#20479=EDGE_CURVE('',#16301,#16314,#456,.T.);
#20480=EDGE_CURVE('',#16315,#16316,#457,.T.);
#20481=EDGE_CURVE('',#16317,#16315,#458,.T.);
#20482=EDGE_CURVE('',#16318,#16317,#459,.T.);
#20483=EDGE_CURVE('',#16316,#16318,#460,.T.);
#20484=EDGE_CURVE('',#16293,#16255,#461,.T.);
#20485=EDGE_CURVE('',#16286,#16295,#462,.T.);
#20486=EDGE_CURVE('',#16313,#16260,#13918,.T.);
#20487=EDGE_CURVE('',#16297,#16242,#463,.T.);
#20488=EDGE_CURVE('',#16244,#16299,#464,.T.);
#20489=EDGE_CURVE('',#16276,#16315,#465,.T.);
#20490=EDGE_CURVE('',#16317,#16278,#466,.T.);
#20491=EDGE_CURVE('',#16319,#16279,#467,.T.);
#20492=EDGE_CURVE('',#16319,#16320,#468,.T.);
#20493=EDGE_CURVE('',#16281,#16320,#469,.T.);
#20494=EDGE_CURVE('',#16321,#16285,#13919,.F.);
#20495=EDGE_CURVE('',#16256,#16321,#13920,.F.);
#20496=EDGE_CURVE('',#16322,#16323,#9879,.T.);
#20497=EDGE_CURVE('',#16322,#16314,#13921,.T.);
#20498=EDGE_CURVE('',#16259,#16324,#13922,.T.);
#20499=EDGE_CURVE('',#16324,#16323,#13923,.T.);
#20500=EDGE_CURVE('',#16325,#16319,#470,.T.);
#20501=EDGE_CURVE('',#16326,#16325,#471,.T.);
#20502=EDGE_CURVE('',#16320,#16326,#472,.T.);
#20503=EDGE_CURVE('',#16327,#16261,#13924,.T.);
#20504=EDGE_CURVE('',#16262,#16327,#9880,.F.);
#20505=EDGE_CURVE('',#16264,#16310,#9881,.F.);
#20506=EDGE_CURVE('',#16311,#16263,#9882,.F.);
#20507=EDGE_CURVE('',#16309,#16265,#9883,.F.);
#20508=EDGE_CURVE('',#16266,#16308,#9884,.F.);
#20509=EDGE_CURVE('',#16307,#16267,#9885,.F.);
#20510=EDGE_CURVE('',#16268,#16306,#9886,.F.);
#20511=EDGE_CURVE('',#16305,#16269,#9887,.F.);
#20512=EDGE_CURVE('',#16270,#16304,#9888,.F.);
#20513=EDGE_CURVE('',#16303,#16271,#9889,.F.);
#20514=EDGE_CURVE('',#16272,#16302,#9890,.F.);
#20515=EDGE_CURVE('',#16300,#16258,#9891,.F.);
#20516=EDGE_CURVE('',#16257,#16301,#9892,.F.);
#20517=EDGE_CURVE('',#16252,#16290,#9893,.F.);
#20518=EDGE_CURVE('',#16291,#16251,#9894,.F.);
#20519=EDGE_CURVE('',#16250,#16284,#9895,.F.);
#20520=EDGE_CURVE('',#16283,#16249,#9896,.F.);
#20521=EDGE_CURVE('',#16328,#16248,#9897,.F.);
#20522=EDGE_CURVE('',#16329,#16328,#181,.T.);
#20523=EDGE_CURVE('',#16247,#16329,#9898,.F.);
#20524=EDGE_CURVE('',#16254,#16245,#13925,.T.);
#20525=EDGE_CURVE('',#16289,#16253,#9899,.F.);
#20526=EDGE_CURVE('',#16246,#16288,#9900,.F.);
#20527=EDGE_CURVE('',#16287,#16243,#473,.F.);
#20528=EDGE_CURVE('',#16285,#16329,#13926,.F.);
#20529=EDGE_CURVE('',#16328,#16256,#13927,.F.);
#20530=EDGE_CURVE('',#16282,#16294,#474,.F.);
#20531=EDGE_CURVE('',#16292,#16280,#475,.T.);
#20532=EDGE_CURVE('',#16314,#16259,#13928,.T.);
#20533=EDGE_CURVE('',#16318,#16330,#476,.F.);
#20534=EDGE_CURVE('',#16330,#16312,#477,.F.);
#20535=EDGE_CURVE('',#16327,#16316,#478,.T.);
#20536=EDGE_CURVE('',#16275,#16298,#479,.T.);
#20537=EDGE_CURVE('',#16296,#16277,#480,.F.);
#20538=EDGE_CURVE('',#16273,#16326,#481,.F.);
#20539=EDGE_CURVE('',#16330,#16130,#9901,.T.);
#20540=EDGE_CURVE('',#16325,#16274,#482,.T.);
#20541=EDGE_CURVE('',#16331,#16331,#13929,.T.);
#20542=EDGE_CURVE('',#16331,#16221,#9902,.T.);
#20543=EDGE_CURVE('',#16332,#16332,#13930,.T.);
#20544=EDGE_CURVE('',#16332,#16331,#9903,.T.);
#20545=EDGE_CURVE('',#16333,#16333,#13931,.T.);
#20546=EDGE_CURVE('',#16334,#16334,#13932,.T.);
#20547=EDGE_CURVE('',#16334,#16333,#9904,.T.);
#20548=EDGE_CURVE('',#16335,#16335,#13933,.T.);
#20549=EDGE_CURVE('',#16335,#16334,#9905,.T.);
#20550=EDGE_CURVE('',#16336,#16336,#13934,.T.);
#20551=EDGE_CURVE('',#16336,#16335,#9906,.T.);
#20552=EDGE_CURVE('',#16337,#16337,#13935,.T.);
#20553=EDGE_CURVE('',#16337,#16336,#9907,.T.);
#20554=EDGE_CURVE('',#16338,#16339,#13936,.T.);
#20555=EDGE_CURVE('',#16159,#16338,#9908,.T.);
#20556=EDGE_CURVE('',#16339,#16158,#9909,.T.);
#20557=EDGE_CURVE('',#16340,#16154,#9910,.T.);
#20558=EDGE_CURVE('',#16339,#16340,#9911,.T.);
#20559=EDGE_CURVE('',#16341,#16338,#9912,.T.);
#20560=EDGE_CURVE('',#16342,#16340,#13937,.T.);
#20561=EDGE_CURVE('',#16342,#16337,#9913,.T.);
#20562=EDGE_CURVE('',#16341,#16342,#13938,.T.);
#20563=EDGE_CURVE('',#16157,#16341,#9914,.T.);
#20564=EDGE_CURVE('',#16343,#16343,#13939,.T.);
#20565=EDGE_CURVE('',#16344,#16344,#13940,.T.);
#20566=EDGE_CURVE('',#16344,#16343,#9915,.T.);
#20567=EDGE_CURVE('',#16322,#16323,#182,.T.);
#20568=EDGE_CURVE('',#16324,#16344,#9916,.T.);
#20569=EDGE_CURVE('',#16153,#16321,#9917,.T.);
#27814=ORIENTED_EDGE('',*,*,#20221,.F.);
#27815=ORIENTED_EDGE('',*,*,#20222,.T.);
#27816=ORIENTED_EDGE('',*,*,#20223,.F.);
#27817=ORIENTED_EDGE('',*,*,#20224,.F.);
#27818=ORIENTED_EDGE('',*,*,#20225,.F.);
#27819=ORIENTED_EDGE('',*,*,#20226,.F.);
#27820=ORIENTED_EDGE('',*,*,#20227,.F.);
#27821=ORIENTED_EDGE('',*,*,#20228,.F.);
#27822=ORIENTED_EDGE('',*,*,#20229,.T.);
#27823=ORIENTED_EDGE('',*,*,#20221,.T.);
#27824=ORIENTED_EDGE('',*,*,#20230,.F.);
#27825=ORIENTED_EDGE('',*,*,#20231,.F.);
#27826=ORIENTED_EDGE('',*,*,#20232,.T.);
#27827=ORIENTED_EDGE('',*,*,#20228,.T.);
#27828=ORIENTED_EDGE('',*,*,#20233,.F.);
#27829=ORIENTED_EDGE('',*,*,#20234,.F.);
#27830=ORIENTED_EDGE('',*,*,#20235,.T.);
#27831=ORIENTED_EDGE('',*,*,#20231,.T.);
#27832=ORIENTED_EDGE('',*,*,#20236,.F.);
#27833=ORIENTED_EDGE('',*,*,#20237,.F.);
#27834=ORIENTED_EDGE('',*,*,#20238,.T.);
#27835=ORIENTED_EDGE('',*,*,#20234,.T.);
#27836=ORIENTED_EDGE('',*,*,#20239,.F.);
#27837=ORIENTED_EDGE('',*,*,#20240,.F.);
#27838=ORIENTED_EDGE('',*,*,#20241,.T.);
#27839=ORIENTED_EDGE('',*,*,#20237,.T.);
#27840=ORIENTED_EDGE('',*,*,#20242,.F.);
#27841=ORIENTED_EDGE('',*,*,#20243,.F.);
#27842=ORIENTED_EDGE('',*,*,#20244,.T.);
#27843=ORIENTED_EDGE('',*,*,#20245,.F.);
#27844=ORIENTED_EDGE('',*,*,#20246,.F.);
#27845=ORIENTED_EDGE('',*,*,#20247,.F.);
#27846=ORIENTED_EDGE('',*,*,#20248,.T.);
#27847=ORIENTED_EDGE('',*,*,#20243,.T.);
#27848=ORIENTED_EDGE('',*,*,#20249,.F.);
#27849=ORIENTED_EDGE('',*,*,#20250,.F.);
#27850=ORIENTED_EDGE('',*,*,#20251,.T.);
#27851=ORIENTED_EDGE('',*,*,#20247,.T.);
#27852=ORIENTED_EDGE('',*,*,#20252,.F.);
#27853=ORIENTED_EDGE('',*,*,#20253,.T.);
#27854=ORIENTED_EDGE('',*,*,#20254,.T.);
#27855=ORIENTED_EDGE('',*,*,#20255,.T.);
#27856=ORIENTED_EDGE('',*,*,#20254,.F.);
#27857=ORIENTED_EDGE('',*,*,#20256,.T.);
#27858=ORIENTED_EDGE('',*,*,#20255,.F.);
#27859=ORIENTED_EDGE('',*,*,#20256,.F.);
#27860=ORIENTED_EDGE('',*,*,#20257,.T.);
#27861=ORIENTED_EDGE('',*,*,#20253,.F.);
#27862=ORIENTED_EDGE('',*,*,#20258,.T.);
#27863=ORIENTED_EDGE('',*,*,#20259,.T.);
#27864=ORIENTED_EDGE('',*,*,#20260,.T.);
#27865=ORIENTED_EDGE('',*,*,#20261,.T.);
#27866=ORIENTED_EDGE('',*,*,#20259,.F.);
#27867=ORIENTED_EDGE('',*,*,#20262,.T.);
#27868=ORIENTED_EDGE('',*,*,#20263,.T.);
#27869=ORIENTED_EDGE('',*,*,#20264,.F.);
#27870=ORIENTED_EDGE('',*,*,#20265,.T.);
#27871=ORIENTED_EDGE('',*,*,#20266,.T.);
#27872=ORIENTED_EDGE('',*,*,#20267,.T.);
#27873=ORIENTED_EDGE('',*,*,#20268,.T.);
#27874=ORIENTED_EDGE('',*,*,#20269,.T.);
#27875=ORIENTED_EDGE('',*,*,#20270,.T.);
#27876=ORIENTED_EDGE('',*,*,#20269,.F.);
#27877=ORIENTED_EDGE('',*,*,#20271,.F.);
#27878=ORIENTED_EDGE('',*,*,#20272,.F.);
#27879=ORIENTED_EDGE('',*,*,#20273,.F.);
#27880=ORIENTED_EDGE('',*,*,#20268,.F.);
#27881=ORIENTED_EDGE('',*,*,#20274,.F.);
#27882=ORIENTED_EDGE('',*,*,#20275,.T.);
#27883=ORIENTED_EDGE('',*,*,#20276,.T.);
#27884=ORIENTED_EDGE('',*,*,#20271,.T.);
#27885=ORIENTED_EDGE('',*,*,#20267,.F.);
#27886=ORIENTED_EDGE('',*,*,#20277,.T.);
#27887=ORIENTED_EDGE('',*,*,#20278,.F.);
#27888=ORIENTED_EDGE('',*,*,#20279,.F.);
#27889=ORIENTED_EDGE('',*,*,#20280,.T.);
#27890=ORIENTED_EDGE('',*,*,#20274,.T.);
#27891=ORIENTED_EDGE('',*,*,#20281,.F.);
#27892=ORIENTED_EDGE('',*,*,#20282,.F.);
#27893=ORIENTED_EDGE('',*,*,#20283,.F.);
#27894=ORIENTED_EDGE('',*,*,#20278,.T.);
#27895=ORIENTED_EDGE('',*,*,#20284,.T.);
#27896=ORIENTED_EDGE('',*,*,#20282,.T.);
#27897=ORIENTED_EDGE('',*,*,#20285,.T.);
#27898=ORIENTED_EDGE('',*,*,#20286,.T.);
#27899=ORIENTED_EDGE('',*,*,#20265,.F.);
#27900=ORIENTED_EDGE('',*,*,#20287,.T.);
#27901=ORIENTED_EDGE('',*,*,#20288,.T.);
#27902=ORIENTED_EDGE('',*,*,#20283,.T.);
#27903=ORIENTED_EDGE('',*,*,#20289,.T.);
#27904=ORIENTED_EDGE('',*,*,#20290,.F.);
#27905=ORIENTED_EDGE('',*,*,#20291,.F.);
#27906=ORIENTED_EDGE('',*,*,#20292,.F.);
#27907=ORIENTED_EDGE('',*,*,#20293,.T.);
#27908=ORIENTED_EDGE('',*,*,#20294,.T.);
#27909=ORIENTED_EDGE('',*,*,#20291,.T.);
#27910=ORIENTED_EDGE('',*,*,#20295,.T.);
#27911=ORIENTED_EDGE('',*,*,#20296,.T.);
#27912=ORIENTED_EDGE('',*,*,#20281,.T.);
#27913=ORIENTED_EDGE('',*,*,#20297,.T.);
#27914=ORIENTED_EDGE('',*,*,#20292,.T.);
#27915=ORIENTED_EDGE('',*,*,#20298,.T.);
#27916=ORIENTED_EDGE('',*,*,#20299,.F.);
#27917=ORIENTED_EDGE('',*,*,#20300,.F.);
#27918=ORIENTED_EDGE('',*,*,#20301,.F.);
#27919=ORIENTED_EDGE('',*,*,#20302,.T.);
#27920=ORIENTED_EDGE('',*,*,#20303,.T.);
#27921=ORIENTED_EDGE('',*,*,#20300,.T.);
#27922=ORIENTED_EDGE('',*,*,#20304,.T.);
#27923=ORIENTED_EDGE('',*,*,#20305,.T.);
#27924=ORIENTED_EDGE('',*,*,#20290,.T.);
#27925=ORIENTED_EDGE('',*,*,#20306,.T.);
#27926=ORIENTED_EDGE('',*,*,#20301,.T.);
#27927=ORIENTED_EDGE('',*,*,#20307,.T.);
#27928=ORIENTED_EDGE('',*,*,#20308,.F.);
#27929=ORIENTED_EDGE('',*,*,#20309,.F.);
#27930=ORIENTED_EDGE('',*,*,#20310,.F.);
#27931=ORIENTED_EDGE('',*,*,#20311,.T.);
#27932=ORIENTED_EDGE('',*,*,#20312,.T.);
#27933=ORIENTED_EDGE('',*,*,#20309,.T.);
#27934=ORIENTED_EDGE('',*,*,#20313,.T.);
#27935=ORIENTED_EDGE('',*,*,#20314,.T.);
#27936=ORIENTED_EDGE('',*,*,#20299,.T.);
#27937=ORIENTED_EDGE('',*,*,#20315,.T.);
#27938=ORIENTED_EDGE('',*,*,#20310,.T.);
#27939=ORIENTED_EDGE('',*,*,#20316,.T.);
#27940=ORIENTED_EDGE('',*,*,#20317,.F.);
#27941=ORIENTED_EDGE('',*,*,#20318,.F.);
#27942=ORIENTED_EDGE('',*,*,#20319,.F.);
#27943=ORIENTED_EDGE('',*,*,#20320,.T.);
#27944=ORIENTED_EDGE('',*,*,#20321,.T.);
#27945=ORIENTED_EDGE('',*,*,#20318,.T.);
#27946=ORIENTED_EDGE('',*,*,#20322,.T.);
#27947=ORIENTED_EDGE('',*,*,#20323,.T.);
#27948=ORIENTED_EDGE('',*,*,#20308,.T.);
#27949=ORIENTED_EDGE('',*,*,#20324,.T.);
#27950=ORIENTED_EDGE('',*,*,#20319,.T.);
#27951=ORIENTED_EDGE('',*,*,#20325,.T.);
#27952=ORIENTED_EDGE('',*,*,#20326,.F.);
#27953=ORIENTED_EDGE('',*,*,#20327,.F.);
#27954=ORIENTED_EDGE('',*,*,#20328,.F.);
#27955=ORIENTED_EDGE('',*,*,#20329,.T.);
#27956=ORIENTED_EDGE('',*,*,#20330,.T.);
#27957=ORIENTED_EDGE('',*,*,#20327,.T.);
#27958=ORIENTED_EDGE('',*,*,#20331,.T.);
#27959=ORIENTED_EDGE('',*,*,#20332,.T.);
#27960=ORIENTED_EDGE('',*,*,#20317,.T.);
#27961=ORIENTED_EDGE('',*,*,#20333,.T.);
#27962=ORIENTED_EDGE('',*,*,#20328,.T.);
#27963=ORIENTED_EDGE('',*,*,#20334,.T.);
#27964=ORIENTED_EDGE('',*,*,#20335,.T.);
#27965=ORIENTED_EDGE('',*,*,#20336,.T.);
#27966=ORIENTED_EDGE('',*,*,#20326,.T.);
#27967=ORIENTED_EDGE('',*,*,#20337,.T.);
#27968=ORIENTED_EDGE('',*,*,#20338,.T.);
#27969=ORIENTED_EDGE('',*,*,#20302,.F.);
#27970=ORIENTED_EDGE('',*,*,#20339,.F.);
#27971=ORIENTED_EDGE('',*,*,#20340,.T.);
#27972=ORIENTED_EDGE('',*,*,#20341,.T.);
#27973=ORIENTED_EDGE('',*,*,#20296,.F.);
#27974=ORIENTED_EDGE('',*,*,#20342,.T.);
#27975=ORIENTED_EDGE('',*,*,#20304,.F.);
#27976=ORIENTED_EDGE('',*,*,#20316,.F.);
#27977=ORIENTED_EDGE('',*,*,#20312,.F.);
#27978=ORIENTED_EDGE('',*,*,#20343,.F.);
#27979=ORIENTED_EDGE('',*,*,#20305,.F.);
#27980=ORIENTED_EDGE('',*,*,#20343,.T.);
#27981=ORIENTED_EDGE('',*,*,#20311,.F.);
#27982=ORIENTED_EDGE('',*,*,#20344,.F.);
#27983=ORIENTED_EDGE('',*,*,#20345,.T.);
#27984=ORIENTED_EDGE('',*,*,#20339,.T.);
#27985=ORIENTED_EDGE('',*,*,#20313,.F.);
#27986=ORIENTED_EDGE('',*,*,#20325,.F.);
#27987=ORIENTED_EDGE('',*,*,#20321,.F.);
#27988=ORIENTED_EDGE('',*,*,#20346,.F.);
#27989=ORIENTED_EDGE('',*,*,#20314,.F.);
#27990=ORIENTED_EDGE('',*,*,#20346,.T.);
#27991=ORIENTED_EDGE('',*,*,#20320,.F.);
#27992=ORIENTED_EDGE('',*,*,#20347,.F.);
#27993=ORIENTED_EDGE('',*,*,#20348,.T.);
#27994=ORIENTED_EDGE('',*,*,#20344,.T.);
#27995=ORIENTED_EDGE('',*,*,#20322,.F.);
#27996=ORIENTED_EDGE('',*,*,#20334,.F.);
#27997=ORIENTED_EDGE('',*,*,#20330,.F.);
#27998=ORIENTED_EDGE('',*,*,#20349,.F.);
#27999=ORIENTED_EDGE('',*,*,#20323,.F.);
#28000=ORIENTED_EDGE('',*,*,#20349,.T.);
#28001=ORIENTED_EDGE('',*,*,#20329,.F.);
#28002=ORIENTED_EDGE('',*,*,#20350,.F.);
#28003=ORIENTED_EDGE('',*,*,#20351,.T.);
#28004=ORIENTED_EDGE('',*,*,#20347,.T.);
#28005=ORIENTED_EDGE('',*,*,#20332,.F.);
#28006=ORIENTED_EDGE('',*,*,#20352,.T.);
#28007=ORIENTED_EDGE('',*,*,#20353,.T.);
#28008=ORIENTED_EDGE('',*,*,#20354,.T.);
#28009=ORIENTED_EDGE('',*,*,#20350,.T.);
#28010=ORIENTED_EDGE('',*,*,#20331,.F.);
#28011=ORIENTED_EDGE('',*,*,#20336,.F.);
#28012=ORIENTED_EDGE('',*,*,#20355,.F.);
#28013=ORIENTED_EDGE('',*,*,#20352,.F.);
#28014=ORIENTED_EDGE('',*,*,#20335,.F.);
#28015=ORIENTED_EDGE('',*,*,#20356,.T.);
#28016=ORIENTED_EDGE('',*,*,#20272,.T.);
#28017=ORIENTED_EDGE('',*,*,#20357,.T.);
#28018=ORIENTED_EDGE('',*,*,#20355,.T.);
#28019=ORIENTED_EDGE('',*,*,#20358,.T.);
#28020=ORIENTED_EDGE('',*,*,#20359,.T.);
#28021=ORIENTED_EDGE('',*,*,#20360,.T.);
#28022=ORIENTED_EDGE('',*,*,#20359,.F.);
#28023=ORIENTED_EDGE('',*,*,#20288,.F.);
#28024=ORIENTED_EDGE('',*,*,#20361,.F.);
#28025=ORIENTED_EDGE('',*,*,#20337,.F.);
#28026=ORIENTED_EDGE('',*,*,#20333,.F.);
#28027=ORIENTED_EDGE('',*,*,#20324,.F.);
#28028=ORIENTED_EDGE('',*,*,#20315,.F.);
#28029=ORIENTED_EDGE('',*,*,#20306,.F.);
#28030=ORIENTED_EDGE('',*,*,#20297,.F.);
#28031=ORIENTED_EDGE('',*,*,#20362,.F.);
#28032=ORIENTED_EDGE('',*,*,#20363,.F.);
#28033=ORIENTED_EDGE('',*,*,#20364,.F.);
#28034=ORIENTED_EDGE('',*,*,#20365,.F.);
#28035=ORIENTED_EDGE('',*,*,#20358,.F.);
#28036=ORIENTED_EDGE('',*,*,#20366,.F.);
#28037=ORIENTED_EDGE('',*,*,#20367,.T.);
#28038=ORIENTED_EDGE('',*,*,#20360,.F.);
#28039=ORIENTED_EDGE('',*,*,#20367,.F.);
#28040=ORIENTED_EDGE('',*,*,#20362,.T.);
#28041=ORIENTED_EDGE('',*,*,#20368,.T.);
#28042=ORIENTED_EDGE('',*,*,#20369,.T.);
#28043=ORIENTED_EDGE('',*,*,#20368,.F.);
#28044=ORIENTED_EDGE('',*,*,#20370,.F.);
#28045=ORIENTED_EDGE('',*,*,#20371,.T.);
#28046=ORIENTED_EDGE('',*,*,#20369,.F.);
#28047=ORIENTED_EDGE('',*,*,#20371,.F.);
#28048=ORIENTED_EDGE('',*,*,#20365,.T.);
#28049=ORIENTED_EDGE('',*,*,#20372,.T.);
#28050=ORIENTED_EDGE('',*,*,#20373,.T.);
#28051=ORIENTED_EDGE('',*,*,#20372,.F.);
#28052=ORIENTED_EDGE('',*,*,#20374,.F.);
#28053=ORIENTED_EDGE('',*,*,#20375,.T.);
#28054=ORIENTED_EDGE('',*,*,#20373,.F.);
#28055=ORIENTED_EDGE('',*,*,#20375,.F.);
#28056=ORIENTED_EDGE('',*,*,#20363,.T.);
#28057=ORIENTED_EDGE('',*,*,#20376,.T.);
#28058=ORIENTED_EDGE('',*,*,#20377,.T.);
#28059=ORIENTED_EDGE('',*,*,#20376,.F.);
#28060=ORIENTED_EDGE('',*,*,#20378,.F.);
#28061=ORIENTED_EDGE('',*,*,#20379,.T.);
#28062=ORIENTED_EDGE('',*,*,#20377,.F.);
#28063=ORIENTED_EDGE('',*,*,#20379,.F.);
#28064=ORIENTED_EDGE('',*,*,#20380,.T.);
#28065=ORIENTED_EDGE('',*,*,#20381,.T.);
#28066=ORIENTED_EDGE('',*,*,#20378,.T.);
#28067=ORIENTED_EDGE('',*,*,#20381,.F.);
#28068=ORIENTED_EDGE('',*,*,#20354,.F.);
#28069=ORIENTED_EDGE('',*,*,#20275,.F.);
#28070=ORIENTED_EDGE('',*,*,#20280,.F.);
#28071=ORIENTED_EDGE('',*,*,#20382,.F.);
#28072=ORIENTED_EDGE('',*,*,#20340,.F.);
#28073=ORIENTED_EDGE('',*,*,#20345,.F.);
#28074=ORIENTED_EDGE('',*,*,#20348,.F.);
#28075=ORIENTED_EDGE('',*,*,#20351,.F.);
#28076=ORIENTED_EDGE('',*,*,#20383,.F.);
#28077=ORIENTED_EDGE('',*,*,#20384,.F.);
#28078=ORIENTED_EDGE('',*,*,#20385,.F.);
#28079=ORIENTED_EDGE('',*,*,#20386,.F.);
#28080=ORIENTED_EDGE('',*,*,#20380,.F.);
#28081=ORIENTED_EDGE('',*,*,#20383,.T.);
#28082=ORIENTED_EDGE('',*,*,#20387,.T.);
#28083=ORIENTED_EDGE('',*,*,#20374,.T.);
#28084=ORIENTED_EDGE('',*,*,#20387,.F.);
#28085=ORIENTED_EDGE('',*,*,#20386,.T.);
#28086=ORIENTED_EDGE('',*,*,#20388,.T.);
#28087=ORIENTED_EDGE('',*,*,#20370,.T.);
#28088=ORIENTED_EDGE('',*,*,#20388,.F.);
#28089=ORIENTED_EDGE('',*,*,#20384,.T.);
#28090=ORIENTED_EDGE('',*,*,#20389,.T.);
#28091=ORIENTED_EDGE('',*,*,#20366,.T.);
#28092=ORIENTED_EDGE('',*,*,#20389,.F.);
#28093=ORIENTED_EDGE('',*,*,#20293,.F.);
#28094=ORIENTED_EDGE('',*,*,#20341,.F.);
#28095=ORIENTED_EDGE('',*,*,#20382,.T.);
#28096=ORIENTED_EDGE('',*,*,#20279,.T.);
#28097=ORIENTED_EDGE('',*,*,#20286,.F.);
#28098=ORIENTED_EDGE('',*,*,#20390,.T.);
#28099=ORIENTED_EDGE('',*,*,#20276,.F.);
#28100=ORIENTED_EDGE('',*,*,#20353,.F.);
#28101=ORIENTED_EDGE('',*,*,#20357,.F.);
#28102=ORIENTED_EDGE('',*,*,#20270,.F.);
#28103=ORIENTED_EDGE('',*,*,#20273,.T.);
#28104=ORIENTED_EDGE('',*,*,#20356,.F.);
#28105=ORIENTED_EDGE('',*,*,#20338,.F.);
#28106=ORIENTED_EDGE('',*,*,#20361,.T.);
#28107=ORIENTED_EDGE('',*,*,#20287,.F.);
#28108=ORIENTED_EDGE('',*,*,#20303,.F.);
#28109=ORIENTED_EDGE('',*,*,#20342,.F.);
#28110=ORIENTED_EDGE('',*,*,#20295,.F.);
#28111=ORIENTED_EDGE('',*,*,#20307,.F.);
#28112=ORIENTED_EDGE('',*,*,#20294,.F.);
#28113=ORIENTED_EDGE('',*,*,#20390,.F.);
#28114=ORIENTED_EDGE('',*,*,#20285,.F.);
#28115=ORIENTED_EDGE('',*,*,#20298,.F.);
#28116=ORIENTED_EDGE('',*,*,#20266,.F.);
#28117=ORIENTED_EDGE('',*,*,#20289,.F.);
#28118=ORIENTED_EDGE('',*,*,#20284,.F.);
#28119=ORIENTED_EDGE('',*,*,#20277,.F.);
#28120=ORIENTED_EDGE('',*,*,#20391,.T.);
#28121=ORIENTED_EDGE('',*,*,#20392,.T.);
#28122=ORIENTED_EDGE('',*,*,#20393,.T.);
#28123=ORIENTED_EDGE('',*,*,#20394,.T.);
#28124=ORIENTED_EDGE('',*,*,#20395,.T.);
#28125=ORIENTED_EDGE('',*,*,#20393,.F.);
#28126=ORIENTED_EDGE('',*,*,#20394,.F.);
#28127=ORIENTED_EDGE('',*,*,#20395,.F.);
#28128=ORIENTED_EDGE('',*,*,#20396,.T.);
#28129=ORIENTED_EDGE('',*,*,#20397,.F.);
#28130=ORIENTED_EDGE('',*,*,#20398,.F.);
#28131=ORIENTED_EDGE('',*,*,#20396,.F.);
#28132=ORIENTED_EDGE('',*,*,#20385,.T.);
#28133=ORIENTED_EDGE('',*,*,#20399,.T.);
#28134=ORIENTED_EDGE('',*,*,#20391,.F.);
#28135=ORIENTED_EDGE('',*,*,#20392,.F.);
#28136=ORIENTED_EDGE('',*,*,#20399,.F.);
#28137=ORIENTED_EDGE('',*,*,#20397,.T.);
#28138=ORIENTED_EDGE('',*,*,#20398,.T.);
#28139=ORIENTED_EDGE('',*,*,#20400,.T.);
#28140=ORIENTED_EDGE('',*,*,#20401,.T.);
#28141=ORIENTED_EDGE('',*,*,#20400,.F.);
#28142=ORIENTED_EDGE('',*,*,#20401,.F.);
#28143=ORIENTED_EDGE('',*,*,#20402,.F.);
#28144=ORIENTED_EDGE('',*,*,#20403,.T.);
#28145=ORIENTED_EDGE('',*,*,#20404,.F.);
#28146=ORIENTED_EDGE('',*,*,#20405,.F.);
#28147=ORIENTED_EDGE('',*,*,#20406,.F.);
#28148=ORIENTED_EDGE('',*,*,#20407,.F.);
#28149=ORIENTED_EDGE('',*,*,#20408,.F.);
#28150=ORIENTED_EDGE('',*,*,#20409,.F.);
#28151=ORIENTED_EDGE('',*,*,#20410,.F.);
#28152=ORIENTED_EDGE('',*,*,#20411,.F.);
#28153=ORIENTED_EDGE('',*,*,#20412,.F.);
#28154=ORIENTED_EDGE('',*,*,#20413,.F.);
#28155=ORIENTED_EDGE('',*,*,#20414,.F.);
#28156=ORIENTED_EDGE('',*,*,#20415,.T.);
#28157=ORIENTED_EDGE('',*,*,#20252,.T.);
#28158=ORIENTED_EDGE('',*,*,#20249,.T.);
#28159=ORIENTED_EDGE('',*,*,#20246,.T.);
#28160=ORIENTED_EDGE('',*,*,#20416,.F.);
#28161=ORIENTED_EDGE('',*,*,#20417,.F.);
#28162=ORIENTED_EDGE('',*,*,#20418,.F.);
#28163=ORIENTED_EDGE('',*,*,#20419,.F.);
#28164=ORIENTED_EDGE('',*,*,#20420,.F.);
#28165=ORIENTED_EDGE('',*,*,#20421,.T.);
#28166=ORIENTED_EDGE('',*,*,#20242,.T.);
#28167=ORIENTED_EDGE('',*,*,#20239,.T.);
#28168=ORIENTED_EDGE('',*,*,#20236,.T.);
#28169=ORIENTED_EDGE('',*,*,#20233,.T.);
#28170=ORIENTED_EDGE('',*,*,#20230,.T.);
#28171=ORIENTED_EDGE('',*,*,#20227,.T.);
#28172=ORIENTED_EDGE('',*,*,#20422,.F.);
#28173=ORIENTED_EDGE('',*,*,#20423,.F.);
#28174=ORIENTED_EDGE('',*,*,#20424,.F.);
#28175=ORIENTED_EDGE('',*,*,#20425,.F.);
#28176=ORIENTED_EDGE('',*,*,#20426,.F.);
#28177=ORIENTED_EDGE('',*,*,#20427,.F.);
#28178=ORIENTED_EDGE('',*,*,#20428,.F.);
#28179=ORIENTED_EDGE('',*,*,#20429,.F.);
#28180=ORIENTED_EDGE('',*,*,#20430,.F.);
#28181=ORIENTED_EDGE('',*,*,#20431,.F.);
#28182=ORIENTED_EDGE('',*,*,#20432,.F.);
#28183=ORIENTED_EDGE('',*,*,#20433,.F.);
#28184=ORIENTED_EDGE('',*,*,#20434,.F.);
#28185=ORIENTED_EDGE('',*,*,#20435,.F.);
#28186=ORIENTED_EDGE('',*,*,#20436,.F.);
#28187=ORIENTED_EDGE('',*,*,#20437,.F.);
#28188=ORIENTED_EDGE('',*,*,#20224,.T.);
#28189=ORIENTED_EDGE('',*,*,#20438,.F.);
#28190=ORIENTED_EDGE('',*,*,#20439,.F.);
#28191=ORIENTED_EDGE('',*,*,#20440,.F.);
#28192=ORIENTED_EDGE('',*,*,#20441,.T.);
#28193=ORIENTED_EDGE('',*,*,#20442,.F.);
#28194=ORIENTED_EDGE('',*,*,#20443,.T.);
#28195=ORIENTED_EDGE('',*,*,#20444,.F.);
#28196=ORIENTED_EDGE('',*,*,#20445,.F.);
#28197=ORIENTED_EDGE('',*,*,#20446,.F.);
#28198=ORIENTED_EDGE('',*,*,#20447,.F.);
#28199=ORIENTED_EDGE('',*,*,#20448,.F.);
#28200=ORIENTED_EDGE('',*,*,#20244,.F.);
#28201=ORIENTED_EDGE('',*,*,#20248,.F.);
#28202=ORIENTED_EDGE('',*,*,#20251,.F.);
#28203=ORIENTED_EDGE('',*,*,#20449,.F.);
#28204=ORIENTED_EDGE('',*,*,#20450,.F.);
#28205=ORIENTED_EDGE('',*,*,#20451,.F.);
#28206=ORIENTED_EDGE('',*,*,#20452,.F.);
#28207=ORIENTED_EDGE('',*,*,#20453,.F.);
#28208=ORIENTED_EDGE('',*,*,#20454,.F.);
#28209=ORIENTED_EDGE('',*,*,#20455,.F.);
#28210=ORIENTED_EDGE('',*,*,#20456,.F.);
#28211=ORIENTED_EDGE('',*,*,#20457,.F.);
#28212=ORIENTED_EDGE('',*,*,#20458,.F.);
#28213=ORIENTED_EDGE('',*,*,#20459,.F.);
#28214=ORIENTED_EDGE('',*,*,#20460,.F.);
#28215=ORIENTED_EDGE('',*,*,#20461,.F.);
#28216=ORIENTED_EDGE('',*,*,#20462,.F.);
#28217=ORIENTED_EDGE('',*,*,#20463,.F.);
#28218=ORIENTED_EDGE('',*,*,#20464,.F.);
#28219=ORIENTED_EDGE('',*,*,#20465,.F.);
#28220=ORIENTED_EDGE('',*,*,#20466,.F.);
#28221=ORIENTED_EDGE('',*,*,#20467,.F.);
#28222=ORIENTED_EDGE('',*,*,#20468,.F.);
#28223=ORIENTED_EDGE('',*,*,#20469,.F.);
#28224=ORIENTED_EDGE('',*,*,#20470,.F.);
#28225=ORIENTED_EDGE('',*,*,#20471,.F.);
#28226=ORIENTED_EDGE('',*,*,#20472,.F.);
#28227=ORIENTED_EDGE('',*,*,#20473,.F.);
#28228=ORIENTED_EDGE('',*,*,#20474,.F.);
#28229=ORIENTED_EDGE('',*,*,#20475,.F.);
#28230=ORIENTED_EDGE('',*,*,#20476,.F.);
#28231=ORIENTED_EDGE('',*,*,#20222,.F.);
#28232=ORIENTED_EDGE('',*,*,#20229,.F.);
#28233=ORIENTED_EDGE('',*,*,#20232,.F.);
#28234=ORIENTED_EDGE('',*,*,#20235,.F.);
#28235=ORIENTED_EDGE('',*,*,#20238,.F.);
#28236=ORIENTED_EDGE('',*,*,#20241,.F.);
#28237=ORIENTED_EDGE('',*,*,#20477,.F.);
#28238=ORIENTED_EDGE('',*,*,#20478,.F.);
#28239=ORIENTED_EDGE('',*,*,#20479,.F.);
#28240=ORIENTED_EDGE('',*,*,#20480,.F.);
#28241=ORIENTED_EDGE('',*,*,#20481,.F.);
#28242=ORIENTED_EDGE('',*,*,#20482,.F.);
#28243=ORIENTED_EDGE('',*,*,#20483,.F.);
#28244=ORIENTED_EDGE('',*,*,#20250,.T.);
#28245=ORIENTED_EDGE('',*,*,#20415,.F.);
#28246=ORIENTED_EDGE('',*,*,#20484,.F.);
#28247=ORIENTED_EDGE('',*,*,#20459,.T.);
#28248=ORIENTED_EDGE('',*,*,#20485,.F.);
#28249=ORIENTED_EDGE('',*,*,#20449,.T.);
#28250=ORIENTED_EDGE('',*,*,#20240,.T.);
#28251=ORIENTED_EDGE('',*,*,#20421,.F.);
#28252=ORIENTED_EDGE('',*,*,#20486,.F.);
#28253=ORIENTED_EDGE('',*,*,#20477,.T.);
#28254=ORIENTED_EDGE('',*,*,#20487,.F.);
#28255=ORIENTED_EDGE('',*,*,#20463,.T.);
#28256=ORIENTED_EDGE('',*,*,#20488,.F.);
#28257=ORIENTED_EDGE('',*,*,#20403,.F.);
#28258=ORIENTED_EDGE('',*,*,#20489,.F.);
#28259=ORIENTED_EDGE('',*,*,#20441,.F.);
#28260=ORIENTED_EDGE('',*,*,#20490,.F.);
#28261=ORIENTED_EDGE('',*,*,#20481,.T.);
#28262=ORIENTED_EDGE('',*,*,#20491,.F.);
#28263=ORIENTED_EDGE('',*,*,#20492,.T.);
#28264=ORIENTED_EDGE('',*,*,#20493,.F.);
#28265=ORIENTED_EDGE('',*,*,#20443,.F.);
#28266=ORIENTED_EDGE('',*,*,#20245,.T.);
#28267=ORIENTED_EDGE('',*,*,#20448,.T.);
#28268=ORIENTED_EDGE('',*,*,#20494,.F.);
#28269=ORIENTED_EDGE('',*,*,#20495,.F.);
#28270=ORIENTED_EDGE('',*,*,#20416,.T.);
#28271=ORIENTED_EDGE('',*,*,#20496,.F.);
#28272=ORIENTED_EDGE('',*,*,#20497,.T.);
#28273=ORIENTED_EDGE('',*,*,#20478,.T.);
#28274=ORIENTED_EDGE('',*,*,#20486,.T.);
#28275=ORIENTED_EDGE('',*,*,#20420,.T.);
#28276=ORIENTED_EDGE('',*,*,#20498,.T.);
#28277=ORIENTED_EDGE('',*,*,#20499,.T.);
#28278=ORIENTED_EDGE('',*,*,#20500,.F.);
#28279=ORIENTED_EDGE('',*,*,#20501,.F.);
#28280=ORIENTED_EDGE('',*,*,#20502,.F.);
#28281=ORIENTED_EDGE('',*,*,#20492,.F.);
#28282=ORIENTED_EDGE('',*,*,#20423,.T.);
#28283=ORIENTED_EDGE('',*,*,#20503,.F.);
#28284=ORIENTED_EDGE('',*,*,#20504,.F.);
#28285=ORIENTED_EDGE('',*,*,#20474,.T.);
#28286=ORIENTED_EDGE('',*,*,#20505,.F.);
#28287=ORIENTED_EDGE('',*,*,#20425,.T.);
#28288=ORIENTED_EDGE('',*,*,#20506,.F.);
#28289=ORIENTED_EDGE('',*,*,#20427,.T.);
#28290=ORIENTED_EDGE('',*,*,#20507,.F.);
#28291=ORIENTED_EDGE('',*,*,#20472,.T.);
#28292=ORIENTED_EDGE('',*,*,#20508,.F.);
#28293=ORIENTED_EDGE('',*,*,#20429,.T.);
#28294=ORIENTED_EDGE('',*,*,#20509,.F.);
#28295=ORIENTED_EDGE('',*,*,#20470,.T.);
#28296=ORIENTED_EDGE('',*,*,#20510,.F.);
#28297=ORIENTED_EDGE('',*,*,#20431,.T.);
#28298=ORIENTED_EDGE('',*,*,#20511,.F.);
#28299=ORIENTED_EDGE('',*,*,#20468,.T.);
#28300=ORIENTED_EDGE('',*,*,#20512,.F.);
#28301=ORIENTED_EDGE('',*,*,#20433,.T.);
#28302=ORIENTED_EDGE('',*,*,#20513,.F.);
#28303=ORIENTED_EDGE('',*,*,#20466,.T.);
#28304=ORIENTED_EDGE('',*,*,#20514,.F.);
#28305=ORIENTED_EDGE('',*,*,#20418,.T.);
#28306=ORIENTED_EDGE('',*,*,#20515,.F.);
#28307=ORIENTED_EDGE('',*,*,#20464,.T.);
#28308=ORIENTED_EDGE('',*,*,#20516,.F.);
#28309=ORIENTED_EDGE('',*,*,#20454,.T.);
#28310=ORIENTED_EDGE('',*,*,#20517,.F.);
#28311=ORIENTED_EDGE('',*,*,#20411,.T.);
#28312=ORIENTED_EDGE('',*,*,#20518,.F.);
#28313=ORIENTED_EDGE('',*,*,#20446,.T.);
#28314=ORIENTED_EDGE('',*,*,#20519,.F.);
#28315=ORIENTED_EDGE('',*,*,#20409,.T.);
#28316=ORIENTED_EDGE('',*,*,#20520,.F.);
#28317=ORIENTED_EDGE('',*,*,#20407,.T.);
#28318=ORIENTED_EDGE('',*,*,#20521,.F.);
#28319=ORIENTED_EDGE('',*,*,#20522,.F.);
#28320=ORIENTED_EDGE('',*,*,#20523,.F.);
#28321=ORIENTED_EDGE('',*,*,#20405,.T.);
#28322=ORIENTED_EDGE('',*,*,#20524,.F.);
#28323=ORIENTED_EDGE('',*,*,#20413,.T.);
#28324=ORIENTED_EDGE('',*,*,#20525,.F.);
#28325=ORIENTED_EDGE('',*,*,#20452,.T.);
#28326=ORIENTED_EDGE('',*,*,#20526,.F.);
#28327=ORIENTED_EDGE('',*,*,#20453,.T.);
#28328=ORIENTED_EDGE('',*,*,#20525,.T.);
#28329=ORIENTED_EDGE('',*,*,#20412,.T.);
#28330=ORIENTED_EDGE('',*,*,#20517,.T.);
#28331=ORIENTED_EDGE('',*,*,#20406,.T.);
#28332=ORIENTED_EDGE('',*,*,#20526,.T.);
#28333=ORIENTED_EDGE('',*,*,#20451,.T.);
#28334=ORIENTED_EDGE('',*,*,#20527,.T.);
#28335=ORIENTED_EDGE('',*,*,#20455,.T.);
#28336=ORIENTED_EDGE('',*,*,#20518,.T.);
#28337=ORIENTED_EDGE('',*,*,#20410,.T.);
#28338=ORIENTED_EDGE('',*,*,#20519,.T.);
#28339=ORIENTED_EDGE('',*,*,#20447,.T.);
#28340=ORIENTED_EDGE('',*,*,#20520,.T.);
#28341=ORIENTED_EDGE('',*,*,#20408,.T.);
#28342=ORIENTED_EDGE('',*,*,#20523,.T.);
#28343=ORIENTED_EDGE('',*,*,#20528,.F.);
#28344=ORIENTED_EDGE('',*,*,#20417,.T.);
#28345=ORIENTED_EDGE('',*,*,#20529,.F.);
#28346=ORIENTED_EDGE('',*,*,#20521,.T.);
#28347=ORIENTED_EDGE('',*,*,#20445,.T.);
#28348=ORIENTED_EDGE('',*,*,#20530,.T.);
#28349=ORIENTED_EDGE('',*,*,#20457,.T.);
#28350=ORIENTED_EDGE('',*,*,#20531,.T.);
#28351=ORIENTED_EDGE('',*,*,#20426,.T.);
#28352=ORIENTED_EDGE('',*,*,#20505,.T.);
#28353=ORIENTED_EDGE('',*,*,#20473,.T.);
#28354=ORIENTED_EDGE('',*,*,#20507,.T.);
#28355=ORIENTED_EDGE('',*,*,#20428,.T.);
#28356=ORIENTED_EDGE('',*,*,#20508,.T.);
#28357=ORIENTED_EDGE('',*,*,#20471,.T.);
#28358=ORIENTED_EDGE('',*,*,#20509,.T.);
#28359=ORIENTED_EDGE('',*,*,#20430,.T.);
#28360=ORIENTED_EDGE('',*,*,#20510,.T.);
#28361=ORIENTED_EDGE('',*,*,#20469,.T.);
#28362=ORIENTED_EDGE('',*,*,#20511,.T.);
#28363=ORIENTED_EDGE('',*,*,#20432,.T.);
#28364=ORIENTED_EDGE('',*,*,#20512,.T.);
#28365=ORIENTED_EDGE('',*,*,#20467,.T.);
#28366=ORIENTED_EDGE('',*,*,#20513,.T.);
#28367=ORIENTED_EDGE('',*,*,#20434,.T.);
#28368=ORIENTED_EDGE('',*,*,#20514,.T.);
#28369=ORIENTED_EDGE('',*,*,#20465,.T.);
#28370=ORIENTED_EDGE('',*,*,#20515,.T.);
#28371=ORIENTED_EDGE('',*,*,#20419,.T.);
#28372=ORIENTED_EDGE('',*,*,#20516,.T.);
#28373=ORIENTED_EDGE('',*,*,#20479,.T.);
#28374=ORIENTED_EDGE('',*,*,#20532,.T.);
#28375=ORIENTED_EDGE('',*,*,#20483,.T.);
#28376=ORIENTED_EDGE('',*,*,#20533,.T.);
#28377=ORIENTED_EDGE('',*,*,#20534,.T.);
#28378=ORIENTED_EDGE('',*,*,#20475,.T.);
#28379=ORIENTED_EDGE('',*,*,#20506,.T.);
#28380=ORIENTED_EDGE('',*,*,#20424,.T.);
#28381=ORIENTED_EDGE('',*,*,#20504,.T.);
#28382=ORIENTED_EDGE('',*,*,#20535,.T.);
#28383=ORIENTED_EDGE('',*,*,#20439,.T.);
#28384=ORIENTED_EDGE('',*,*,#20536,.T.);
#28385=ORIENTED_EDGE('',*,*,#20461,.T.);
#28386=ORIENTED_EDGE('',*,*,#20537,.T.);
#28387=ORIENTED_EDGE('',*,*,#20502,.T.);
#28388=ORIENTED_EDGE('',*,*,#20538,.F.);
#28389=ORIENTED_EDGE('',*,*,#20435,.T.);
#28390=ORIENTED_EDGE('',*,*,#20223,.T.);
#28391=ORIENTED_EDGE('',*,*,#20476,.T.);
#28392=ORIENTED_EDGE('',*,*,#20534,.F.);
#28393=ORIENTED_EDGE('',*,*,#20539,.T.);
#28394=ORIENTED_EDGE('',*,*,#20225,.T.);
#28395=ORIENTED_EDGE('',*,*,#20437,.T.);
#28396=ORIENTED_EDGE('',*,*,#20540,.F.);
#28397=ORIENTED_EDGE('',*,*,#20500,.T.);
#28398=ORIENTED_EDGE('',*,*,#20491,.T.);
#28399=ORIENTED_EDGE('',*,*,#20442,.T.);
#28400=ORIENTED_EDGE('',*,*,#20531,.F.);
#28401=ORIENTED_EDGE('',*,*,#20456,.T.);
#28402=ORIENTED_EDGE('',*,*,#20484,.T.);
#28403=ORIENTED_EDGE('',*,*,#20414,.T.);
#28404=ORIENTED_EDGE('',*,*,#20524,.T.);
#28405=ORIENTED_EDGE('',*,*,#20404,.T.);
#28406=ORIENTED_EDGE('',*,*,#20488,.T.);
#28407=ORIENTED_EDGE('',*,*,#20462,.T.);
#28408=ORIENTED_EDGE('',*,*,#20536,.F.);
#28409=ORIENTED_EDGE('',*,*,#20438,.T.);
#28410=ORIENTED_EDGE('',*,*,#20489,.T.);
#28411=ORIENTED_EDGE('',*,*,#20480,.T.);
#28412=ORIENTED_EDGE('',*,*,#20535,.F.);
#28413=ORIENTED_EDGE('',*,*,#20503,.T.);
#28414=ORIENTED_EDGE('',*,*,#20422,.T.);
#28415=ORIENTED_EDGE('',*,*,#20226,.T.);
#28416=ORIENTED_EDGE('',*,*,#20539,.F.);
#28417=ORIENTED_EDGE('',*,*,#20533,.F.);
#28418=ORIENTED_EDGE('',*,*,#20482,.T.);
#28419=ORIENTED_EDGE('',*,*,#20490,.T.);
#28420=ORIENTED_EDGE('',*,*,#20440,.T.);
#28421=ORIENTED_EDGE('',*,*,#20537,.F.);
#28422=ORIENTED_EDGE('',*,*,#20460,.T.);
#28423=ORIENTED_EDGE('',*,*,#20487,.T.);
#28424=ORIENTED_EDGE('',*,*,#20402,.T.);
#28425=ORIENTED_EDGE('',*,*,#20527,.F.);
#28426=ORIENTED_EDGE('',*,*,#20450,.T.);
#28427=ORIENTED_EDGE('',*,*,#20485,.T.);
#28428=ORIENTED_EDGE('',*,*,#20458,.T.);
#28429=ORIENTED_EDGE('',*,*,#20530,.F.);
#28430=ORIENTED_EDGE('',*,*,#20444,.T.);
#28431=ORIENTED_EDGE('',*,*,#20493,.T.);
#28432=ORIENTED_EDGE('',*,*,#20541,.F.);
#28433=ORIENTED_EDGE('',*,*,#20542,.T.);
#28434=ORIENTED_EDGE('',*,*,#20364,.T.);
#28435=ORIENTED_EDGE('',*,*,#20542,.F.);
#28436=ORIENTED_EDGE('',*,*,#20543,.F.);
#28437=ORIENTED_EDGE('',*,*,#20544,.T.);
#28438=ORIENTED_EDGE('',*,*,#20541,.T.);
#28439=ORIENTED_EDGE('',*,*,#20544,.F.);
#28440=ORIENTED_EDGE('',*,*,#20543,.T.);
#28441=ORIENTED_EDGE('',*,*,#20545,.F.);
#28442=ORIENTED_EDGE('',*,*,#20546,.F.);
#28443=ORIENTED_EDGE('',*,*,#20547,.T.);
#28444=ORIENTED_EDGE('',*,*,#20545,.T.);
#28445=ORIENTED_EDGE('',*,*,#20547,.F.);
#28446=ORIENTED_EDGE('',*,*,#20548,.F.);
#28447=ORIENTED_EDGE('',*,*,#20549,.T.);
#28448=ORIENTED_EDGE('',*,*,#20546,.T.);
#28449=ORIENTED_EDGE('',*,*,#20549,.F.);
#28450=ORIENTED_EDGE('',*,*,#20550,.F.);
#28451=ORIENTED_EDGE('',*,*,#20551,.T.);
#28452=ORIENTED_EDGE('',*,*,#20548,.T.);
#28453=ORIENTED_EDGE('',*,*,#20551,.F.);
#28454=ORIENTED_EDGE('',*,*,#20552,.F.);
#28455=ORIENTED_EDGE('',*,*,#20553,.T.);
#28456=ORIENTED_EDGE('',*,*,#20550,.T.);
#28457=ORIENTED_EDGE('',*,*,#20553,.F.);
#28458=ORIENTED_EDGE('',*,*,#20554,.F.);
#28459=ORIENTED_EDGE('',*,*,#20555,.F.);
#28460=ORIENTED_EDGE('',*,*,#20263,.F.);
#28461=ORIENTED_EDGE('',*,*,#20556,.F.);
#28462=ORIENTED_EDGE('',*,*,#20557,.F.);
#28463=ORIENTED_EDGE('',*,*,#20558,.F.);
#28464=ORIENTED_EDGE('',*,*,#20556,.T.);
#28465=ORIENTED_EDGE('',*,*,#20262,.F.);
#28466=ORIENTED_EDGE('',*,*,#20258,.F.);
#28467=ORIENTED_EDGE('',*,*,#20559,.T.);
#28468=ORIENTED_EDGE('',*,*,#20554,.T.);
#28469=ORIENTED_EDGE('',*,*,#20558,.T.);
#28470=ORIENTED_EDGE('',*,*,#20560,.F.);
#28471=ORIENTED_EDGE('',*,*,#20561,.T.);
#28472=ORIENTED_EDGE('',*,*,#20552,.T.);
#28473=ORIENTED_EDGE('',*,*,#20561,.F.);
#28474=ORIENTED_EDGE('',*,*,#20562,.F.);
#28475=ORIENTED_EDGE('',*,*,#20563,.F.);
#28476=ORIENTED_EDGE('',*,*,#20260,.F.);
#28477=ORIENTED_EDGE('',*,*,#20264,.T.);
#28478=ORIENTED_EDGE('',*,*,#20555,.T.);
#28479=ORIENTED_EDGE('',*,*,#20559,.F.);
#28480=ORIENTED_EDGE('',*,*,#20563,.T.);
#28481=ORIENTED_EDGE('',*,*,#20562,.T.);
#28482=ORIENTED_EDGE('',*,*,#20560,.T.);
#28483=ORIENTED_EDGE('',*,*,#20557,.T.);
#28484=ORIENTED_EDGE('',*,*,#20261,.F.);
#28485=ORIENTED_EDGE('',*,*,#20564,.F.);
#28486=ORIENTED_EDGE('',*,*,#20565,.F.);
#28487=ORIENTED_EDGE('',*,*,#20566,.T.);
#28488=ORIENTED_EDGE('',*,*,#20564,.T.);
#28489=ORIENTED_EDGE('',*,*,#20566,.F.);
#28490=ORIENTED_EDGE('',*,*,#20567,.T.);
#28491=ORIENTED_EDGE('',*,*,#20499,.F.);
#28492=ORIENTED_EDGE('',*,*,#20568,.T.);
#28493=ORIENTED_EDGE('',*,*,#20565,.T.);
#28494=ORIENTED_EDGE('',*,*,#20568,.F.);
#28495=ORIENTED_EDGE('',*,*,#20498,.F.);
#28496=ORIENTED_EDGE('',*,*,#20532,.F.);
#28497=ORIENTED_EDGE('',*,*,#20497,.F.);
#28498=ORIENTED_EDGE('',*,*,#20257,.F.);
#28499=ORIENTED_EDGE('',*,*,#20569,.T.);
#28500=ORIENTED_EDGE('',*,*,#20494,.T.);
#28501=ORIENTED_EDGE('',*,*,#20528,.T.);
#28502=ORIENTED_EDGE('',*,*,#20522,.T.);
#28503=ORIENTED_EDGE('',*,*,#20529,.T.);
#28504=ORIENTED_EDGE('',*,*,#20495,.T.);
#28505=ORIENTED_EDGE('',*,*,#20569,.F.);
#28506=ORIENTED_EDGE('',*,*,#20496,.T.);
#28507=ORIENTED_EDGE('',*,*,#20567,.F.);
#28508=ORIENTED_EDGE('',*,*,#20501,.T.);
#28509=ORIENTED_EDGE('',*,*,#20540,.T.);
#28510=ORIENTED_EDGE('',*,*,#20436,.T.);
#28511=ORIENTED_EDGE('',*,*,#20538,.T.);
#31967=CONICAL_SURFACE('',#36177,3.02920176969664,1.10124348056693);
#31968=CONICAL_SURFACE('',#36180,1.5,0.631690634338971);
#31969=CONICAL_SURFACE('',#36218,7.,0.785398163397446);
#31970=CONICAL_SURFACE('',#36228,7.,0.785398163397446);
#31971=CONICAL_SURFACE('',#36232,7.,0.785398163397446);
#31972=CONICAL_SURFACE('',#36236,7.,0.785398163397446);
#31973=CONICAL_SURFACE('',#36240,7.,0.785398163397448);
#31974=CONICAL_SURFACE('',#36247,7.,0.785398163397448);
#31975=CONICAL_SURFACE('',#36248,7.,0.785398163397448);
#31976=CONICAL_SURFACE('',#36249,7.,0.785398163397448);
#31977=CONICAL_SURFACE('',#36256,25.2232233047034,0.392699081698712);
#31978=CONICAL_SURFACE('',#36261,25.,0.785398163397448);
#31979=CONICAL_SURFACE('',#36265,24.5267766952966,1.17809724509617);
#31980=CONICAL_SURFACE('',#36312,23.61565,1.17289539365476);
#31981=CONICAL_SURFACE('',#36318,17.72,0.785398163397448);
#31982=CONICAL_SURFACE('',#36322,15.72,0.610725964389208);
#31983=CONICAL_SURFACE('',#36324,13.72,0.785398163397451);
#31984=CONICAL_SURFACE('',#36337,12.3,1.01219701145133);
#31985=CONICAL_SURFACE('',#36338,12.35,0.785398163397447);
#33369=ADVANCED_FACE('',(#4395),#3017,.T.);
#33370=ADVANCED_FACE('',(#4396),#3018,.T.);
#33371=ADVANCED_FACE('',(#4397),#3019,.T.);
#33372=ADVANCED_FACE('',(#4398),#3020,.T.);
#33373=ADVANCED_FACE('',(#4399),#3021,.T.);
#33374=ADVANCED_FACE('',(#4400),#3022,.T.);
#33375=ADVANCED_FACE('',(#4401),#3023,.T.);
#33376=ADVANCED_FACE('',(#4402),#3024,.T.);
#33377=ADVANCED_FACE('',(#4403),#3025,.T.);
#33378=ADVANCED_FACE('',(#4404),#31967,.F.);
#33379=ADVANCED_FACE('',(#4405),#31968,.F.);
#33380=ADVANCED_FACE('',(#4406,#1221),#2527,.T.);
#33381=ADVANCED_FACE('',(#4407),#2528,.T.);
#33382=ADVANCED_FACE('',(#4408),#2529,.F.);
#33383=ADVANCED_FACE('',(#4409),#2530,.T.);
#33384=ADVANCED_FACE('',(#4410),#2531,.T.);
#33385=ADVANCED_FACE('',(#4411),#2532,.T.);
#33386=ADVANCED_FACE('',(#4412),#2533,.T.);
#33387=ADVANCED_FACE('',(#4413),#2534,.T.);
#33388=ADVANCED_FACE('',(#4414),#2535,.T.);
#33389=ADVANCED_FACE('',(#4415),#2536,.T.);
#33390=ADVANCED_FACE('',(#4416),#2537,.T.);
#33391=ADVANCED_FACE('',(#4417),#2538,.T.);
#33392=ADVANCED_FACE('',(#4418),#2539,.T.);
#33393=ADVANCED_FACE('',(#4419),#2540,.T.);
#33394=ADVANCED_FACE('',(#4420),#2541,.T.);
#33395=ADVANCED_FACE('',(#4421),#2542,.T.);
#33396=ADVANCED_FACE('',(#4422),#2543,.T.);
#33397=ADVANCED_FACE('',(#4423),#2544,.T.);
#33398=ADVANCED_FACE('',(#4424),#2545,.T.);
#33399=ADVANCED_FACE('',(#4425),#2546,.T.);
#33400=ADVANCED_FACE('',(#4426),#2547,.T.);
#33401=ADVANCED_FACE('',(#4427),#2548,.T.);
#33402=ADVANCED_FACE('',(#4428),#2549,.T.);
#33403=ADVANCED_FACE('',(#4429),#2550,.T.);
#33404=ADVANCED_FACE('',(#4430),#2551,.T.);
#33405=ADVANCED_FACE('',(#4431),#2552,.T.);
#33406=ADVANCED_FACE('',(#4432),#2553,.T.);
#33407=ADVANCED_FACE('',(#4433),#2554,.T.);
#33408=ADVANCED_FACE('',(#4434),#2555,.T.);
#33409=ADVANCED_FACE('',(#4435),#2556,.T.);
#33410=ADVANCED_FACE('',(#4436),#2557,.T.);
#33411=ADVANCED_FACE('',(#4437),#2558,.T.);
#33412=ADVANCED_FACE('',(#4438),#2559,.T.);
#33413=ADVANCED_FACE('',(#4439),#2560,.T.);
#33414=ADVANCED_FACE('',(#4440),#2561,.T.);
#33415=ADVANCED_FACE('',(#4441),#2562,.T.);
#33416=ADVANCED_FACE('',(#4442),#31969,.F.);
#33417=ADVANCED_FACE('',(#4443,#1222,#1223,#1224,#1225,#1226),#2563,.T.);
#33418=ADVANCED_FACE('',(#4444),#3026,.F.);
#33419=ADVANCED_FACE('',(#4445),#31970,.F.);
#33420=ADVANCED_FACE('',(#4446),#3027,.F.);
#33421=ADVANCED_FACE('',(#4447),#31971,.F.);
#33422=ADVANCED_FACE('',(#4448),#3028,.F.);
#33423=ADVANCED_FACE('',(#4449),#31972,.F.);
#33424=ADVANCED_FACE('',(#4450),#3029,.F.);
#33425=ADVANCED_FACE('',(#4451),#31973,.F.);
#33426=ADVANCED_FACE('',(#4452,#1227,#1228,#1229,#1230,#1231),#2564,.F.);
#33427=ADVANCED_FACE('',(#4453),#31974,.F.);
#33428=ADVANCED_FACE('',(#4454),#31975,.F.);
#33429=ADVANCED_FACE('',(#4455),#31976,.F.);
#33430=ADVANCED_FACE('',(#4456),#2565,.T.);
#33431=ADVANCED_FACE('',(#4457),#2566,.T.);
#33432=ADVANCED_FACE('',(#4458),#2567,.T.);
#33433=ADVANCED_FACE('',(#4459),#2568,.T.);
#33434=ADVANCED_FACE('',(#4460),#2569,.T.);
#33435=ADVANCED_FACE('',(#4461),#2570,.T.);
#33436=ADVANCED_FACE('',(#4462),#31977,.T.);
#33437=ADVANCED_FACE('',(#4463),#31978,.T.);
#33438=ADVANCED_FACE('',(#4464),#3030,.T.);
#33439=ADVANCED_FACE('',(#4465),#31979,.T.);
#33440=ADVANCED_FACE('',(#4466),#2571,.T.);
#33441=ADVANCED_FACE('',(#4467),#275,.F.);
#33442=ADVANCED_FACE('',(#4468),#276,.F.);
#33443=ADVANCED_FACE('',(#4469),#277,.F.);
#33444=ADVANCED_FACE('',(#4470),#278,.F.);
#33445=ADVANCED_FACE('',(#4471),#279,.F.);
#33446=ADVANCED_FACE('',(#4472),#280,.F.);
#33447=ADVANCED_FACE('',(#4473),#281,.F.);
#33448=ADVANCED_FACE('',(#4474),#282,.F.);
#33449=ADVANCED_FACE('',(#4475),#283,.F.);
#33450=ADVANCED_FACE('',(#4476),#284,.F.);
#33451=ADVANCED_FACE('',(#4477),#285,.F.);
#33452=ADVANCED_FACE('',(#4478),#3031,.T.);
#33453=ADVANCED_FACE('',(#4479),#3032,.T.);
#33454=ADVANCED_FACE('',(#4480),#3033,.T.);
#33455=ADVANCED_FACE('',(#4481),#3034,.T.);
#33456=ADVANCED_FACE('',(#4482),#3035,.T.);
#33457=ADVANCED_FACE('',(#4483),#2572,.F.);
#33458=ADVANCED_FACE('',(#4484),#2573,.T.);
#33459=ADVANCED_FACE('',(#4485),#286,.F.);
#33460=ADVANCED_FACE('',(#4486),#2574,.F.);
#33461=ADVANCED_FACE('',(#4487),#2575,.F.);
#33462=ADVANCED_FACE('',(#4488),#2576,.F.);
#33463=ADVANCED_FACE('',(#4489),#2577,.F.);
#33464=ADVANCED_FACE('',(#4490),#2578,.F.);
#33465=ADVANCED_FACE('',(#4491),#2579,.F.);
#33466=ADVANCED_FACE('',(#4492),#2580,.F.);
#33467=ADVANCED_FACE('',(#4493),#2581,.F.);
#33468=ADVANCED_FACE('',(#4494),#2582,.F.);
#33469=ADVANCED_FACE('',(#4495),#2583,.F.);
#33470=ADVANCED_FACE('',(#4496),#2584,.F.);
#33471=ADVANCED_FACE('',(#4497),#3036,.T.);
#33472=ADVANCED_FACE('',(#4498),#3037,.T.);
#33473=ADVANCED_FACE('',(#4499),#3038,.T.);
#33474=ADVANCED_FACE('',(#4500),#3039,.T.);
#33475=ADVANCED_FACE('',(#4501),#3040,.T.);
#33476=ADVANCED_FACE('',(#4502),#3041,.T.);
#33477=ADVANCED_FACE('',(#4503),#3042,.T.);
#33478=ADVANCED_FACE('',(#4504),#3043,.T.);
#33479=ADVANCED_FACE('',(#4505),#3044,.T.);
#33480=ADVANCED_FACE('',(#4506),#3045,.T.);
#33481=ADVANCED_FACE('',(#4507),#3046,.T.);
#33482=ADVANCED_FACE('',(#4508),#3047,.T.);
#33483=ADVANCED_FACE('',(#4509),#3048,.T.);
#33484=ADVANCED_FACE('',(#4510),#3049,.T.);
#33485=ADVANCED_FACE('',(#4511),#3050,.F.);
#33486=ADVANCED_FACE('',(#4512),#31980,.T.);
#33487=ADVANCED_FACE('',(#4513),#3051,.T.);
#33488=ADVANCED_FACE('',(#4514,#1232),#2585,.T.);
#33489=ADVANCED_FACE('',(#4515),#31981,.T.);
#33490=ADVANCED_FACE('',(#4516),#3052,.T.);
#33491=ADVANCED_FACE('',(#4517),#31982,.T.);
#33492=ADVANCED_FACE('',(#4518),#31983,.T.);
#33493=ADVANCED_FACE('',(#4519),#2586,.F.);
#33494=ADVANCED_FACE('',(#4520),#2587,.F.);
#33495=ADVANCED_FACE('',(#4521),#3053,.T.);
#33496=ADVANCED_FACE('',(#4522),#2588,.F.);
#33497=ADVANCED_FACE('',(#4523,#1233),#2589,.T.);
#33498=ADVANCED_FACE('',(#4524),#3054,.T.);
#33499=ADVANCED_FACE('',(#4525),#31984,.T.);
#33500=ADVANCED_FACE('',(#4526),#31985,.T.);
#33501=ADVANCED_FACE('',(#4527),#2590,.F.);
#33502=ADVANCED_FACE('',(#4528),#3055,.T.);
#34209=CLOSED_SHELL('',(#33369,#33370,#33371,#33372,#33373,#33374,#33375,
#33376,#33377,#33378,#33379,#33380,#33381,#33382,#33383,#33384,#33385,#33386,
#33387,#33388,#33389,#33390,#33391,#33392,#33393,#33394,#33395,#33396,#33397,
#33398,#33399,#33400,#33401,#33402,#33403,#33404,#33405,#33406,#33407,#33408,
#33409,#33410,#33411,#33412,#33413,#33414,#33415,#33416,#33417,#33418,#33419,
#33420,#33421,#33422,#33423,#33424,#33425,#33426,#33427,#33428,#33429,#33430,
#33431,#33432,#33433,#33434,#33435,#33436,#33437,#33438,#33439,#33440,#33441,
#33442,#33443,#33444,#33445,#33446,#33447,#33448,#33449,#33450,#33451,#33452,
#33453,#33454,#33455,#33456,#33457,#33458,#33459,#33460,#33461,#33462,#33463,
#33464,#33465,#33466,#33467,#33468,#33469,#33470,#33471,#33472,#33473,#33474,
#33475,#33476,#33477,#33478,#33479,#33480,#33481,#33482,#33483,#33484,#33485,
#33486,#33487,#33488,#33489,#33490,#33491,#33492,#33493,#33494,#33495,#33496,
#33497,#33498,#33499,#33500,#33501,#33502));
#36166=AXIS2_PLACEMENT_3D('',#52952,#43478,#43479);
#36167=AXIS2_PLACEMENT_3D('',#52953,#43480,#43481);
#36168=AXIS2_PLACEMENT_3D('',#53007,#43483,#43484);
#36169=AXIS2_PLACEMENT_3D('',#53044,#43486,#43487);
#36170=AXIS2_PLACEMENT_3D('',#53082,#43489,#43490);
#36171=AXIS2_PLACEMENT_3D('',#53120,#43492,#43493);
#36172=AXIS2_PLACEMENT_3D('',#53157,#43495,#43496);
#36173=AXIS2_PLACEMENT_3D('',#53194,#43498,#43499);
#36174=AXIS2_PLACEMENT_3D('',#53215,#43501,#43502);
#36175=AXIS2_PLACEMENT_3D('',#53228,#43503,#43504);
#36176=AXIS2_PLACEMENT_3D('',#53266,#43506,#43507);
#36177=AXIS2_PLACEMENT_3D('',#53303,#43509,#43510);
#36178=AXIS2_PLACEMENT_3D('',#53305,#43511,#43512);
#36179=AXIS2_PLACEMENT_3D('',#53308,#43514,#43515);
#36180=AXIS2_PLACEMENT_3D('',#53309,#43516,#43517);
#36181=AXIS2_PLACEMENT_3D('',#53312,#43519,#43520);
#36182=AXIS2_PLACEMENT_3D('',#53314,#43521,#43522);
#36183=AXIS2_PLACEMENT_3D('',#53315,#43523,#43524);
#36184=AXIS2_PLACEMENT_3D('',#53324,#43529,#43530);
#36185=AXIS2_PLACEMENT_3D('',#53330,#43534,#43535);
#36186=AXIS2_PLACEMENT_3D('',#53343,#43542,#43543);
#36187=AXIS2_PLACEMENT_3D('',#53349,#43547,#43548);
#36188=AXIS2_PLACEMENT_3D('',#53355,#43552,#43553);
#36189=AXIS2_PLACEMENT_3D('',#53363,#43558,#43559);
#36190=AXIS2_PLACEMENT_3D('',#53370,#43563,#43564);
#36191=AXIS2_PLACEMENT_3D('',#53375,#43568,#43569);
#36192=AXIS2_PLACEMENT_3D('',#53380,#43573,#43574);
#36193=AXIS2_PLACEMENT_3D('',#53387,#43578,#43579);
#36194=AXIS2_PLACEMENT_3D('',#53395,#43584,#43585);
#36195=AXIS2_PLACEMENT_3D('',#53398,#43588,#43589);
#36196=AXIS2_PLACEMENT_3D('',#53405,#43593,#43594);
#36197=AXIS2_PLACEMENT_3D('',#53413,#43599,#43600);
#36198=AXIS2_PLACEMENT_3D('',#53416,#43603,#43604);
#36199=AXIS2_PLACEMENT_3D('',#53423,#43608,#43609);
#36200=AXIS2_PLACEMENT_3D('',#53431,#43614,#43615);
#36201=AXIS2_PLACEMENT_3D('',#53434,#43618,#43619);
#36202=AXIS2_PLACEMENT_3D('',#53441,#43623,#43624);
#36203=AXIS2_PLACEMENT_3D('',#53449,#43629,#43630);
#36204=AXIS2_PLACEMENT_3D('',#53452,#43633,#43634);
#36205=AXIS2_PLACEMENT_3D('',#53459,#43638,#43639);
#36206=AXIS2_PLACEMENT_3D('',#53467,#43644,#43645);
#36207=AXIS2_PLACEMENT_3D('',#53470,#43648,#43649);
#36208=AXIS2_PLACEMENT_3D('',#53478,#43654,#43655);
#36209=AXIS2_PLACEMENT_3D('',#53485,#43660,#43661);
#36210=AXIS2_PLACEMENT_3D('',#53487,#43663,#43664);
#36211=AXIS2_PLACEMENT_3D('',#53491,#43667,#43668);
#36212=AXIS2_PLACEMENT_3D('',#53493,#43670,#43671);
#36213=AXIS2_PLACEMENT_3D('',#53497,#43674,#43675);
#36214=AXIS2_PLACEMENT_3D('',#53499,#43677,#43678);
#36215=AXIS2_PLACEMENT_3D('',#53503,#43681,#43682);
#36216=AXIS2_PLACEMENT_3D('',#53508,#43686,#43687);
#36217=AXIS2_PLACEMENT_3D('',#53510,#43689,#43690);
#36218=AXIS2_PLACEMENT_3D('',#53513,#43693,#43694);
#36219=AXIS2_PLACEMENT_3D('',#53515,#43695,#43696);
#36220=AXIS2_PLACEMENT_3D('',#53518,#43698,#43699);
#36221=AXIS2_PLACEMENT_3D('',#53519,#43700,#43701);
#36222=AXIS2_PLACEMENT_3D('',#53522,#43703,#43704);
#36223=AXIS2_PLACEMENT_3D('',#53524,#43705,#43706);
#36224=AXIS2_PLACEMENT_3D('',#53526,#43707,#43708);
#36225=AXIS2_PLACEMENT_3D('',#53528,#43709,#43710);
#36226=AXIS2_PLACEMENT_3D('',#53529,#43711,#43712);
#36227=AXIS2_PLACEMENT_3D('',#53531,#43713,#43714);
#36228=AXIS2_PLACEMENT_3D('',#53533,#43716,#43717);
#36229=AXIS2_PLACEMENT_3D('',#53536,#43719,#43720);
#36230=AXIS2_PLACEMENT_3D('',#53537,#43721,#43722);
#36231=AXIS2_PLACEMENT_3D('',#53539,#43723,#43724);
#36232=AXIS2_PLACEMENT_3D('',#53541,#43726,#43727);
#36233=AXIS2_PLACEMENT_3D('',#53544,#43729,#43730);
#36234=AXIS2_PLACEMENT_3D('',#53545,#43731,#43732);
#36235=AXIS2_PLACEMENT_3D('',#53547,#43733,#43734);
#36236=AXIS2_PLACEMENT_3D('',#53549,#43736,#43737);
#36237=AXIS2_PLACEMENT_3D('',#53552,#43739,#43740);
#36238=AXIS2_PLACEMENT_3D('',#53553,#43741,#43742);
#36239=AXIS2_PLACEMENT_3D('',#53555,#43743,#43744);
#36240=AXIS2_PLACEMENT_3D('',#53557,#43746,#43747);
#36241=AXIS2_PLACEMENT_3D('',#53559,#43748,#43749);
#36242=AXIS2_PLACEMENT_3D('',#53561,#43751,#43752);
#36243=AXIS2_PLACEMENT_3D('',#53564,#43754,#43755);
#36244=AXIS2_PLACEMENT_3D('',#53566,#43756,#43757);
#36245=AXIS2_PLACEMENT_3D('',#53568,#43758,#43759);
#36246=AXIS2_PLACEMENT_3D('',#53570,#43760,#43761);
#36247=AXIS2_PLACEMENT_3D('',#53571,#43762,#43763);
#36248=AXIS2_PLACEMENT_3D('',#53573,#43765,#43766);
#36249=AXIS2_PLACEMENT_3D('',#53575,#43768,#43769);
#36250=AXIS2_PLACEMENT_3D('',#53577,#43771,#43772);
#36251=AXIS2_PLACEMENT_3D('',#53579,#43774,#43775);
#36252=AXIS2_PLACEMENT_3D('',#53580,#43776,#43777);
#36253=AXIS2_PLACEMENT_3D('',#53581,#43778,#43779);
#36254=AXIS2_PLACEMENT_3D('',#53582,#43780,#43781);
#36255=AXIS2_PLACEMENT_3D('',#53583,#43782,#43783);
#36256=AXIS2_PLACEMENT_3D('',#53584,#43784,#43785);
#36257=AXIS2_PLACEMENT_3D('',#53587,#43786,#43787);
#36258=AXIS2_PLACEMENT_3D('',#53588,#43788,#43789);
#36259=AXIS2_PLACEMENT_3D('',#53592,#43791,#43792);
#36260=AXIS2_PLACEMENT_3D('',#53593,#43793,#43794);
#36261=AXIS2_PLACEMENT_3D('',#53594,#43795,#43796);
#36262=AXIS2_PLACEMENT_3D('',#53598,#43798,#43799);
#36263=AXIS2_PLACEMENT_3D('',#53599,#43800,#43801);
#36264=AXIS2_PLACEMENT_3D('',#53600,#43802,#43803);
#36265=AXIS2_PLACEMENT_3D('',#53602,#43805,#43806);
#36266=AXIS2_PLACEMENT_3D('',#53605,#43808,#43809);
#36267=AXIS2_PLACEMENT_3D('',#53606,#43810,#43811);
#36268=AXIS2_PLACEMENT_3D('',#57631,#43812,#43813);
#36269=AXIS2_PLACEMENT_3D('',#57644,#43814,#43815);
#36270=AXIS2_PLACEMENT_3D('',#57645,#43816,#43817);
#36271=AXIS2_PLACEMENT_3D('',#57646,#43818,#43819);
#36272=AXIS2_PLACEMENT_3D('',#57657,#43820,#43821);
#36273=AXIS2_PLACEMENT_3D('',#57666,#43822,#43823);
#36274=AXIS2_PLACEMENT_3D('',#57686,#43824,#43825);
#36275=AXIS2_PLACEMENT_3D('',#57688,#43826,#43827);
#36276=AXIS2_PLACEMENT_3D('',#57689,#43828,#43829);
#36277=AXIS2_PLACEMENT_3D('',#57690,#43830,#43831);
#36278=AXIS2_PLACEMENT_3D('',#57694,#43833,#43834);
#36279=AXIS2_PLACEMENT_3D('',#57696,#43835,#43836);
#36280=AXIS2_PLACEMENT_3D('',#57697,#43837,#43838);
#36281=AXIS2_PLACEMENT_3D('',#57784,#43839,#43840);
#36282=AXIS2_PLACEMENT_3D('',#57786,#43841,#43842);
#36283=AXIS2_PLACEMENT_3D('',#57788,#43844,#43845);
#36284=AXIS2_PLACEMENT_3D('',#57791,#43848,#43849);
#36285=AXIS2_PLACEMENT_3D('',#57794,#43852,#43853);
#36286=AXIS2_PLACEMENT_3D('',#57797,#43856,#43857);
#36287=AXIS2_PLACEMENT_3D('',#57800,#43860,#43861);
#36288=AXIS2_PLACEMENT_3D('',#57803,#43864,#43865);
#36289=AXIS2_PLACEMENT_3D('',#57806,#43868,#43869);
#36290=AXIS2_PLACEMENT_3D('',#57809,#43872,#43873);
#36291=AXIS2_PLACEMENT_3D('',#57812,#43876,#43877);
#36292=AXIS2_PLACEMENT_3D('',#57820,#43880,#43881);
#36293=AXIS2_PLACEMENT_3D('',#57821,#43882,#43883);
#36294=AXIS2_PLACEMENT_3D('',#57824,#43886,#43887);
#36295=AXIS2_PLACEMENT_3D('',#57825,#43888,#43889);
#36296=AXIS2_PLACEMENT_3D('',#57832,#43890,#43891);
#36297=AXIS2_PLACEMENT_3D('',#57833,#43892,#43893);
#36298=AXIS2_PLACEMENT_3D('',#57834,#43894,#43895);
#36299=AXIS2_PLACEMENT_3D('',#57835,#43896,#43897);
#36300=AXIS2_PLACEMENT_3D('',#57836,#43898,#43899);
#36301=AXIS2_PLACEMENT_3D('',#57837,#43900,#43901);
#36302=AXIS2_PLACEMENT_3D('',#57846,#43902,#43903);
#36303=AXIS2_PLACEMENT_3D('',#57847,#43904,#43905);
#36304=AXIS2_PLACEMENT_3D('',#57848,#43906,#43907);
#36305=AXIS2_PLACEMENT_3D('',#57849,#43908,#43909);
#36306=AXIS2_PLACEMENT_3D('',#57850,#43910,#43911);
#36307=AXIS2_PLACEMENT_3D('',#57851,#43912,#43913);
#36308=AXIS2_PLACEMENT_3D('',#57852,#43914,#43915);
#36309=AXIS2_PLACEMENT_3D('',#57853,#43916,#43917);
#36310=AXIS2_PLACEMENT_3D('',#57869,#43918,#43919);
#36311=AXIS2_PLACEMENT_3D('',#57878,#43920,#43921);
#36312=AXIS2_PLACEMENT_3D('',#57888,#43923,#43924);
#36313=AXIS2_PLACEMENT_3D('',#57890,#43925,#43926);
#36314=AXIS2_PLACEMENT_3D('',#57892,#43928,#43929);
#36315=AXIS2_PLACEMENT_3D('',#57894,#43930,#43931);
#36316=AXIS2_PLACEMENT_3D('',#57896,#43933,#43934);
#36317=AXIS2_PLACEMENT_3D('',#57898,#43935,#43936);
#36318=AXIS2_PLACEMENT_3D('',#57899,#43937,#43938);
#36319=AXIS2_PLACEMENT_3D('',#57901,#43939,#43940);
#36320=AXIS2_PLACEMENT_3D('',#57903,#43942,#43943);
#36321=AXIS2_PLACEMENT_3D('',#57905,#43944,#43945);
#36322=AXIS2_PLACEMENT_3D('',#57907,#43947,#43948);
#36323=AXIS2_PLACEMENT_3D('',#57909,#43949,#43950);
#36324=AXIS2_PLACEMENT_3D('',#57911,#43952,#43953);
#36325=AXIS2_PLACEMENT_3D('',#57913,#43954,#43955);
#36326=AXIS2_PLACEMENT_3D('',#57915,#43957,#43958);
#36327=AXIS2_PLACEMENT_3D('',#57918,#43959,#43960);
#36328=AXIS2_PLACEMENT_3D('',#57921,#43963,#43964);
#36329=AXIS2_PLACEMENT_3D('',#57925,#43967,#43968);
#36330=AXIS2_PLACEMENT_3D('',#57929,#43970,#43971);
#36331=AXIS2_PLACEMENT_3D('',#57931,#43973,#43974);
#36332=AXIS2_PLACEMENT_3D('',#57932,#43975,#43976);
#36333=AXIS2_PLACEMENT_3D('',#57934,#43978,#43979);
#36334=AXIS2_PLACEMENT_3D('',#57936,#43980,#43981);
#36335=AXIS2_PLACEMENT_3D('',#57937,#43982,#43983);
#36336=AXIS2_PLACEMENT_3D('',#57939,#43984,#43985);
#36337=AXIS2_PLACEMENT_3D('',#57941,#43987,#43988);
#36338=AXIS2_PLACEMENT_3D('',#57946,#43990,#43991);
#36339=AXIS2_PLACEMENT_3D('',#57948,#43993,#43994);
#36340=AXIS2_PLACEMENT_3D('',#57949,#43995,#43996);
#43478=DIRECTION('axis',(0.,0.,1.));
#43479=DIRECTION('refdir',(1.,0.,0.));
#43480=DIRECTION('center_axis',(1.,0.,0.));
#43481=DIRECTION('ref_axis',(0.,0.655966063895196,-0.754790383495871));
#43482=DIRECTION('',(1.,0.,0.));
#43483=DIRECTION('center_axis',(1.,0.,0.));
#43484=DIRECTION('ref_axis',(0.,1.,4.47017618667391E-14));
#43485=DIRECTION('',(1.,0.,0.));
#43486=DIRECTION('center_axis',(1.,0.,0.));
#43487=DIRECTION('ref_axis',(0.,1.,4.47017618667391E-14));
#43488=DIRECTION('',(1.,0.,0.));
#43489=DIRECTION('center_axis',(1.,0.,0.));
#43490=DIRECTION('ref_axis',(0.,1.,4.47017618667391E-14));
#43491=DIRECTION('',(1.,0.,0.));
#43492=DIRECTION('center_axis',(1.,0.,0.));
#43493=DIRECTION('ref_axis',(0.,1.,4.47017618667391E-14));
#43494=DIRECTION('',(1.,0.,0.));
#43495=DIRECTION('center_axis',(1.,0.,0.));
#43496=DIRECTION('ref_axis',(0.,1.,4.47017618667391E-14));
#43497=DIRECTION('',(1.,0.,0.));
#43498=DIRECTION('center_axis',(1.,0.,0.));
#43499=DIRECTION('ref_axis',(0.,0.947929631065919,-0.31847984951521));
#43500=DIRECTION('',(1.,0.,0.));
#43501=DIRECTION('center_axis',(1.,0.,0.));
#43502=DIRECTION('ref_axis',(0.,1.,4.47017618667391E-14));
#43503=DIRECTION('center_axis',(1.,0.,0.));
#43504=DIRECTION('ref_axis',(0.,1.,4.47017618667391E-14));
#43505=DIRECTION('',(1.,0.,0.));
#43506=DIRECTION('center_axis',(1.,0.,0.));
#43507=DIRECTION('ref_axis',(0.,1.,4.47017618667391E-14));
#43508=DIRECTION('',(1.,0.,0.));
#43509=DIRECTION('center_axis',(1.,0.,3.99334313142758E-16));
#43510=DIRECTION('ref_axis',(0.,1.,2.6597345215342E-17));
#43511=DIRECTION('center_axis',(1.,0.,0.));
#43512=DIRECTION('ref_axis',(0.,1.,0.));
#43513=DIRECTION('',(-0.452487571992747,0.891770708866415,-4.77646659520457E-17));
#43514=DIRECTION('center_axis',(-1.,0.,0.));
#43515=DIRECTION('ref_axis',(0.,1.,6.12323399573677E-17));
#43516=DIRECTION('center_axis',(1.,0.,0.));
#43517=DIRECTION('ref_axis',(0.,1.,0.));
#43518=DIRECTION('',(0.807030325658429,-0.590509994384219,-7.23166174487155E-17));
#43519=DIRECTION('center_axis',(1.,0.,0.));
#43520=DIRECTION('ref_axis',(0.,0.,-1.));
#43521=DIRECTION('center_axis',(1.,0.,0.));
#43522=DIRECTION('ref_axis',(0.,0.,-1.));
#43523=DIRECTION('center_axis',(0.707106781186543,0.,-0.707106781186552));
#43524=DIRECTION('ref_axis',(-0.707106781186552,0.,-0.707106781186543));
#43525=DIRECTION('',(0.707106781186552,0.,0.707106781186543));
#43526=DIRECTION('',(0.,1.,0.));
#43527=DIRECTION('',(-0.707106781186552,0.,-0.707106781186543));
#43528=DIRECTION('',(0.,-1.,0.));
#43529=DIRECTION('center_axis',(0.,0.,1.));
#43530=DIRECTION('ref_axis',(0.,1.,0.));
#43531=DIRECTION('',(-1.,0.,0.));
#43532=DIRECTION('',(0.,1.,0.));
#43533=DIRECTION('',(-1.,0.,0.));
#43534=DIRECTION('center_axis',(0.,-0.38268343236509,0.923879532511287));
#43535=DIRECTION('ref_axis',(1.,0.,0.));
#43536=DIRECTION('',(-0.357406744336595,0.862856209461016,0.357406744336593));
#43537=DIRECTION('',(-1.,0.,0.));
#43538=DIRECTION('',(-0.357406744336594,-0.862856209461017,-0.357406744336594));
#43539=DIRECTION('',(0.357406744336593,-0.862856209461017,-0.357406744336594));
#43540=DIRECTION('',(1.,0.,0.));
#43541=DIRECTION('',(0.357406744336594,0.862856209461017,0.357406744336593));
#43542=DIRECTION('center_axis',(0.,-0.707106781186548,0.707106781186548));
#43543=DIRECTION('ref_axis',(0.,-0.707106781186548,-0.707106781186548));
#43544=DIRECTION('',(0.,0.707106781186548,0.707106781186548));
#43545=DIRECTION('',(-1.,0.,0.));
#43546=DIRECTION('',(0.,-0.707106781186548,-0.707106781186548));
#43547=DIRECTION('center_axis',(-0.707106781186548,-0.5,0.5));
#43548=DIRECTION('ref_axis',(0.577350269189625,0.,0.816496580927726));
#43549=DIRECTION('',(0.67859834454585,-0.281084637714835,0.678598344545838));
#43550=DIRECTION('',(0.,-0.707106781186548,-0.707106781186548));
#43551=DIRECTION('',(0.653281482438187,-0.191341716182544,0.732537816328743));
#43552=DIRECTION('center_axis',(-0.707106781186548,0.,0.707106781186548));
#43553=DIRECTION('ref_axis',(0.707106781186548,0.,0.707106781186548));
#43554=DIRECTION('',(0.,1.,0.));
#43555=DIRECTION('',(0.357406744336594,-0.862856209461017,0.357406744336594));
#43556=DIRECTION('',(0.678598344545847,0.281084637714822,0.678598344545847));
#43557=DIRECTION('',(0.,-1.,0.));
#43558=DIRECTION('center_axis',(0.573302186256021,0.313549377219833,0.756975158957757));
#43559=DIRECTION('ref_axis',(0.797175191421303,0.,-0.603748055220394));
#43560=DIRECTION('',(0.653281482438189,-0.732537816328742,-0.191341716182544));
#43561=DIRECTION('',(0.,0.923879532511287,-0.38268343236509));
#43562=DIRECTION('',(-0.653281482438193,-0.382683432365078,0.65328148243819));
#43563=DIRECTION('center_axis',(0.,0.38268343236509,0.923879532511287));
#43564=DIRECTION('ref_axis',(1.,0.,0.));
#43565=DIRECTION('',(1.,0.,0.));
#43566=DIRECTION('',(-1.,0.,0.));
#43567=DIRECTION('',(-0.357406744336593,-0.862856209461017,0.357406744336594));
#43568=DIRECTION('center_axis',(0.707106781186546,0.,0.707106781186549));
#43569=DIRECTION('ref_axis',(0.707106781186549,0.,-0.707106781186546));
#43570=DIRECTION('',(0.678598344545848,0.281084637714821,-0.678598344545845));
#43571=DIRECTION('',(0.,1.,0.));
#43572=DIRECTION('',(0.,-1.,0.));
#43573=DIRECTION('center_axis',(0.573302186256017,0.75697515895776,0.313549377219834));
#43574=DIRECTION('ref_axis',(0.479841491130335,0.,-0.87735519796136));
#43575=DIRECTION('',(0.65328148243819,-0.653281482438187,0.382683432365088));
#43576=DIRECTION('',(0.,0.38268343236509,-0.923879532511287));
#43577=DIRECTION('',(-0.653281482438189,0.191341716182544,0.732537816328742));
#43578=DIRECTION('center_axis',(0.,0.923879532511287,0.38268343236509));
#43579=DIRECTION('ref_axis',(0.,-0.38268343236509,0.923879532511287));
#43580=DIRECTION('',(0.357406744336592,-0.357406744336594,0.862856209461017));
#43581=DIRECTION('',(1.,0.,0.));
#43582=DIRECTION('',(-1.,0.,0.));
#43583=DIRECTION('',(-0.357406744336593,-0.357406744336593,0.862856209461017));
#43584=DIRECTION('center_axis',(0.707106781186547,0.500000000000001,0.500000000000001));
#43585=DIRECTION('ref_axis',(0.577350269189627,0.,-0.816496580927725));
#43586=DIRECTION('',(0.,0.707106781186548,-0.707106781186548));
#43587=DIRECTION('',(0.,-0.707106781186548,0.707106781186548));
#43588=DIRECTION('center_axis',(0.573302186256021,0.756975158957757,-0.313549377219833));
#43589=DIRECTION('ref_axis',(-0.479841491130332,0.,-0.877355197961361));
#43590=DIRECTION('',(0.653281482438189,-0.191341716182544,0.732537816328742));
#43591=DIRECTION('',(0.,-0.38268343236509,-0.923879532511287));
#43592=DIRECTION('',(-0.653281482438193,0.65328148243819,0.382683432365078));
#43593=DIRECTION('center_axis',(0.,0.923879532511287,-0.38268343236509));
#43594=DIRECTION('ref_axis',(0.,0.38268343236509,0.923879532511287));
#43595=DIRECTION('',(0.357406744336593,0.357406744336593,0.862856209461017));
#43596=DIRECTION('',(1.,0.,0.));
#43597=DIRECTION('',(-1.,0.,0.));
#43598=DIRECTION('',(-0.357406744336592,0.357406744336594,0.862856209461017));
#43599=DIRECTION('center_axis',(0.707106781186546,0.707106781186549,0.));
#43600=DIRECTION('ref_axis',(0.,0.,-1.));
#43601=DIRECTION('',(0.,0.,-1.));
#43602=DIRECTION('',(0.,0.,1.));
#43603=DIRECTION('center_axis',(0.573302186256017,0.313549377219834,-0.75697515895776));
#43604=DIRECTION('ref_axis',(-0.797175191421306,0.,-0.603748055220391));
#43605=DIRECTION('',(0.65328148243819,0.382683432365088,0.653281482438187));
#43606=DIRECTION('',(0.,-0.923879532511287,-0.38268343236509));
#43607=DIRECTION('',(-0.653281482438189,0.732537816328742,-0.191341716182544));
#43608=DIRECTION('center_axis',(0.,0.38268343236509,-0.923879532511287));
#43609=DIRECTION('ref_axis',(-1.,0.,0.));
#43610=DIRECTION('',(0.357406744336593,0.862856209461017,0.357406744336594));
#43611=DIRECTION('',(1.,0.,0.));
#43612=DIRECTION('',(-1.,0.,0.));
#43613=DIRECTION('',(-0.357406744336594,0.862856209461017,0.357406744336594));
#43614=DIRECTION('center_axis',(0.707106781186547,0.500000000000001,-0.500000000000001));
#43615=DIRECTION('ref_axis',(-0.577350269189627,0.,-0.816496580927725));
#43616=DIRECTION('',(0.,-0.707106781186548,-0.707106781186548));
#43617=DIRECTION('',(0.,0.707106781186548,0.707106781186548));
#43618=DIRECTION('center_axis',(0.573302186256021,-0.313549377219833,-0.756975158957757));
#43619=DIRECTION('ref_axis',(-0.797175191421303,0.,-0.603748055220394));
#43620=DIRECTION('',(0.653281482438189,0.732537816328742,0.191341716182544));
#43621=DIRECTION('',(0.,-0.923879532511287,0.38268343236509));
#43622=DIRECTION('',(-0.653281482438193,0.382683432365078,-0.65328148243819));
#43623=DIRECTION('center_axis',(0.,-0.38268343236509,-0.923879532511287));
#43624=DIRECTION('ref_axis',(-1.,0.,0.));
#43625=DIRECTION('',(0.357406744336594,0.862856209461017,-0.357406744336594));
#43626=DIRECTION('',(1.,0.,0.));
#43627=DIRECTION('',(-1.,0.,0.));
#43628=DIRECTION('',(-0.357406744336593,0.862856209461017,-0.357406744336594));
#43629=DIRECTION('center_axis',(0.707106781186546,0.,-0.707106781186549));
#43630=DIRECTION('ref_axis',(-0.707106781186549,0.,-0.707106781186546));
#43631=DIRECTION('',(0.,-1.,0.));
#43632=DIRECTION('',(0.,1.,0.));
#43633=DIRECTION('center_axis',(0.573302186256017,-0.75697515895776,-0.313549377219834));
#43634=DIRECTION('ref_axis',(-0.479841491130335,0.,-0.87735519796136));
#43635=DIRECTION('',(0.65328148243819,0.653281482438187,-0.382683432365088));
#43636=DIRECTION('',(0.,-0.38268343236509,0.923879532511287));
#43637=DIRECTION('',(-0.653281482438189,-0.191341716182544,-0.732537816328742));
#43638=DIRECTION('center_axis',(0.,-0.923879532511287,-0.38268343236509));
#43639=DIRECTION('ref_axis',(0.,0.38268343236509,-0.923879532511287));
#43640=DIRECTION('',(0.357406744336592,0.357406744336594,-0.862856209461017));
#43641=DIRECTION('',(1.,0.,0.));
#43642=DIRECTION('',(-1.,0.,0.));
#43643=DIRECTION('',(-0.357406744336593,0.357406744336593,-0.862856209461017));
#43644=DIRECTION('center_axis',(0.707106781186547,-0.500000000000001,-0.500000000000001));
#43645=DIRECTION('ref_axis',(-0.577350269189627,0.,-0.816496580927725));
#43646=DIRECTION('',(0.,-0.707106781186548,0.707106781186548));
#43647=DIRECTION('',(0.,0.707106781186548,-0.707106781186548));
#43648=DIRECTION('center_axis',(0.707106781186546,-0.707106781186549,0.));
#43649=DIRECTION('ref_axis',(0.,0.,-1.));
#43650=DIRECTION('',(-0.357406744336595,-0.357406744336593,-0.862856209461016));
#43651=DIRECTION('',(0.,0.,-1.));
#43652=DIRECTION('',(0.,0.,1.));
#43653=DIRECTION('',(-0.678598344545848,-0.678598344545845,0.281084637714821));
#43654=DIRECTION('center_axis',(-0.707106781186548,0.707106781186548,0.));
#43655=DIRECTION('ref_axis',(0.,0.,1.));
#43656=DIRECTION('',(0.678598344545847,0.678598344545847,-0.281084637714822));
#43657=DIRECTION('',(0.,0.,1.));
#43658=DIRECTION('',(0.67859834454585,0.678598344545838,0.281084637714835));
#43659=DIRECTION('',(0.,0.,-1.));
#43660=DIRECTION('center_axis',(0.,0.707106781186548,-0.707106781186548));
#43661=DIRECTION('ref_axis',(0.,0.707106781186548,0.707106781186548));
#43662=DIRECTION('',(0.,-0.707106781186548,-0.707106781186548));
#43663=DIRECTION('center_axis',(-0.707106781186548,0.5,-0.5));
#43664=DIRECTION('ref_axis',(-0.577350269189625,0.,0.816496580927726));
#43665=DIRECTION('',(0.67859834454585,0.281084637714835,-0.678598344545838));
#43666=DIRECTION('',(0.,0.707106781186548,0.707106781186548));
#43667=DIRECTION('center_axis',(0.,0.,-1.));
#43668=DIRECTION('ref_axis',(0.,1.,0.));
#43669=DIRECTION('',(0.,-1.,0.));
#43670=DIRECTION('center_axis',(-0.707106781186548,0.,-0.707106781186548));
#43671=DIRECTION('ref_axis',(-0.707106781186548,0.,0.707106781186548));
#43672=DIRECTION('',(0.678598344545847,-0.281084637714822,-0.678598344545847));
#43673=DIRECTION('',(0.,1.,0.));
#43674=DIRECTION('center_axis',(0.,-0.707106781186548,-0.707106781186548));
#43675=DIRECTION('ref_axis',(0.,0.707106781186548,-0.707106781186548));
#43676=DIRECTION('',(0.,-0.707106781186548,0.707106781186548));
#43677=DIRECTION('center_axis',(-0.707106781186548,-0.5,-0.5));
#43678=DIRECTION('ref_axis',(-0.577350269189625,0.,0.816496580927726));
#43679=DIRECTION('',(0.67859834454585,-0.678598344545838,-0.281084637714835));
#43680=DIRECTION('',(0.,0.707106781186548,-0.707106781186548));
#43681=DIRECTION('center_axis',(-0.707106781186548,-0.707106781186548,0.));
#43682=DIRECTION('ref_axis',(0.,0.,1.));
#43683=DIRECTION('',(0.,0.,1.));
#43684=DIRECTION('',(-0.653281482438189,0.653281482438189,0.382683432365089));
#43685=DIRECTION('',(0.,0.,-1.));
#43686=DIRECTION('center_axis',(0.,-1.,0.));
#43687=DIRECTION('ref_axis',(0.,0.,-1.));
#43688=DIRECTION('',(1.,0.,0.));
#43689=DIRECTION('center_axis',(0.,-0.923879532511287,0.38268343236509));
#43690=DIRECTION('ref_axis',(0.,-0.38268343236509,-0.923879532511287));
#43691=DIRECTION('',(-0.35740674433659,0.357406744336597,0.862856209461016));
#43692=DIRECTION('',(0.,-0.38268343236509,-0.923879532511287));
#43693=DIRECTION('center_axis',(1.,0.,0.));
#43694=DIRECTION('ref_axis',(0.,0.,-1.));
#43695=DIRECTION('center_axis',(1.,0.,0.));
#43696=DIRECTION('ref_axis',(0.,0.,-1.));
#43697=DIRECTION('',(-0.707106781186549,8.65956056235492E-17,-0.707106781186546));
#43698=DIRECTION('center_axis',(-1.,0.,0.));
#43699=DIRECTION('ref_axis',(0.,0.,-1.));
#43700=DIRECTION('center_axis',(1.,0.,0.));
#43701=DIRECTION('ref_axis',(0.,0.,-1.));
#43702=DIRECTION('',(0.,0.707106781186548,0.707106781186548));
#43703=DIRECTION('center_axis',(1.,0.,0.));
#43704=DIRECTION('ref_axis',(0.,0.,-1.));
#43705=DIRECTION('center_axis',(1.,0.,0.));
#43706=DIRECTION('ref_axis',(0.,0.,-1.));
#43707=DIRECTION('center_axis',(1.,0.,0.));
#43708=DIRECTION('ref_axis',(0.,0.,-1.));
#43709=DIRECTION('center_axis',(1.,0.,0.));
#43710=DIRECTION('ref_axis',(0.,0.,-1.));
#43711=DIRECTION('center_axis',(1.,0.,0.));
#43712=DIRECTION('ref_axis',(0.,0.,-1.));
#43713=DIRECTION('center_axis',(1.,0.,0.));
#43714=DIRECTION('ref_axis',(0.,0.,-1.));
#43715=DIRECTION('',(1.,0.,0.));
#43716=DIRECTION('center_axis',(1.,0.,0.));
#43717=DIRECTION('ref_axis',(0.,0.,-1.));
#43718=DIRECTION('',(-0.707106781186549,8.65956056235491E-17,-0.707106781186546));
#43719=DIRECTION('center_axis',(-1.,0.,0.));
#43720=DIRECTION('ref_axis',(0.,0.,-1.));
#43721=DIRECTION('center_axis',(1.,0.,0.));
#43722=DIRECTION('ref_axis',(0.,0.,-1.));
#43723=DIRECTION('center_axis',(1.,0.,0.));
#43724=DIRECTION('ref_axis',(0.,0.,-1.));
#43725=DIRECTION('',(1.,0.,0.));
#43726=DIRECTION('center_axis',(1.,0.,0.));
#43727=DIRECTION('ref_axis',(0.,0.,-1.));
#43728=DIRECTION('',(-0.707106781186549,8.65956056235491E-17,-0.707106781186546));
#43729=DIRECTION('center_axis',(-1.,0.,0.));
#43730=DIRECTION('ref_axis',(0.,0.,-1.));
#43731=DIRECTION('center_axis',(1.,0.,0.));
#43732=DIRECTION('ref_axis',(0.,0.,-1.));
#43733=DIRECTION('center_axis',(1.,0.,0.));
#43734=DIRECTION('ref_axis',(0.,0.,-1.));
#43735=DIRECTION('',(1.,0.,0.));
#43736=DIRECTION('center_axis',(1.,0.,0.));
#43737=DIRECTION('ref_axis',(0.,0.,-1.));
#43738=DIRECTION('',(-0.707106781186549,8.65956056235491E-17,-0.707106781186546));
#43739=DIRECTION('center_axis',(-1.,0.,0.));
#43740=DIRECTION('ref_axis',(0.,0.,-1.));
#43741=DIRECTION('center_axis',(1.,0.,0.));
#43742=DIRECTION('ref_axis',(0.,0.,-1.));
#43743=DIRECTION('center_axis',(1.,0.,0.));
#43744=DIRECTION('ref_axis',(0.,0.,-1.));
#43745=DIRECTION('',(1.,0.,0.));
#43746=DIRECTION('center_axis',(-1.,0.,0.));
#43747=DIRECTION('ref_axis',(0.,0.,-1.));
#43748=DIRECTION('center_axis',(-1.,0.,0.));
#43749=DIRECTION('ref_axis',(0.,0.,-1.));
#43750=DIRECTION('',(0.707106781186548,-8.65956056235493E-17,-0.707106781186548));
#43751=DIRECTION('center_axis',(1.,0.,0.));
#43752=DIRECTION('ref_axis',(0.,0.,-1.));
#43753=DIRECTION('',(0.,-0.707106781186548,0.707106781186548));
#43754=DIRECTION('center_axis',(-1.,0.,0.));
#43755=DIRECTION('ref_axis',(0.,0.,-1.));
#43756=DIRECTION('center_axis',(-1.,0.,0.));
#43757=DIRECTION('ref_axis',(0.,0.,-1.));
#43758=DIRECTION('center_axis',(-1.,0.,0.));
#43759=DIRECTION('ref_axis',(0.,1.,0.));
#43760=DIRECTION('center_axis',(-1.,0.,0.));
#43761=DIRECTION('ref_axis',(0.,0.,-1.));
#43762=DIRECTION('center_axis',(-1.,0.,0.));
#43763=DIRECTION('ref_axis',(0.,0.,-1.));
#43764=DIRECTION('',(0.707106781186548,-8.65956056235493E-17,-0.707106781186548));
#43765=DIRECTION('center_axis',(-1.,0.,0.));
#43766=DIRECTION('ref_axis',(0.,0.,-1.));
#43767=DIRECTION('',(0.707106781186548,-8.65956056235493E-17,-0.707106781186548));
#43768=DIRECTION('center_axis',(-1.,0.,0.));
#43769=DIRECTION('ref_axis',(0.,0.,-1.));
#43770=DIRECTION('',(0.707106781186547,-8.65956056235493E-17,-0.707106781186547));
#43771=DIRECTION('center_axis',(-0.707106781186548,0.5,0.5));
#43772=DIRECTION('ref_axis',(0.577350269189625,0.,0.816496580927726));
#43773=DIRECTION('',(0.,0.707106781186548,-0.707106781186548));
#43774=DIRECTION('center_axis',(-0.573302186256018,-0.756975158957759,0.313549377219833));
#43775=DIRECTION('ref_axis',(0.479841491130334,0.,0.87735519796136));
#43776=DIRECTION('center_axis',(0.707106781186547,-0.500000000000001,0.500000000000001));
#43777=DIRECTION('ref_axis',(0.577350269189627,0.,-0.816496580927725));
#43778=DIRECTION('center_axis',(0.,1.,0.));
#43779=DIRECTION('ref_axis',(0.,0.,1.));
#43780=DIRECTION('center_axis',(0.,0.707106781186548,0.707106781186548));
#43781=DIRECTION('ref_axis',(0.,-0.707106781186548,0.707106781186548));
#43782=DIRECTION('center_axis',(0.,0.,1.));
#43783=DIRECTION('ref_axis',(0.,-1.,0.));
#43784=DIRECTION('center_axis',(1.,0.,1.79678570832605E-15));
#43785=DIRECTION('ref_axis',(0.,-1.,-3.04015968733321E-17));
#43786=DIRECTION('center_axis',(-1.,0.,0.));
#43787=DIRECTION('ref_axis',(0.,-1.,0.));
#43788=DIRECTION('center_axis',(-1.,0.,0.));
#43789=DIRECTION('ref_axis',(0.,-1.,0.));
#43790=DIRECTION('',(-0.923879532511291,-0.382683432365078,-1.71851293172537E-15));
#43791=DIRECTION('center_axis',(1.,0.,0.));
#43792=DIRECTION('ref_axis',(0.,-1.,-6.12323399573677E-17));
#43793=DIRECTION('center_axis',(1.,0.,0.));
#43794=DIRECTION('ref_axis',(0.,-1.,-6.12323399573677E-17));
#43795=DIRECTION('center_axis',(1.,0.,0.));
#43796=DIRECTION('ref_axis',(0.,1.,0.));
#43797=DIRECTION('',(-0.707106781186548,0.707106781186548,8.65956056235493E-17));
#43798=DIRECTION('center_axis',(-1.,0.,0.));
#43799=DIRECTION('ref_axis',(0.,-1.,-6.12323399573677E-17));
#43800=DIRECTION('center_axis',(-1.,0.,0.));
#43801=DIRECTION('ref_axis',(0.,-1.,-6.12323399573677E-17));
#43802=DIRECTION('center_axis',(1.,0.,0.));
#43803=DIRECTION('ref_axis',(0.,1.,0.));
#43804=DIRECTION('',(-1.,0.,0.));
#43805=DIRECTION('center_axis',(1.,0.,-4.321736136636E-15));
#43806=DIRECTION('ref_axis',(0.,-1.,-3.11489047937176E-17));
#43807=DIRECTION('',(-0.382683432365088,-0.923879532511287,1.51193637171627E-15));
#43808=DIRECTION('center_axis',(1.,0.,0.));
#43809=DIRECTION('ref_axis',(0.,-1.,0.));
#43810=DIRECTION('center_axis',(-1.,0.,0.));
#43811=DIRECTION('ref_axis',(0.,0.,1.));
#43812=DIRECTION('center_axis',(1.,0.,0.));
#43813=DIRECTION('ref_axis',(0.,0.662617229149953,0.748958214878266));
#43814=DIRECTION('center_axis',(1.,0.,0.));
#43815=DIRECTION('ref_axis',(0.,1.,4.47017618667391E-14));
#43816=DIRECTION('center_axis',(-1.,0.,0.));
#43817=DIRECTION('ref_axis',(0.,1.,4.47017618667391E-14));
#43818=DIRECTION('center_axis',(1.,0.,0.));
#43819=DIRECTION('ref_axis',(0.,-0.999706152813195,-0.0242406276206029));
#43820=DIRECTION('center_axis',(1.,0.,0.));
#43821=DIRECTION('ref_axis',(0.,-0.999825056376581,0.0187044551261706));
#43822=DIRECTION('center_axis',(1.,0.,0.));
#43823=DIRECTION('ref_axis',(0.,1.,4.47017618667391E-14));
#43824=DIRECTION('center_axis',(1.,0.,0.));
#43825=DIRECTION('ref_axis',(0.,0.,-1.));
#43826=DIRECTION('center_axis',(-1.,0.,0.));
#43827=DIRECTION('ref_axis',(0.,1.,0.));
#43828=DIRECTION('center_axis',(-1.,0.,0.));
#43829=DIRECTION('ref_axis',(0.,1.,0.));
#43830=DIRECTION('center_axis',(1.,0.,0.));
#43831=DIRECTION('ref_axis',(0.,0.,-1.));
#43832=DIRECTION('',(0.,-1.,0.));
#43833=DIRECTION('center_axis',(1.,0.,0.));
#43834=DIRECTION('ref_axis',(0.,1.,0.));
#43835=DIRECTION('center_axis',(1.,0.,0.));
#43836=DIRECTION('ref_axis',(0.,1.,0.));
#43837=DIRECTION('center_axis',(1.,0.,0.));
#43838=DIRECTION('ref_axis',(0.,1.,0.));
#43839=DIRECTION('center_axis',(0.,0.,1.));
#43840=DIRECTION('ref_axis',(0.,1.,0.));
#43841=DIRECTION('center_axis',(0.,0.,-1.));
#43842=DIRECTION('ref_axis',(1.,0.,0.));
#43843=DIRECTION('',(-1.,0.,0.));
#43844=DIRECTION('center_axis',(0.,0.,1.));
#43845=DIRECTION('ref_axis',(0.,1.,0.));
#43846=DIRECTION('',(-1.,0.,0.));
#43847=DIRECTION('',(1.,0.,0.));
#43848=DIRECTION('center_axis',(0.,0.,1.));
#43849=DIRECTION('ref_axis',(0.,1.,0.));
#43850=DIRECTION('',(1.,0.,0.));
#43851=DIRECTION('',(-1.,0.,0.));
#43852=DIRECTION('center_axis',(0.,0.,1.));
#43853=DIRECTION('ref_axis',(0.,1.,0.));
#43854=DIRECTION('',(1.,0.,0.));
#43855=DIRECTION('',(-1.,0.,0.));
#43856=DIRECTION('center_axis',(0.,0.,1.));
#43857=DIRECTION('ref_axis',(0.,1.,0.));
#43858=DIRECTION('',(1.,0.,0.));
#43859=DIRECTION('',(-1.,0.,0.));
#43860=DIRECTION('center_axis',(0.,0.,1.));
#43861=DIRECTION('ref_axis',(0.,1.,0.));
#43862=DIRECTION('',(1.,0.,0.));
#43863=DIRECTION('',(-1.,0.,0.));
#43864=DIRECTION('center_axis',(0.,0.,1.));
#43865=DIRECTION('ref_axis',(0.,1.,0.));
#43866=DIRECTION('',(1.,0.,0.));
#43867=DIRECTION('',(-1.,0.,0.));
#43868=DIRECTION('center_axis',(0.,0.,1.));
#43869=DIRECTION('ref_axis',(0.,1.,0.));
#43870=DIRECTION('',(-1.,0.,0.));
#43871=DIRECTION('',(1.,0.,0.));
#43872=DIRECTION('center_axis',(0.,0.,1.));
#43873=DIRECTION('ref_axis',(0.,1.,0.));
#43874=DIRECTION('',(-1.,0.,0.));
#43875=DIRECTION('',(1.,0.,0.));
#43876=DIRECTION('center_axis',(0.,0.,1.));
#43877=DIRECTION('ref_axis',(0.,1.,0.));
#43878=DIRECTION('',(1.,0.,0.));
#43879=DIRECTION('',(-1.,0.,0.));
#43880=DIRECTION('center_axis',(0.,0.,1.));
#43881=DIRECTION('ref_axis',(0.,1.,0.));
#43882=DIRECTION('center_axis',(0.,0.,-1.));
#43883=DIRECTION('ref_axis',(1.,0.,0.));
#43884=DIRECTION('',(1.,0.,0.));
#43885=DIRECTION('',(-1.,0.,0.));
#43886=DIRECTION('center_axis',(1.,0.,0.));
#43887=DIRECTION('ref_axis',(0.,4.25719507862852E-15,1.));
#43888=DIRECTION('center_axis',(1.,0.,0.));
#43889=DIRECTION('ref_axis',(0.,-0.99996617381244,0.00822503683331852));
#43890=DIRECTION('center_axis',(1.,0.,0.));
#43891=DIRECTION('ref_axis',(0.,1.13626224362295E-14,1.));
#43892=DIRECTION('center_axis',(1.,0.,0.));
#43893=DIRECTION('ref_axis',(0.,1.40271576953299E-14,1.));
#43894=DIRECTION('center_axis',(-1.,0.,0.));
#43895=DIRECTION('ref_axis',(0.,1.,0.));
#43896=DIRECTION('center_axis',(1.,0.,0.));
#43897=DIRECTION('ref_axis',(0.,1.,0.));
#43898=DIRECTION('center_axis',(-1.,0.,0.));
#43899=DIRECTION('ref_axis',(0.,1.,0.));
#43900=DIRECTION('center_axis',(1.,0.,0.));
#43901=DIRECTION('ref_axis',(0.,1.,0.));
#43902=DIRECTION('center_axis',(1.,0.,0.));
#43903=DIRECTION('ref_axis',(0.,2.04893359930602E-14,1.));
#43904=DIRECTION('center_axis',(1.,0.,0.));
#43905=DIRECTION('ref_axis',(0.,1.1607551796059E-14,1.));
#43906=DIRECTION('center_axis',(1.,0.,0.));
#43907=DIRECTION('ref_axis',(0.,-1.59259792146449E-14,1.));
#43908=DIRECTION('center_axis',(1.,0.,0.));
#43909=DIRECTION('ref_axis',(0.,3.86969935969128E-14,1.));
#43910=DIRECTION('center_axis',(1.,0.,0.));
#43911=DIRECTION('ref_axis',(0.,-2.52518526214962E-14,1.));
#43912=DIRECTION('center_axis',(1.,0.,0.));
#43913=DIRECTION('ref_axis',(0.,-0.957484047746987,0.288486218579061));
#43914=DIRECTION('center_axis',(1.,0.,0.));
#43915=DIRECTION('ref_axis',(0.,1.,0.));
#43916=DIRECTION('center_axis',(1.,0.,0.));
#43917=DIRECTION('ref_axis',(0.,-1.08418380562736E-14,1.));
#43918=DIRECTION('center_axis',(1.,0.,0.));
#43919=DIRECTION('ref_axis',(0.,-0.999997956527064,-0.00202161858351363));
#43920=DIRECTION('center_axis',(0.,0.,-1.));
#43921=DIRECTION('ref_axis',(1.,0.,0.));
#43922=DIRECTION('',(0.,0.,-1.));
#43923=DIRECTION('center_axis',(-1.,0.,0.));
#43924=DIRECTION('ref_axis',(0.,1.,0.));
#43925=DIRECTION('center_axis',(1.,0.,0.));
#43926=DIRECTION('ref_axis',(0.,0.,-1.));
#43927=DIRECTION('',(-0.387484117215795,-0.921876379405339,-1.1289729572483E-16));
#43928=DIRECTION('center_axis',(1.,0.,0.));
#43929=DIRECTION('ref_axis',(0.,1.,0.));
#43930=DIRECTION('center_axis',(1.,0.,0.));
#43931=DIRECTION('ref_axis',(0.,0.,-1.));
#43932=DIRECTION('',(-1.,0.,0.));
#43933=DIRECTION('center_axis',(1.,0.,0.));
#43934=DIRECTION('ref_axis',(0.,0.,-1.));
#43935=DIRECTION('center_axis',(1.,0.,0.));
#43936=DIRECTION('ref_axis',(0.,0.,-1.));
#43937=DIRECTION('center_axis',(-1.,0.,0.));
#43938=DIRECTION('ref_axis',(0.,1.,0.));
#43939=DIRECTION('center_axis',(1.,0.,0.));
#43940=DIRECTION('ref_axis',(0.,0.,-1.));
#43941=DIRECTION('',(-0.707106781186547,-0.707106781186548,-8.65956056235494E-17));
#43942=DIRECTION('center_axis',(1.,0.,0.));
#43943=DIRECTION('ref_axis',(0.,1.,0.));
#43944=DIRECTION('center_axis',(1.,0.,0.));
#43945=DIRECTION('ref_axis',(0.,0.,-1.));
#43946=DIRECTION('',(-1.,0.,0.));
#43947=DIRECTION('center_axis',(-1.,0.,0.));
#43948=DIRECTION('ref_axis',(0.,1.,0.));
#43949=DIRECTION('center_axis',(1.,0.,0.));
#43950=DIRECTION('ref_axis',(0.,0.,-1.));
#43951=DIRECTION('',(-0.81923192051904,-0.573462344363328,-7.02288824456087E-17));
#43952=DIRECTION('center_axis',(-1.,0.,0.));
#43953=DIRECTION('ref_axis',(0.,1.,0.));
#43954=DIRECTION('center_axis',(1.,0.,0.));
#43955=DIRECTION('ref_axis',(0.,0.,-1.));
#43956=DIRECTION('',(-0.707106781186546,-0.707106781186549,-8.65956056235495E-17));
#43957=DIRECTION('center_axis',(-1.,0.,0.));
#43958=DIRECTION('ref_axis',(0.,0.,1.));
#43959=DIRECTION('center_axis',(-1.,0.,0.));
#43960=DIRECTION('ref_axis',(0.,1.,0.));
#43961=DIRECTION('',(0.,0.,-1.));
#43962=DIRECTION('',(0.,0.,1.));
#43963=DIRECTION('center_axis',(0.,-1.,0.));
#43964=DIRECTION('ref_axis',(0.,0.,1.));
#43965=DIRECTION('',(0.,0.,1.));
#43966=DIRECTION('',(1.,0.,0.));
#43967=DIRECTION('center_axis',(1.,0.,0.));
#43968=DIRECTION('ref_axis',(0.,1.,0.));
#43969=DIRECTION('',(-1.,0.,0.));
#43970=DIRECTION('center_axis',(1.,0.,0.));
#43971=DIRECTION('ref_axis',(0.,0.,-1.));
#43972=DIRECTION('',(-1.,0.,0.));
#43973=DIRECTION('center_axis',(1.,0.,0.));
#43974=DIRECTION('ref_axis',(0.,0.,-1.));
#43975=DIRECTION('center_axis',(0.,1.,0.));
#43976=DIRECTION('ref_axis',(0.,0.,-1.));
#43977=DIRECTION('',(0.,0.,-1.));
#43978=DIRECTION('center_axis',(1.,0.,0.));
#43979=DIRECTION('ref_axis',(0.,0.,-1.));
#43980=DIRECTION('center_axis',(1.,0.,0.));
#43981=DIRECTION('ref_axis',(0.,0.,-1.));
#43982=DIRECTION('center_axis',(1.,0.,0.));
#43983=DIRECTION('ref_axis',(0.,1.,0.));
#43984=DIRECTION('center_axis',(1.,0.,0.));
#43985=DIRECTION('ref_axis',(0.,0.,-1.));
#43986=DIRECTION('',(-1.,0.,0.));
#43987=DIRECTION('center_axis',(1.,0.,0.));
#43988=DIRECTION('ref_axis',(0.,1.,0.));
#43989=DIRECTION('',(-0.529998940003185,0.847998304005085,1.03849840868221E-16));
#43990=DIRECTION('center_axis',(-1.,0.,0.));
#43991=DIRECTION('ref_axis',(0.,1.,0.));
#43992=DIRECTION('',(-0.707106781186549,-0.707106781186546,-8.65956056235492E-17));
#43993=DIRECTION('center_axis',(0.,0.,1.));
#43994=DIRECTION('ref_axis',(0.,1.,0.));
#43995=DIRECTION('center_axis',(1.,0.,0.));
#43996=DIRECTION('ref_axis',(0.,1.,0.));
#52952=CARTESIAN_POINT('',(0.,0.,0.));
#52953=CARTESIAN_POINT('Origin',(93.0806848796603,0.,0.));
#52954=CARTESIAN_POINT('',(106.687827736803,-11.5967315487946,7.87168637228455E-6));
#52955=CARTESIAN_POINT('',(107.068507977483,-11.5985329378162,-8.63915123328063E-5));
#52956=CARTESIAN_POINT('',(93.0806848796603,-11.59764,-5.19855242766535E-13));
#52957=CARTESIAN_POINT('',(108.008153428708,1.61683638546944,11.4839173606684));
#52958=CARTESIAN_POINT('Ctrl Pts',(106.687827736803,-11.5967315487946,7.87168637238211E-6));
#52959=CARTESIAN_POINT('Ctrl Pts',(106.711594970266,-11.596708823616,-0.954793789917175));
#52960=CARTESIAN_POINT('Ctrl Pts',(106.782454004811,-11.2488354439901,-3.80143203778901));
#52961=CARTESIAN_POINT('Ctrl Pts',(106.90040484044,-8.94469671038593,-8.10505773452174));
#52962=CARTESIAN_POINT('Ctrl Pts',(107.041680243689,-4.08614924745149,-11.3579434776441));
#52963=CARTESIAN_POINT('Ctrl Pts',(107.182955646938,1.73118676492076,-11.9458275473958));
#52964=CARTESIAN_POINT('Ctrl Pts',(107.324231050188,7.14228240914768,-9.73071187083892));
#52965=CARTESIAN_POINT('Ctrl Pts',(107.465506453437,10.8775923704873,-5.2324691939163));
#52966=CARTESIAN_POINT('Ctrl Pts',(107.606781856686,12.0604357325722,0.493684347847536));
#52967=CARTESIAN_POINT('Ctrl Pts',(107.748057259935,10.4137508886283,6.10364517469624));
#52968=CARTESIAN_POINT('Ctrl Pts',(107.881847783942,6.53964630458162,10.0607723786066));
#52969=CARTESIAN_POINT('Ctrl Pts',(107.968546506866,3.1919014918455,11.2608399260662));
#52970=CARTESIAN_POINT('Ctrl Pts',(108.008153428708,1.61683638546944,11.4839173606684));
#52971=CARTESIAN_POINT('',(108.381837686686,1.89465380507476,11.4418329182223));
#52972=CARTESIAN_POINT('Ctrl Pts',(108.381837686686,1.89465380507475,11.4418329182223));
#52973=CARTESIAN_POINT('Ctrl Pts',(108.245634554207,1.81427119940562,11.4551434787576));
#52974=CARTESIAN_POINT('Ctrl Pts',(108.119678552464,1.71980777108499,11.4698872225825));
#52975=CARTESIAN_POINT('Ctrl Pts',(108.008153428707,1.61690871966318,11.4843745916736));
#52976=CARTESIAN_POINT('',(107.547344722949,1.0134778581722,-11.5532729648613));
#52977=CARTESIAN_POINT('Ctrl Pts',(107.547344722949,1.01347785817195,-11.5532729648613));
#52978=CARTESIAN_POINT('Ctrl Pts',(107.609159016559,3.48672851139089,-11.3363141184487));
#52979=CARTESIAN_POINT('Ctrl Pts',(107.701880456974,7.0775262685878,-9.77461236926229));
#52980=CARTESIAN_POINT('Ctrl Pts',(107.825509044195,10.2343745743181,-5.85997992529276));
#52981=CARTESIAN_POINT('Ctrl Pts',(107.949137631415,12.0158490350764,-1.15276339618737));
#52982=CARTESIAN_POINT('Ctrl Pts',(108.072766218635,11.3809885644172,4.02471057714319));
#52983=CARTESIAN_POINT('Ctrl Pts',(108.227301952661,7.79854554867288,9.20330948728365));
#52984=CARTESIAN_POINT('Ctrl Pts',(108.320023393076,4.34404808711794,11.0362375708885));
#52985=CARTESIAN_POINT('Ctrl Pts',(108.381837686686,1.89465380507476,11.4418329182223));
#52986=CARTESIAN_POINT('',(107.3,-5.24483772964977E-16,-11.59764));
#52987=CARTESIAN_POINT('Ctrl Pts',(107.3,-1.2490009027033E-15,-11.59764));
#52988=CARTESIAN_POINT('Ctrl Pts',(107.3,0.276953548632659,-11.59764));
#52989=CARTESIAN_POINT('Ctrl Pts',(107.355486366965,0.571913365577543,-11.5867146442773));
#52990=CARTESIAN_POINT('Ctrl Pts',(107.491919613987,0.900866393499067,-11.5627453043894));
#52991=CARTESIAN_POINT('Ctrl Pts',(107.518478464707,0.957861594797325,-11.5581517426463));
#52992=CARTESIAN_POINT('Ctrl Pts',(107.547344722949,1.01347785817219,-11.5532729648613));
#52993=CARTESIAN_POINT('',(107.499276121999,-0.914933857717795,-11.5614942635285));
#52994=CARTESIAN_POINT('Ctrl Pts',(107.499276121999,-0.914933857717795,
-11.5614942635285));
#52995=CARTESIAN_POINT('Ctrl Pts',(107.488376247984,-0.891098650368292,
-11.563380493605));
#52996=CARTESIAN_POINT('Ctrl Pts',(107.4778971503,-0.867056951964309,-11.565208847591));
#52997=CARTESIAN_POINT('Ctrl Pts',(107.355486366965,-0.571913365577543,
-11.5867146442773));
#52998=CARTESIAN_POINT('Ctrl Pts',(107.3,-0.27695354863266,-11.59764));
#52999=CARTESIAN_POINT('Ctrl Pts',(107.3,4.85722573273506E-16,-11.59764));
#53000=CARTESIAN_POINT('Ctrl Pts',(107.068507977483,-11.5985329378162,-8.63915123330145E-5));
#53001=CARTESIAN_POINT('Ctrl Pts',(107.070148102946,-11.5985543598099,-0.0659446921696183));
#53002=CARTESIAN_POINT('Ctrl Pts',(107.119104647089,-11.5821690115654,-2.03175412121691));
#53003=CARTESIAN_POINT('Ctrl Pts',(107.215377609914,-10.5467853781223,-5.88028127277808));
#53004=CARTESIAN_POINT('Ctrl Pts',(107.357326865957,-6.5216081564048,-10.1627828959428));
#53005=CARTESIAN_POINT('Ctrl Pts',(107.451959703319,-2.80945746568101,-11.4115686783349));
#53006=CARTESIAN_POINT('Ctrl Pts',(107.499276121999,-0.914933857717795,
-11.5614942635285));
#53007=CARTESIAN_POINT('Origin',(93.0806848796603,0.,0.));
#53008=CARTESIAN_POINT('',(104.873542022517,-11.5970620128151,-0.000217152463837714));
#53009=CARTESIAN_POINT('',(105.254222263197,-11.5979149765058,0.000262464412231905));
#53010=CARTESIAN_POINT('',(93.0806848796603,-11.59764,-5.19855242766535E-13));
#53011=CARTESIAN_POINT('Ctrl Pts',(104.873542022517,-11.5970620128151,-0.000217152463837314));
#53012=CARTESIAN_POINT('Ctrl Pts',(104.889877746662,-11.5975244094225,-0.656419016915337));
#53013=CARTESIAN_POINT('Ctrl Pts',(104.95330527189,-11.3847135734158,-3.20398978174987));
#53014=CARTESIAN_POINT('Ctrl Pts',(105.063824598201,-9.54321881653396,-7.39097662401987));
#53015=CARTESIAN_POINT('Ctrl Pts',(105.20510000145,-4.95004576133935,-11.0089330909609));
#53016=CARTESIAN_POINT('Ctrl Pts',(105.346375404699,0.80460272604254,-12.0437608442455));
#53017=CARTESIAN_POINT('Ctrl Pts',(105.487650807948,6.3704597694178,-10.2526485946914));
#53018=CARTESIAN_POINT('Ctrl Pts',(105.628926211197,10.4415563792162,-6.05586171641488));
#53019=CARTESIAN_POINT('Ctrl Pts',(105.770201614447,12.062653180839,-0.438131499218847));
#53020=CARTESIAN_POINT('Ctrl Pts',(105.911477017696,10.8533770682464,5.28240162572942));
#53021=CARTESIAN_POINT('Ctrl Pts',(106.052752420945,7.09747185328678,9.76347550654746));
#53022=CARTESIAN_POINT('Ctrl Pts',(106.194027824194,1.67622047878578,11.9536541207404));
#53023=CARTESIAN_POINT('Ctrl Pts',(106.335303227443,-4.13833793915172,11.3390350829177));
#53024=CARTESIAN_POINT('Ctrl Pts',(106.476578630693,-8.98187994449148,8.0638328962862));
#53025=CARTESIAN_POINT('Ctrl Pts',(106.594086800479,-11.2576257684445,3.76584875965195));
#53026=CARTESIAN_POINT('Ctrl Pts',(106.664503169183,-11.5967538507156,0.937026307393627));
#53027=CARTESIAN_POINT('Ctrl Pts',(106.687827736803,-11.5967315487946,7.87168637238211E-6));
#53028=CARTESIAN_POINT('Ctrl Pts',(105.254222263197,-11.5979149765058,0.000262464412231628));
#53029=CARTESIAN_POINT('Ctrl Pts',(105.292827269251,-11.596406322082,-1.55016204041523));
#53030=CARTESIAN_POINT('Ctrl Pts',(105.378748693986,-10.8995437237543,-5.00218789188436));
#53031=CARTESIAN_POINT('Ctrl Pts',(105.511986537402,-7.57509950853803,-9.40367293367282));
#53032=CARTESIAN_POINT('Ctrl Pts',(105.653935793445,-2.23922610928576,-11.8657938991006));
#53033=CARTESIAN_POINT('Ctrl Pts',(105.795885049488,3.6269801590525,-11.5176477156709));
#53034=CARTESIAN_POINT('Ctrl Pts',(105.93783430553,8.63418136051829,-8.44168924241129));
#53035=CARTESIAN_POINT('Ctrl Pts',(106.079783561573,11.5964822941979,-3.36641977915706));
#53036=CARTESIAN_POINT('Ctrl Pts',(106.221732817616,11.8123013659403,2.50614254258396));
#53037=CARTESIAN_POINT('Ctrl Pts',(106.363682073658,9.23051857694247,7.78516037256956));
#53038=CARTESIAN_POINT('Ctrl Pts',(106.505631329701,4.46260964811663,11.2203497277713));
#53039=CARTESIAN_POINT('Ctrl Pts',(106.647580585744,-1.36223065258046,11.9981569780826));
#53040=CARTESIAN_POINT('Ctrl Pts',(106.789529841786,-6.86440734641473,9.9343085302927));
#53041=CARTESIAN_POINT('Ctrl Pts',(106.929838972366,-10.6961186798297,5.56875601983415));
#53042=CARTESIAN_POINT('Ctrl Pts',(107.022831684265,-11.597936350978,1.83401905935505));
#53043=CARTESIAN_POINT('Ctrl Pts',(107.068507977483,-11.5985329378162,-8.63915123330145E-5));
#53044=CARTESIAN_POINT('Origin',(93.0806848796603,0.,0.));
#53045=CARTESIAN_POINT('',(103.059256308232,-11.5978818050668,-0.000259090622128178));
#53046=CARTESIAN_POINT('',(103.439936548911,-11.5968529998687,0.000153614214355446));
#53047=CARTESIAN_POINT('',(93.0806848796603,-11.59764,-5.19855242766535E-13));
#53048=CARTESIAN_POINT('Ctrl Pts',(103.059256308232,-11.5978818050668,-0.000259090622127499));
#53049=CARTESIAN_POINT('Ctrl Pts',(103.068160523058,-11.5982264103411,-0.357866351962969));
#53050=CARTESIAN_POINT('Ctrl Pts',(103.124156538968,-11.4961896948955,-2.60655846572717));
#53051=CARTESIAN_POINT('Ctrl Pts',(103.227244355961,-10.0848767600063,-6.63285923053644));
#53052=CARTESIAN_POINT('Ctrl Pts',(103.36851975921,-5.7844519333586,-10.5943228508145));
#53053=CARTESIAN_POINT('Ctrl Pts',(103.50979516246,-0.126767166023071,-12.0699416287838));
#53054=CARTESIAN_POINT('Ctrl Pts',(103.651070565709,5.56066216453452,-10.7134773593142));
#53055=CARTESIAN_POINT('Ctrl Pts',(103.792345968958,9.94334143638835,-6.84320991319397));
#53056=CARTESIAN_POINT('Ctrl Pts',(103.933621372207,11.992921710502,-1.36725626068703));
#53057=CARTESIAN_POINT('Ctrl Pts',(104.074896775456,11.2284908393957,4.42950948822145));
#53058=CARTESIAN_POINT('Ctrl Pts',(104.216172178705,7.82941437242525,9.18693808738774));
#53059=CARTESIAN_POINT('Ctrl Pts',(104.357447581955,2.59324934302537,11.7887496657387));
#53060=CARTESIAN_POINT('Ctrl Pts',(104.498722985204,-3.25139398131772,11.6244568911889));
#53061=CARTESIAN_POINT('Ctrl Pts',(104.639998388453,-8.33313239206491,8.73260931064738));
#53062=CARTESIAN_POINT('Ctrl Pts',(104.764938067557,-11.0980767761605,4.36306161391605));
#53063=CARTESIAN_POINT('Ctrl Pts',(104.842785945579,-11.5961914358203,1.23524659872623));
#53064=CARTESIAN_POINT('Ctrl Pts',(104.873542022517,-11.5970620128151,-0.000217152463837314));
#53065=CARTESIAN_POINT('Ctrl Pts',(103.439936548911,-11.5968529998687,0.000153614214355169));
#53066=CARTESIAN_POINT('Ctrl Pts',(103.468190016876,-11.5963058546535,-1.1348392538219));
#53067=CARTESIAN_POINT('Ctrl Pts',(103.543759903522,-11.1534213600585,-4.17103610100268));
#53068=CARTESIAN_POINT('Ctrl Pts',(103.666646208848,-8.54072618632016,-8.53622829798181));
#53069=CARTESIAN_POINT('Ctrl Pts',(103.808595464891,-3.49996651231003,-11.5568781146813));
#53070=CARTESIAN_POINT('Ctrl Pts',(103.950544720934,2.36971705558015,-11.8404239122457));
#53071=CARTESIAN_POINT('Ctrl Pts',(104.092493976976,7.67816237096933,-9.3197113662083));
#53072=CARTESIAN_POINT('Ctrl Pts',(104.234443233019,11.168129644454,-4.59174014842598));
#53073=CARTESIAN_POINT('Ctrl Pts',(104.376392489061,12.0130631783326,1.22372808128535));
#53074=CARTESIAN_POINT('Ctrl Pts',(104.518341745104,10.0128508883889,6.74937141017876));
#53075=CARTESIAN_POINT('Ctrl Pts',(104.660291001147,5.64121838056578,10.6765093795372));
#53076=CARTESIAN_POINT('Ctrl Pts',(104.802240257189,-0.0664671110029323,
12.0750478032933));
#53077=CARTESIAN_POINT('Ctrl Pts',(104.944189513232,-5.75841068985474,10.6137601120454));
#53078=CARTESIAN_POINT('Ctrl Pts',(105.086138769275,-10.0865457254805,6.63873426049027));
#53079=CARTESIAN_POINT('Ctrl Pts',(105.189483019263,-11.4983987440124,2.60007647808839));
#53080=CARTESIAN_POINT('Ctrl Pts',(105.24551085057,-11.5982554119192,0.35012350546277));
#53081=CARTESIAN_POINT('Ctrl Pts',(105.254222263197,-11.5979149765058,0.000262464412231628));
#53082=CARTESIAN_POINT('Origin',(93.0806848796603,0.,0.));
#53083=CARTESIAN_POINT('',(101.244970593946,-11.5985409258756,-5.7588822467809E-5));
#53084=CARTESIAN_POINT('',(101.625650834626,-11.5969301646075,-0.000186353423677899));
#53085=CARTESIAN_POINT('',(93.0806848796603,-11.59764,-5.19855242766535E-13));
#53086=CARTESIAN_POINT('Ctrl Pts',(101.244970593946,-11.5985409258756,-5.75888224674682E-5));
#53087=CARTESIAN_POINT('Ctrl Pts',(101.246443299455,-11.5985577555476,-0.0591940151317032));
#53088=CARTESIAN_POINT('Ctrl Pts',(101.295007806047,-11.5839431479448,-2.00929134158216));
#53089=CARTESIAN_POINT('Ctrl Pts',(101.390664113722,-10.5664450398852,-5.83522065184453));
#53090=CARTESIAN_POINT('Ctrl Pts',(101.531939516971,-6.58439206452233,-10.1165874669912));
#53091=CARTESIAN_POINT('Ctrl Pts',(101.67321492022,-1.05738173003248,-12.0242049514145));
#53092=CARTESIAN_POINT('Ctrl Pts',(101.814490323469,4.71773194782029,-11.1104710118493));
#53093=CARTESIAN_POINT('Ctrl Pts',(101.955765726718,9.38588015038702,-7.58978356998396));
#53094=CARTESIAN_POINT('Ctrl Pts',(102.097041129968,11.8517316992723,-2.28823437722007));
#53095=CARTESIAN_POINT('Ctrl Pts',(102.238316533217,11.5367008329307,3.55022460248401));
#53096=CARTESIAN_POINT('Ctrl Pts',(102.379591936466,8.51470618356667,8.55566125113419));
#53097=CARTESIAN_POINT('Ctrl Pts',(102.520867339715,3.49482655861225,11.5536032544763));
#53098=CARTESIAN_POINT('Ctrl Pts',(102.662142742964,-2.34507683735861,11.8406155018864));
#53099=CARTESIAN_POINT('Ctrl Pts',(102.803418146214,-7.63473296948303,9.34935363120446));
#53100=CARTESIAN_POINT('Ctrl Pts',(102.935789334636,-10.912495171678,4.95964805911867));
#53101=CARTESIAN_POINT('Ctrl Pts',(103.021068721975,-11.5964038933259,1.53341438918833));
#53102=CARTESIAN_POINT('Ctrl Pts',(103.059256308232,-11.5978818050668,-0.000259090622127499));
#53103=CARTESIAN_POINT('Ctrl Pts',(101.625650834626,-11.5969301646075,-0.000186353423678731));
#53104=CARTESIAN_POINT('Ctrl Pts',(101.643552764501,-11.5973545849506,-0.719325510492189));
#53105=CARTESIAN_POINT('Ctrl Pts',(101.708771113057,-11.3573577041451,-3.33893460572594));
#53106=CARTESIAN_POINT('Ctrl Pts',(101.821305880294,-9.40766205636401,-7.57014477921035));
#53107=CARTESIAN_POINT('Ctrl Pts',(101.963255136337,-4.72026363022087,-11.1144189504522));
#53108=CARTESIAN_POINT('Ctrl Pts',(102.105204392379,1.08507100893144,-12.0263800975411));
#53109=CARTESIAN_POINT('Ctrl Pts',(102.247153648422,6.63341996474086,-10.0900414724784));
#53110=CARTESIAN_POINT('Ctrl Pts',(102.389102904465,10.610725229854,-5.76400099249621));
#53111=CARTESIAN_POINT('Ctrl Pts',(102.531052160507,12.0750111151176,-0.0728279804925511));
#53112=CARTESIAN_POINT('Ctrl Pts',(102.67300141655,10.6794795716148,5.63559344030584));
#53113=CARTESIAN_POINT('Ctrl Pts',(102.814950672592,6.75464503055027,10.0092940738206));
#53114=CARTESIAN_POINT('Ctrl Pts',(102.956899928635,1.23005613734974,12.0124168777114));
#53115=CARTESIAN_POINT('Ctrl Pts',(103.098849184678,-4.58585637836471,11.1705469258209));
#53116=CARTESIAN_POINT('Ctrl Pts',(103.24079844072,-9.31566538066349,7.68307073119021));
#53117=CARTESIAN_POINT('Ctrl Pts',(103.354494228798,-11.3368967970257,3.4322783363807));
#53118=CARTESIAN_POINT('Ctrl Pts',(103.420873598195,-11.59722216525,0.765946795195559));
#53119=CARTESIAN_POINT('Ctrl Pts',(103.439936548911,-11.5968529998687,0.000153614214355169));
#53120=CARTESIAN_POINT('Origin',(93.0806848796603,0.,0.));
#53121=CARTESIAN_POINT('',(99.4306848796602,-11.5982123705775,0.000204477995816285));
#53122=CARTESIAN_POINT('',(99.8113651203399,-11.5980517843054,-0.000244059920104789));
#53123=CARTESIAN_POINT('',(93.0806848796603,-11.59764,-5.19855242766535E-13));
#53124=CARTESIAN_POINT('Ctrl Pts',(99.4306848796602,-11.5982123705775,0.000204477995815917));
#53125=CARTESIAN_POINT('Ctrl Pts',(99.4718178769342,-11.5968382129007,-1.6516251690263));
#53126=CARTESIAN_POINT('Ctrl Pts',(99.5600426752913,-10.8315259674307,-5.19581284549921));
#53127=CARTESIAN_POINT('Ctrl Pts',(99.6953592747313,-7.34509979707817,-9.57857347461386));
#53128=CARTESIAN_POINT('Ctrl Pts',(99.8366346779806,-1.98169599765362,-11.9068233298798));
#53129=CARTESIAN_POINT('Ctrl Pts',(99.9779100812298,3.84669162792076,-11.4412641065812));
#53130=CARTESIAN_POINT('Ctrl Pts',(100.119185484479,8.77249409748291,-8.29113430998339));
#53131=CARTESIAN_POINT('Ctrl Pts',(100.260460887728,11.6399244073961,-3.19557829300717));
#53132=CARTESIAN_POINT('Ctrl Pts',(100.401736290977,11.7761706236747,2.64978608169418));
#53133=CARTESIAN_POINT('Ctrl Pts',(100.543011694227,9.14926402506894,7.8734064188378));
#53134=CARTESIAN_POINT('Ctrl Pts',(100.684287097476,4.37558022249231,11.2496159291403));
#53135=CARTESIAN_POINT('Ctrl Pts',(100.825562500725,-1.42478680291599,11.9862230666236));
#53136=CARTESIAN_POINT('Ctrl Pts',(100.966837903974,-6.89084280389226,9.91039082421449));
#53137=CARTESIAN_POINT('Ctrl Pts',(101.106640601714,-10.699910676898,5.55507077934471));
#53138=CARTESIAN_POINT('Ctrl Pts',(101.199351498372,-11.5980196034472,1.83177523010779));
#53139=CARTESIAN_POINT('Ctrl Pts',(101.244970593946,-11.5985409258756,-5.75888224674682E-5));
#53140=CARTESIAN_POINT('Ctrl Pts',(99.8113651203399,-11.5980517843054,-0.000244059920105136));
#53141=CARTESIAN_POINT('Ctrl Pts',(99.8189155121257,-11.5983353502102,-0.303466742622632));
#53142=CARTESIAN_POINT('Ctrl Pts',(99.8737823225923,-11.5136117348972,-2.50675216138025));
#53143=CARTESIAN_POINT('Ctrl Pts',(99.9759655517397,-10.1658893729505,-6.51658580867914));
#53144=CARTESIAN_POINT('Ctrl Pts',(100.117914807782,-5.88601658741872,-10.5435291092497));
#53145=CARTESIAN_POINT('Ctrl Pts',(100.259864063825,-0.212113381356825,
-12.0733676022228));
#53146=CARTESIAN_POINT('Ctrl Pts',(100.401813319868,5.51202626250981,-10.7437779121853));
#53147=CARTESIAN_POINT('Ctrl Pts',(100.54376257591,9.93071048086492,-6.8696569557873));
#53148=CARTESIAN_POINT('Ctrl Pts',(100.685711831953,11.997428424203,-1.36854249151505));
#53149=CARTESIAN_POINT('Ctrl Pts',(100.827661087996,11.2227034420802,4.45669437992771));
#53150=CARTESIAN_POINT('Ctrl Pts',(100.969610344038,7.7900195897285,9.22641816397909));
#53151=CARTESIAN_POINT('Ctrl Pts',(101.111559600081,2.51236569298111,11.8109786203214));
#53152=CARTESIAN_POINT('Ctrl Pts',(101.253508856124,-3.3603110263314,11.5982544872611));
#53153=CARTESIAN_POINT('Ctrl Pts',(101.395458112166,-8.43713953088349,8.63862685161016));
#53154=CARTESIAN_POINT('Ctrl Pts',(101.519505438333,-11.1274784823704,4.26432569210168));
#53155=CARTESIAN_POINT('Ctrl Pts',(101.59623634582,-11.5962328036236,1.18142427920913));
#53156=CARTESIAN_POINT('Ctrl Pts',(101.625650834626,-11.5969301646075,-0.000186353423678731));
#53157=CARTESIAN_POINT('Origin',(93.0806848796603,0.,0.));
#53158=CARTESIAN_POINT('',(97.6163991653745,-11.5973549676912,0.000264155725229257));
#53159=CARTESIAN_POINT('',(97.9970794060541,-11.5984942842416,0.000109136483176162));
#53160=CARTESIAN_POINT('',(93.0806848796603,-11.59764,-5.19855242766535E-13));
#53161=CARTESIAN_POINT('Ctrl Pts',(97.6163991653745,-11.5973549676912,0.00026415572522899));
#53162=CARTESIAN_POINT('Ctrl Pts',(97.6501006533306,-11.5961500955102,-1.35341785052988));
#53163=CARTESIAN_POINT('Ctrl Pts',(97.7308939423697,-11.0276899039031,-4.59961573681585));
#53164=CARTESIAN_POINT('Ctrl Pts',(97.8587790324919,-8.06204243838756,-8.9834859317315));
#53165=CARTESIAN_POINT('Ctrl Pts',(98.0000544357412,-2.89420258720722,-11.7184964778204));
#53166=CARTESIAN_POINT('Ctrl Pts',(98.1413298389903,2.95273122806244,-11.7038855003407));
#53167=CARTESIAN_POINT('Ctrl Pts',(98.2826052422396,8.10683806242452,-8.94308328046984));
#53168=CARTESIAN_POINT('Ctrl Pts',(98.4238806454887,11.3587618711925,-4.08388166193566));
#53169=CARTESIAN_POINT('Ctrl Pts',(98.5651560487379,11.9454733539258,1.73355907649387));
#53170=CARTESIAN_POINT('Ctrl Pts',(98.706431451987,9.7293069528249,7.14423874107845));
#53171=CARTESIAN_POINT('Ctrl Pts',(98.8477068552363,5.23026245722293,10.8785989620564));
#53172=CARTESIAN_POINT('Ctrl Pts',(98.9889822584854,-0.496007327832227,
12.0604120000411));
#53173=CARTESIAN_POINT('Ctrl Pts',(99.1302576617347,-6.10589428573641,10.4123780084834));
#53174=CARTESIAN_POINT('Ctrl Pts',(99.2715330649838,-10.2830982833774,6.32119059473821));
#53175=CARTESIAN_POINT('Ctrl Pts',(99.371675470959,-11.5337740761537,2.36981230115211));
#53176=CARTESIAN_POINT('Ctrl Pts',(99.4247260758512,-11.59841144034,0.23949967759091));
#53177=CARTESIAN_POINT('Ctrl Pts',(99.4306848796602,-11.5982123705775,0.000204477995815917));
#53178=CARTESIAN_POINT('Ctrl Pts',(97.9970794060541,-11.5984942842416,0.000109136483176196));
#53179=CARTESIAN_POINT('Ctrl Pts',(98.0415946784313,-11.5976002818738,-1.7874203035197));
#53180=CARTESIAN_POINT('Ctrl Pts',(98.1334263694893,-10.7312077943355,-5.47579749744129));
#53181=CARTESIAN_POINT('Ctrl Pts',(98.2725744792281,-6.98375473307958,-9.85080540269698));
#53182=CARTESIAN_POINT('Ctrl Pts',(98.4145237352708,-1.50684673412838,-11.9808434723489));
#53183=CARTESIAN_POINT('Ctrl Pts',(98.5564729913134,4.32693932863066,-11.2733665501931));
#53184=CARTESIAN_POINT('Ctrl Pts',(98.6984222473561,9.13594318590594,-7.89593182926991));
#53185=CARTESIAN_POINT('Ctrl Pts',(98.8403715033986,11.781211598614,-2.64844305476444));
#53186=CARTESIAN_POINT('Ctrl Pts',(98.9823207594414,11.6362453734974,3.22629678599122));
#53187=CARTESIAN_POINT('Ctrl Pts',(99.124270015484,8.73537797318143,8.33692803205455));
#53188=CARTESIAN_POINT('Ctrl Pts',(99.2662192715265,3.76564405694391,11.4730607154675));
#53189=CARTESIAN_POINT('Ctrl Pts',(99.4081685275693,-2.0959362022484,11.8919404968782));
#53190=CARTESIAN_POINT('Ctrl Pts',(99.5501177836118,-7.46111982681854,9.49436086710135));
#53191=CARTESIAN_POINT('Ctrl Pts',(99.6845166478687,-10.8678430079567,5.09529409224268));
#53192=CARTESIAN_POINT('Ctrl Pts',(99.7715990934448,-11.59655831354,1.59675404265655));
#53193=CARTESIAN_POINT('Ctrl Pts',(99.8113651203399,-11.5980517843054,-0.000244059920105136));
#53194=CARTESIAN_POINT('Origin',(93.0806848796603,0.,0.));
#53195=CARTESIAN_POINT('',(115.759256308232,-11.5966977159097,-2.20020729888378E-5));
#53196=CARTESIAN_POINT('',(116.139936548911,-11.5978562621874,0.000265160474589299));
#53197=CARTESIAN_POINT('',(93.0806848796603,-11.59764,-5.19855242766535E-13));
#53198=CARTESIAN_POINT('',(117.38636,-9.24570028839849,7.00280438584369));
#53199=CARTESIAN_POINT('Ctrl Pts',(115.759256308232,-11.5966977159097,-2.20020729886639E-5));
#53200=CARTESIAN_POINT('Ctrl Pts',(115.782472788843,-11.5967602494871,-0.932708015072538));
#53201=CARTESIAN_POINT('Ctrl Pts',(115.853334649975,-11.2572698648965,-3.77942835970487));
#53202=CARTESIAN_POINT('Ctrl Pts',(115.971841891627,-8.95294307109407,-8.11300498914965));
#53203=CARTESIAN_POINT('Ctrl Pts',(116.11477803319,-4.0242321603504,-11.3921725585846));
#53204=CARTESIAN_POINT('Ctrl Pts',(116.257714174752,1.87059427966267,-11.9363694039364));
#53205=CARTESIAN_POINT('Ctrl Pts',(116.400650316314,7.31633898196617,-9.61494819743955));
#53206=CARTESIAN_POINT('Ctrl Pts',(116.543586457876,11.005616292,-4.98522204048877));
#53207=CARTESIAN_POINT('Ctrl Pts',(116.686522599438,12.0527268155209,0.841327506667632));
#53208=CARTESIAN_POINT('Ctrl Pts',(116.829458741,10.2062813712173,6.46589893037503));
#53209=CARTESIAN_POINT('Ctrl Pts',(116.972394882562,5.9095743448429,10.5381658364625));
#53210=CARTESIAN_POINT('Ctrl Pts',(117.115331024124,0.194114641227306,12.0805020392623));
#53211=CARTESIAN_POINT('Ctrl Pts',(117.253319396603,-5.36846226369204,10.7695908115406));
#53212=CARTESIAN_POINT('Ctrl Pts',(117.343662388562,-8.20939703265164,8.36879965219385));
#53213=CARTESIAN_POINT('Ctrl Pts',(117.38636,-9.24570028839849,7.00280438584369));
#53214=CARTESIAN_POINT('',(117.38636,4.47152467205382,10.7009682121205));
#53215=CARTESIAN_POINT('Origin',(117.38636,0.,0.));
#53216=CARTESIAN_POINT('Ctrl Pts',(116.139936548911,-11.5978562621874,0.000265160474589889));
#53217=CARTESIAN_POINT('Ctrl Pts',(116.177899585767,-11.5963703069285,-1.52440435616002));
#53218=CARTESIAN_POINT('Ctrl Pts',(116.263051553478,-10.917763149328,-4.94555756957596));
#53219=CARTESIAN_POINT('Ctrl Pts',(116.395392452043,-7.64837610766902,-9.34078625853751));
#53220=CARTESIAN_POINT('Ctrl Pts',(116.536959244609,-2.34918804318456,-11.8418520279979));
#53221=CARTESIAN_POINT('Ctrl Pts',(116.678526037174,3.50341987815323,-11.5530757135873));
#53222=CARTESIAN_POINT('Ctrl Pts',(116.820092829739,8.53070918247288,-8.54259995247553));
#53223=CARTESIAN_POINT('Ctrl Pts',(116.961659622304,11.5481555073598,-3.51942696985816));
#53224=CARTESIAN_POINT('Ctrl Pts',(117.103226414869,11.8451994508802,2.33252276799301));
#53225=CARTESIAN_POINT('Ctrl Pts',(117.244793207435,9.35114240419514,7.63559939886844));
#53226=CARTESIAN_POINT('Ctrl Pts',(117.339171069145,6.22031361682587,9.97021630652136));
#53227=CARTESIAN_POINT('Ctrl Pts',(117.38636,4.47152467205382,10.7009682121205));
#53228=CARTESIAN_POINT('Origin',(93.0806848796603,0.,0.));
#53229=CARTESIAN_POINT('',(113.944970593946,-11.5979544128403,-0.000269279950390758));
#53230=CARTESIAN_POINT('',(114.325650834626,-11.5969419105478,0.000182072225077823));
#53231=CARTESIAN_POINT('',(93.0806848796603,-11.59764,-5.19855242766535E-13));
#53232=CARTESIAN_POINT('Ctrl Pts',(113.944970593946,-11.5979544128403,-0.000269279950390472));
#53233=CARTESIAN_POINT('Ctrl Pts',(113.95355903255,-11.5982957222328,-0.345189041569635));
#53234=CARTESIAN_POINT('Ctrl Pts',(114.009792851675,-11.4995210665118,-2.60339725427472));
#53235=CARTESIAN_POINT('Ctrl Pts',(114.11367205132,-10.078006847733,-6.66406913873543));
#53236=CARTESIAN_POINT('Ctrl Pts',(114.256608192883,-5.7025528495123,-10.6516163368671));
#53237=CARTESIAN_POINT('Ctrl Pts',(114.399544334445,0.0419388972008348,
-12.0819816539827));
#53238=CARTESIAN_POINT('Ctrl Pts',(114.542480476007,5.77636218068765,-10.6117708005521));
#53239=CARTESIAN_POINT('Ctrl Pts',(114.685416617569,10.1240279793146,-6.59394396708397));
#53240=CARTESIAN_POINT('Ctrl Pts',(114.828352759131,12.0411724308134,-0.993079077887869));
#53241=CARTESIAN_POINT('Ctrl Pts',(114.971288900693,11.0675379662367,4.84619881277042));
#53242=CARTESIAN_POINT('Ctrl Pts',(115.114225042255,7.43686942972829,9.52202775941664));
#53243=CARTESIAN_POINT('Ctrl Pts',(115.257161183817,2.02079789647468,11.9118602837624));
#53244=CARTESIAN_POINT('Ctrl Pts',(115.400097325379,-3.88041576111888,11.4419584473181));
#53245=CARTESIAN_POINT('Ctrl Pts',(115.543033466941,-8.85004039162967,8.22513371169866));
#53246=CARTESIAN_POINT('Ctrl Pts',(115.662753127892,-11.23290225591,3.87689112845648));
#53247=CARTESIAN_POINT('Ctrl Pts',(115.734827408322,-11.5966319166816,0.981371071238124));
#53248=CARTESIAN_POINT('Ctrl Pts',(115.759256308232,-11.5966977159097,-2.20020729886639E-5));
#53249=CARTESIAN_POINT('Ctrl Pts',(114.325650834626,-11.5969419105478,0.000182072225077753));
#53250=CARTESIAN_POINT('Ctrl Pts',(114.354919675127,-11.5962607053732,-1.17557795589793));
#53251=CARTESIAN_POINT('Ctrl Pts',(114.431377446484,-11.1315096647659,-4.24749348564229));
#53252=CARTESIAN_POINT('Ctrl Pts',(114.555024148696,-8.45978526537628,-8.6127818545234));
#53253=CARTESIAN_POINT('Ctrl Pts',(114.696590941261,-3.40781807628825,-11.581655924795));
#53254=CARTESIAN_POINT('Ctrl Pts',(114.838157733826,2.44699275634759,-11.8220220132816));
#53255=CARTESIAN_POINT('Ctrl Pts',(114.979724526391,7.72531959196485,-9.2772525651793));
#53256=CARTESIAN_POINT('Ctrl Pts',(115.121291318956,11.1836479525214,-4.54686667674157));
#53257=CARTESIAN_POINT('Ctrl Pts',(115.262858111522,12.0072345239343,1.25470992130988));
#53258=CARTESIAN_POINT('Ctrl Pts',(115.404424904087,10.0020516002354,6.76069092494371));
#53259=CARTESIAN_POINT('Ctrl Pts',(115.545991696652,5.64049766960815,10.6739292014239));
#53260=CARTESIAN_POINT('Ctrl Pts',(115.687558489217,-0.0498940161182073,
12.0725095394857));
#53261=CARTESIAN_POINT('Ctrl Pts',(115.829125281783,-5.72853146574744,10.6269426623712));
#53262=CARTESIAN_POINT('Ctrl Pts',(115.970692074348,-10.0575907787097,6.67778673879954));
#53263=CARTESIAN_POINT('Ctrl Pts',(116.074295830057,-11.4917013921148,2.63631752302503));
#53264=CARTESIAN_POINT('Ctrl Pts',(116.130710654912,-11.5982173836055,0.370795036632186));
#53265=CARTESIAN_POINT('Ctrl Pts',(116.139936548911,-11.5978562621874,0.000265160474589889));
#53266=CARTESIAN_POINT('Origin',(93.0806848796603,0.,0.));
#53267=CARTESIAN_POINT('',(112.13068487966,-11.5982247539793,0.000228379848985116));
#53268=CARTESIAN_POINT('',(112.51136512034,-11.5967929078458,-0.000103121459272826));
#53269=CARTESIAN_POINT('',(93.0806848796603,-11.59764,-5.19855242766535E-13));
#53270=CARTESIAN_POINT('Ctrl Pts',(112.13068487966,-11.5982247539793,0.000228379848985077));
#53271=CARTESIAN_POINT('Ctrl Pts',(112.172290656778,-11.596775601192,-1.67056794358247));
#53272=CARTESIAN_POINT('Ctrl Pts',(112.261541814416,-10.8135367102492,-5.25606952472166));
#53273=CARTESIAN_POINT('Ctrl Pts',(112.398438352575,-7.24939531411746,-9.66549613681094));
#53274=CARTESIAN_POINT('Ctrl Pts',(112.541374494138,-1.78769147784434,-11.9490739890003));
#53275=CARTESIAN_POINT('Ctrl Pts',(112.6843106357,4.1032269254419,-11.363957802295));
#53276=CARTESIAN_POINT('Ctrl Pts',(112.827246777262,9.00904847698782,-8.05065674001605));
#53277=CARTESIAN_POINT('Ctrl Pts',(112.970182918824,11.7520346070574,-2.80459235140811));
#53278=CARTESIAN_POINT('Ctrl Pts',(113.113119060386,11.6736528323709,3.11478061972093));
#53279=CARTESIAN_POINT('Ctrl Pts',(113.256055201948,8.79272593142687,8.28637530125792));
#53280=CARTESIAN_POINT('Ctrl Pts',(113.39899134351,3.80088861740511,11.4686216793657));
#53281=CARTESIAN_POINT('Ctrl Pts',(113.541927485072,-2.10344490785294,11.897544267814));
#53282=CARTESIAN_POINT('Ctrl Pts',(113.684863626634,-7.50279504034574,9.47016927888733));
#53283=CARTESIAN_POINT('Ctrl Pts',(113.819211329592,-10.8847189596875,5.05170665773232));
#53284=CARTESIAN_POINT('Ctrl Pts',(113.905913652029,-11.5964022679471,1.56829419431985));
#53285=CARTESIAN_POINT('Ctrl Pts',(113.944970593946,-11.5979544128403,-0.000269279950390472));
#53286=CARTESIAN_POINT('Ctrl Pts',(112.51136512034,-11.5967929078458,-0.000103121459272826));
#53287=CARTESIAN_POINT('Ctrl Pts',(112.531939764487,-11.5970590783192,-0.826638577717111));
#53288=CARTESIAN_POINT('Ctrl Pts',(112.59970333949,-11.3098683964611,-3.54869026150752));
#53289=CARTESIAN_POINT('Ctrl Pts',(112.714655845348,-9.20221848328371,-7.81454784931888));
#53290=CARTESIAN_POINT('Ctrl Pts',(112.856222637913,-4.43865660418402,-11.2270344946451));
#53291=CARTESIAN_POINT('Ctrl Pts',(112.997789430478,1.37060254033464,-11.9945582342283));
#53292=CARTESIAN_POINT('Ctrl Pts',(113.139356223043,6.85696329237368,-9.9362987275659));
#53293=CARTESIAN_POINT('Ctrl Pts',(113.280923015609,10.7279004735232,-5.53715895830823));
#53294=CARTESIAN_POINT('Ctrl Pts',(113.422489808174,12.0714648968156,0.166473261964394));
#53295=CARTESIAN_POINT('Ctrl Pts',(113.564056600739,10.5711278304476,5.83088624039759));
#53296=CARTESIAN_POINT('Ctrl Pts',(113.705623393304,6.58035185125043,10.1216079525872));
#53297=CARTESIAN_POINT('Ctrl Pts',(113.847190185869,1.03931892093069,12.0277925731204));
#53298=CARTESIAN_POINT('Ctrl Pts',(113.988756978435,-4.74656586578709,11.1003644305775));
#53299=CARTESIAN_POINT('Ctrl Pts',(114.130323771,-9.41421307630654,7.55781517133264));
#53300=CARTESIAN_POINT('Ctrl Pts',(114.242621723064,-11.3574903143052,3.33527400553394));
#53301=CARTESIAN_POINT('Ctrl Pts',(114.307730744272,-11.5973589840659,0.720050901223368));
#53302=CARTESIAN_POINT('Ctrl Pts',(114.325650834626,-11.5969419105478,0.000182072225077753));
#53303=CARTESIAN_POINT('Origin',(117.798242418585,0.,-8.05687251955465E-17));
#53304=CARTESIAN_POINT('',(118.,-3.4268292682927,-4.19665549463912E-16));
#53305=CARTESIAN_POINT('Origin',(118.,0.,0.));
#53306=CARTESIAN_POINT('',(117.596484837171,-2.63157427110059,0.));
#53307=CARTESIAN_POINT('',(117.798242418585,-3.02920176969664,-5.32107675514142E-16));
#53308=CARTESIAN_POINT('Origin',(117.596484837171,0.,-1.61137450391093E-16));
#53309=CARTESIAN_POINT('Origin',(116.05,0.,0.));
#53310=CARTESIAN_POINT('',(114.,0.,0.));
#53311=CARTESIAN_POINT('',(116.05,-1.5,-1.83697019872103E-16));
#53312=CARTESIAN_POINT('Origin',(118.,0.,0.));
#53313=CARTESIAN_POINT('',(118.,-12.,-1.46957615897682E-15));
#53314=CARTESIAN_POINT('Origin',(118.,0.,0.));
#53315=CARTESIAN_POINT('Origin',(94.75,4.6,-12.25));
#53316=CARTESIAN_POINT('',(95.,-2.7,-12.));
#53317=CARTESIAN_POINT('',(94.5,-2.7,-12.5));
#53318=CARTESIAN_POINT('',(99.7500000000001,-2.7,-7.24999999999999));
#53319=CARTESIAN_POINT('',(94.5,2.7,-12.5));
#53320=CARTESIAN_POINT('',(94.5,4.6,-12.5));
#53321=CARTESIAN_POINT('',(95.,2.7,-12.));
#53322=CARTESIAN_POINT('',(100.625,2.7,-6.375));
#53323=CARTESIAN_POINT('',(95.,4.6,-12.));
#53324=CARTESIAN_POINT('Origin',(118.5,-2.7,-12.5));
#53325=CARTESIAN_POINT('',(86.,-2.7,-12.5));
#53326=CARTESIAN_POINT('',(118.5,-2.7,-12.5));
#53327=CARTESIAN_POINT('',(86.,2.7,-12.5));
#53328=CARTESIAN_POINT('',(86.,-2.7,-12.5));
#53329=CARTESIAN_POINT('',(118.5,2.7,-12.5));
#53330=CARTESIAN_POINT('Origin',(-22.,-41.9267766952966,53.8232233047034));
#53331=CARTESIAN_POINT('',(-14.3232233047034,-41.9267766952966,53.8232233047034));
#53332=CARTESIAN_POINT('',(-14.5,-41.5,54.));
#53333=CARTESIAN_POINT('',(-24.5071980214169,-17.3404868153423,64.0071980214168));
#53334=CARTESIAN_POINT('',(-21.5,-41.5,54.));
#53335=CARTESIAN_POINT('',(-22.,-41.5,54.));
#53336=CARTESIAN_POINT('',(-21.6767766952966,-41.9267766952966,53.8232233047034));
#53337=CARTESIAN_POINT('',(-12.0037603021723,-18.5740493299586,63.4962396978277));
#53338=CARTESIAN_POINT('',(-21.5,-42.3535533905933,53.6464466094067));
#53339=CARTESIAN_POINT('',(-21.0638697904486,-43.4064648574528,53.2103163998554));
#53340=CARTESIAN_POINT('',(-14.5,-42.3535533905933,53.6464466094067));
#53341=CARTESIAN_POINT('',(-22.,-42.3535533905933,53.6464466094067));
#53342=CARTESIAN_POINT('',(-15.4470885331405,-44.6400273720691,52.6993580762662));
#53343=CARTESIAN_POINT('Origin',(-22.,-42.,54.));
#53344=CARTESIAN_POINT('',(-21.5,-53.6464466094067,42.3535533905933));
#53345=CARTESIAN_POINT('',(-21.5,-45.,51.));
#53346=CARTESIAN_POINT('',(-14.5,-53.6464466094067,42.3535533905933));
#53347=CARTESIAN_POINT('',(-22.,-53.6464466094067,42.3535533905933));
#53348=CARTESIAN_POINT('',(-14.5,-45.,51.));
#53349=CARTESIAN_POINT('Origin',(-21.75,-44.8232233047034,50.8232233047034));
#53350=CARTESIAN_POINT('',(-22.,-41.7928932188134,53.5));
#53351=CARTESIAN_POINT('',(-22.,-41.7928932188134,53.5));
#53352=CARTESIAN_POINT('',(-22.,-53.5,41.7928932188135));
#53353=CARTESIAN_POINT('',(-22.,-44.6464466094067,50.6464466094067));
#53354=CARTESIAN_POINT('',(-22.,-53.5,41.7928932188135));
#53355=CARTESIAN_POINT('Origin',(-21.75,21.,53.75));
#53356=CARTESIAN_POINT('',(-21.5,41.5,54.));
#53357=CARTESIAN_POINT('',(-21.5,21.,54.));
#53358=CARTESIAN_POINT('',(-21.6767766952966,41.9267766952966,53.8232233047034));
#53359=CARTESIAN_POINT('',(-18.4799635039079,34.2089869322727,57.0200364960921));
#53360=CARTESIAN_POINT('',(-22.,41.7928932188135,53.5));
#53361=CARTESIAN_POINT('',(-22.,41.7928932188135,53.5));
#53362=CARTESIAN_POINT('',(-22.,21.,53.5));
#53363=CARTESIAN_POINT('Origin',(-14.5,41.5,54.));
#53364=CARTESIAN_POINT('',(-14.5,42.3535533905933,53.6464466094067));
#53365=CARTESIAN_POINT('',(-14.,41.7928932188134,53.5));
#53366=CARTESIAN_POINT('',(-14.5,42.3535533905933,53.6464466094067));
#53367=CARTESIAN_POINT('',(-14.5,41.5,54.));
#53368=CARTESIAN_POINT('',(-14.5,41.5,54.));
#53369=CARTESIAN_POINT('',(-14.,41.7928932188134,53.5));
#53370=CARTESIAN_POINT('Origin',(-22.,41.9267766952966,53.8232233047034));
#53371=CARTESIAN_POINT('',(-22.,41.5,54.));
#53372=CARTESIAN_POINT('',(-21.5,42.3535533905933,53.6464466094067));
#53373=CARTESIAN_POINT('',(-22.,42.3535533905933,53.6464466094067));
#53374=CARTESIAN_POINT('',(-19.7554791617946,46.5651992580313,51.9019257712013));
#53375=CARTESIAN_POINT('Origin',(-14.25,21.,53.75));
#53376=CARTESIAN_POINT('',(-14.,-41.7928932188134,53.5));
#53377=CARTESIAN_POINT('',(-7.85670147864286,-39.2482556535607,47.3567014786429));
#53378=CARTESIAN_POINT('',(-14.,21.,53.5));
#53379=CARTESIAN_POINT('',(-14.5,21.,54.));
#53380=CARTESIAN_POINT('Origin',(-14.5,53.6464466094067,42.3535533905933));
#53381=CARTESIAN_POINT('',(-14.5,54.,41.5));
#53382=CARTESIAN_POINT('',(-14.,53.5,41.7928932188135));
#53383=CARTESIAN_POINT('',(-14.5,54.,41.5));
#53384=CARTESIAN_POINT('',(-14.5,53.6464466094067,42.3535533905933));
#53385=CARTESIAN_POINT('',(-14.5,53.6464466094067,42.3535533905933));
#53386=CARTESIAN_POINT('',(-14.,53.5,41.7928932188134));
#53387=CARTESIAN_POINT('Origin',(-22.,53.8232233047034,41.9267766952966));
#53388=CARTESIAN_POINT('',(-21.6767766952966,53.8232233047034,41.9267766952966));
#53389=CARTESIAN_POINT('',(-21.5,53.6464466094067,42.3535533905933));
#53390=CARTESIAN_POINT('',(-21.0638697904486,53.2103163998554,43.4064648574528));
#53391=CARTESIAN_POINT('',(-22.,53.6464466094067,42.3535533905933));
#53392=CARTESIAN_POINT('',(-21.5,54.,41.5));
#53393=CARTESIAN_POINT('',(-22.,54.,41.5));
#53394=CARTESIAN_POINT('',(-12.0037603021723,63.4962396978277,18.5740493299586));
#53395=CARTESIAN_POINT('Origin',(-14.25,50.8232233047034,44.8232233047034));
#53396=CARTESIAN_POINT('',(-14.,50.6464466094067,44.6464466094067));
#53397=CARTESIAN_POINT('',(-14.5,51.,45.));
#53398=CARTESIAN_POINT('Origin',(-14.5,54.,-41.5));
#53399=CARTESIAN_POINT('',(-14.5,53.6464466094067,-42.3535533905933));
#53400=CARTESIAN_POINT('',(-14.,53.5,-41.7928932188134));
#53401=CARTESIAN_POINT('',(-14.5,53.6464466094067,-42.3535533905933));
#53402=CARTESIAN_POINT('',(-14.5,54.,-41.5));
#53403=CARTESIAN_POINT('',(-14.5,54.,-41.5));
#53404=CARTESIAN_POINT('',(-14.,53.5,-41.7928932188134));
#53405=CARTESIAN_POINT('Origin',(-22.,53.8232233047034,-41.9267766952966));
#53406=CARTESIAN_POINT('',(-21.6767766952966,53.8232233047034,-41.9267766952966));
#53407=CARTESIAN_POINT('',(-21.5,54.,-41.5));
#53408=CARTESIAN_POINT('',(-18.4799635039079,57.0200364960921,-34.2089869322727));
#53409=CARTESIAN_POINT('',(-22.,54.,-41.5));
#53410=CARTESIAN_POINT('',(-21.5,53.6464466094067,-42.3535533905933));
#53411=CARTESIAN_POINT('',(-22.,53.6464466094067,-42.3535533905933));
#53412=CARTESIAN_POINT('',(-19.7554791617946,51.9019257712013,-46.5651992580313));
#53413=CARTESIAN_POINT('Origin',(-14.25,53.75,-21.));
#53414=CARTESIAN_POINT('',(-14.,53.5,-21.));
#53415=CARTESIAN_POINT('',(-14.5,54.,-21.));
#53416=CARTESIAN_POINT('Origin',(-14.5,42.3535533905933,-53.6464466094067));
#53417=CARTESIAN_POINT('',(-14.5,41.5,-54.));
#53418=CARTESIAN_POINT('',(-14.,41.7928932188135,-53.5));
#53419=CARTESIAN_POINT('',(-14.5,41.5,-54.));
#53420=CARTESIAN_POINT('',(-14.5,42.3535533905933,-53.6464466094067));
#53421=CARTESIAN_POINT('',(-14.5,42.3535533905933,-53.6464466094067));
#53422=CARTESIAN_POINT('',(-14.,41.7928932188134,-53.5));
#53423=CARTESIAN_POINT('Origin',(-22.,41.9267766952966,-53.8232233047034));
#53424=CARTESIAN_POINT('',(-21.6767766952966,41.9267766952966,-53.8232233047034));
#53425=CARTESIAN_POINT('',(-21.5,42.3535533905933,-53.6464466094067));
#53426=CARTESIAN_POINT('',(-21.0638697904486,43.4064648574528,-53.2103163998554));
#53427=CARTESIAN_POINT('',(-22.,42.3535533905933,-53.6464466094067));
#53428=CARTESIAN_POINT('',(-21.5,41.5,-54.));
#53429=CARTESIAN_POINT('',(-22.,41.5,-54.));
#53430=CARTESIAN_POINT('',(-12.0037603021723,18.5740493299586,-63.4962396978277));
#53431=CARTESIAN_POINT('Origin',(-14.25,44.8232233047034,-50.8232233047034));
#53432=CARTESIAN_POINT('',(-14.,44.6464466094067,-50.6464466094067));
#53433=CARTESIAN_POINT('',(-14.5,45.,-51.));
#53434=CARTESIAN_POINT('Origin',(-14.5,-41.5,-54.));
#53435=CARTESIAN_POINT('',(-14.5,-42.3535533905933,-53.6464466094067));
#53436=CARTESIAN_POINT('',(-14.,-41.7928932188134,-53.5));
#53437=CARTESIAN_POINT('',(-14.5,-42.3535533905933,-53.6464466094067));
#53438=CARTESIAN_POINT('',(-14.5,-41.5,-54.));
#53439=CARTESIAN_POINT('',(-14.5,-41.5,-54.));
#53440=CARTESIAN_POINT('',(-14.,-41.7928932188134,-53.5));
#53441=CARTESIAN_POINT('Origin',(-22.,-41.9267766952966,-53.8232233047034));
#53442=CARTESIAN_POINT('',(-21.6767766952966,-41.9267766952966,-53.8232233047034));
#53443=CARTESIAN_POINT('',(-21.5,-41.5,-54.));
#53444=CARTESIAN_POINT('',(-18.4799635039079,-34.2089869322727,-57.0200364960921));
#53445=CARTESIAN_POINT('',(-22.,-41.5,-54.));
#53446=CARTESIAN_POINT('',(-21.5,-42.3535533905933,-53.6464466094067));
#53447=CARTESIAN_POINT('',(-22.,-42.3535533905933,-53.6464466094067));
#53448=CARTESIAN_POINT('',(-19.7554791617946,-46.5651992580313,-51.9019257712013));
#53449=CARTESIAN_POINT('Origin',(-14.25,-21.,-53.75));
#53450=CARTESIAN_POINT('',(-14.,-21.,-53.5));
#53451=CARTESIAN_POINT('',(-14.5,-21.,-54.));
#53452=CARTESIAN_POINT('Origin',(-14.5,-53.6464466094067,-42.3535533905933));
#53453=CARTESIAN_POINT('',(-14.5,-54.,-41.5));
#53454=CARTESIAN_POINT('',(-14.,-53.5,-41.7928932188135));
#53455=CARTESIAN_POINT('',(-14.5,-54.,-41.5));
#53456=CARTESIAN_POINT('',(-14.5,-53.6464466094067,-42.3535533905933));
#53457=CARTESIAN_POINT('',(-14.5,-53.6464466094067,-42.3535533905933));
#53458=CARTESIAN_POINT('',(-14.,-53.5,-41.7928932188134));
#53459=CARTESIAN_POINT('Origin',(-22.,-53.8232233047034,-41.9267766952966));
#53460=CARTESIAN_POINT('',(-21.6767766952966,-53.8232233047034,-41.9267766952966));
#53461=CARTESIAN_POINT('',(-21.5,-53.6464466094067,-42.3535533905933));
#53462=CARTESIAN_POINT('',(-21.0638697904486,-53.2103163998554,-43.4064648574528));
#53463=CARTESIAN_POINT('',(-22.,-53.6464466094067,-42.3535533905933));
#53464=CARTESIAN_POINT('',(-21.5,-54.,-41.5));
#53465=CARTESIAN_POINT('',(-22.,-54.,-41.5));
#53466=CARTESIAN_POINT('',(-12.0037603021723,-63.4962396978277,-18.5740493299586));
#53467=CARTESIAN_POINT('Origin',(-14.25,-50.8232233047034,-44.8232233047034));
#53468=CARTESIAN_POINT('',(-14.,-50.6464466094067,-44.6464466094067));
#53469=CARTESIAN_POINT('',(-14.5,-51.,-45.));
#53470=CARTESIAN_POINT('Origin',(-14.25,-53.75,21.));
#53471=CARTESIAN_POINT('',(-14.3232233047034,-53.8232233047034,41.9267766952966));
#53472=CARTESIAN_POINT('',(-14.5,-54.,41.5));
#53473=CARTESIAN_POINT('',(-18.0309948196813,-57.5309948196812,32.9754244176564));
#53474=CARTESIAN_POINT('',(-14.5,-54.,21.));
#53475=CARTESIAN_POINT('',(-14.,-53.5,41.7928932188134));
#53476=CARTESIAN_POINT('',(-14.,-53.5,21.));
#53477=CARTESIAN_POINT('',(-11.0530600149149,-50.5530600149149,40.5722307094916));
#53478=CARTESIAN_POINT('Origin',(-21.75,53.75,-21.));
#53479=CARTESIAN_POINT('',(-22.,53.5,-41.7928932188135));
#53480=CARTESIAN_POINT('',(-22.,53.5,-41.7928932188135));
#53481=CARTESIAN_POINT('',(-22.,53.5,41.7928932188134));
#53482=CARTESIAN_POINT('',(-22.,53.5,-21.));
#53483=CARTESIAN_POINT('',(-22.,53.5,41.7928932188134));
#53484=CARTESIAN_POINT('',(-21.5,54.,-21.));
#53485=CARTESIAN_POINT('Origin',(-22.,42.,-54.));
#53486=CARTESIAN_POINT('',(-21.5,45.,-51.));
#53487=CARTESIAN_POINT('Origin',(-21.75,44.8232233047034,-50.8232233047034));
#53488=CARTESIAN_POINT('',(-22.,41.7928932188134,-53.5));
#53489=CARTESIAN_POINT('',(-22.,41.7928932188134,-53.5));
#53490=CARTESIAN_POINT('',(-22.,44.6464466094067,-50.6464466094067));
#53491=CARTESIAN_POINT('Origin',(-22.,-42.,-54.));
#53492=CARTESIAN_POINT('',(-21.5,-21.,-54.));
#53493=CARTESIAN_POINT('Origin',(-21.75,-21.,-53.75));
#53494=CARTESIAN_POINT('',(-22.,-41.7928932188135,-53.5));
#53495=CARTESIAN_POINT('',(-22.,-41.7928932188135,-53.5));
#53496=CARTESIAN_POINT('',(-22.,-21.,-53.5));
#53497=CARTESIAN_POINT('Origin',(-22.,-54.,-42.));
#53498=CARTESIAN_POINT('',(-21.5,-51.,-45.));
#53499=CARTESIAN_POINT('Origin',(-21.75,-50.8232233047034,-44.8232233047034));
#53500=CARTESIAN_POINT('',(-22.,-53.5,-41.7928932188134));
#53501=CARTESIAN_POINT('',(-22.,-53.5,-41.7928932188134));
#53502=CARTESIAN_POINT('',(-22.,-50.6464466094067,-44.6464466094067));
#53503=CARTESIAN_POINT('Origin',(-21.75,-53.75,21.));
#53504=CARTESIAN_POINT('',(-21.5,-54.,41.5));
#53505=CARTESIAN_POINT('',(-21.5,-54.,21.));
#53506=CARTESIAN_POINT('',(-21.5,-54.,41.5));
#53507=CARTESIAN_POINT('',(-22.,-53.5,21.));
#53508=CARTESIAN_POINT('Origin',(-22.,-54.,42.));
#53509=CARTESIAN_POINT('',(-22.,-54.,41.5));
#53510=CARTESIAN_POINT('Origin',(-22.,-53.8232233047034,41.9267766952966));
#53511=CARTESIAN_POINT('',(-14.1464466094067,-54.,41.5));
#53512=CARTESIAN_POINT('',(-21.5,-53.6464466094067,42.3535533905933));
#53513=CARTESIAN_POINT('Origin',(-14.25,34.7896536343781,-34.7896536343781));
#53514=CARTESIAN_POINT('',(-14.,34.7896536343781,-27.5396536343781));
#53515=CARTESIAN_POINT('Origin',(-14.,34.7896536343781,-34.7896536343781));
#53516=CARTESIAN_POINT('',(-14.5,34.7896536343781,-28.0396536343781));
#53517=CARTESIAN_POINT('',(-14.25,34.7896536343781,-27.7896536343781));
#53518=CARTESIAN_POINT('Origin',(-14.5,34.7896536343781,-34.7896536343781));
#53519=CARTESIAN_POINT('Origin',(-14.,0.,0.));
#53520=CARTESIAN_POINT('',(-14.,-44.6464466094067,50.6464466094067));
#53521=CARTESIAN_POINT('',(-14.,34.7896536343781,42.0396536343781));
#53522=CARTESIAN_POINT('Origin',(-14.,34.7896536343781,34.7896536343781));
#53523=CARTESIAN_POINT('',(-14.,-34.7896536343781,-27.5396536343781));
#53524=CARTESIAN_POINT('Origin',(-14.,-34.7896536343781,-34.7896536343781));
#53525=CARTESIAN_POINT('',(-14.,-25.4,-3.11060286983428E-15));
#53526=CARTESIAN_POINT('Origin',(-14.,0.,0.));
#53527=CARTESIAN_POINT('',(-14.,-34.7896536343781,42.0396536343781));
#53528=CARTESIAN_POINT('Origin',(-14.,-34.7896536343781,34.7896536343781));
#53529=CARTESIAN_POINT('Origin',(-22.,34.7896536343781,-34.7896536343781));
#53530=CARTESIAN_POINT('',(-21.5,34.7896536343781,-28.0396536343781));
#53531=CARTESIAN_POINT('Origin',(-21.5,34.7896536343781,-34.7896536343781));
#53532=CARTESIAN_POINT('',(-22.,34.7896536343781,-28.0396536343781));
#53533=CARTESIAN_POINT('Origin',(-14.25,34.7896536343781,34.7896536343781));
#53534=CARTESIAN_POINT('',(-14.5,34.7896536343781,41.5396536343781));
#53535=CARTESIAN_POINT('',(-14.25,34.7896536343781,41.7896536343781));
#53536=CARTESIAN_POINT('Origin',(-14.5,34.7896536343781,34.7896536343781));
#53537=CARTESIAN_POINT('Origin',(-22.,34.7896536343781,34.7896536343781));
#53538=CARTESIAN_POINT('',(-21.5,34.7896536343781,41.5396536343781));
#53539=CARTESIAN_POINT('Origin',(-21.5,34.7896536343781,34.7896536343781));
#53540=CARTESIAN_POINT('',(-22.,34.7896536343781,41.5396536343781));
#53541=CARTESIAN_POINT('Origin',(-14.25,-34.7896536343781,34.7896536343781));
#53542=CARTESIAN_POINT('',(-14.5,-34.7896536343781,41.5396536343781));
#53543=CARTESIAN_POINT('',(-14.25,-34.7896536343781,41.7896536343781));
#53544=CARTESIAN_POINT('Origin',(-14.5,-34.7896536343781,34.7896536343781));
#53545=CARTESIAN_POINT('Origin',(-22.,-34.7896536343781,34.7896536343781));
#53546=CARTESIAN_POINT('',(-21.5,-34.7896536343781,41.5396536343781));
#53547=CARTESIAN_POINT('Origin',(-21.5,-34.7896536343781,34.7896536343781));
#53548=CARTESIAN_POINT('',(-22.,-34.7896536343781,41.5396536343781));
#53549=CARTESIAN_POINT('Origin',(-14.25,-34.7896536343781,-34.7896536343781));
#53550=CARTESIAN_POINT('',(-14.5,-34.7896536343781,-28.0396536343781));
#53551=CARTESIAN_POINT('',(-14.25,-34.7896536343781,-27.7896536343781));
#53552=CARTESIAN_POINT('Origin',(-14.5,-34.7896536343781,-34.7896536343781));
#53553=CARTESIAN_POINT('Origin',(-22.,-34.7896536343781,-34.7896536343781));
#53554=CARTESIAN_POINT('',(-21.5,-34.7896536343781,-28.0396536343781));
#53555=CARTESIAN_POINT('Origin',(-21.5,-34.7896536343781,-34.7896536343781));
#53556=CARTESIAN_POINT('',(-22.,-34.7896536343781,-28.0396536343781));
#53557=CARTESIAN_POINT('Origin',(-21.75,-34.7896536343781,-34.7896536343781));
#53558=CARTESIAN_POINT('',(-22.,-34.7896536343781,-27.5396536343781));
#53559=CARTESIAN_POINT('Origin',(-22.,-34.7896536343781,-34.7896536343781));
#53560=CARTESIAN_POINT('',(-21.75,-34.7896536343781,-27.7896536343781));
#53561=CARTESIAN_POINT('Origin',(-22.,0.,0.));
#53562=CARTESIAN_POINT('',(-22.,50.6464466094067,44.6464466094067));
#53563=CARTESIAN_POINT('',(-22.,-34.7896536343781,42.0396536343781));
#53564=CARTESIAN_POINT('Origin',(-22.,-34.7896536343781,34.7896536343781));
#53565=CARTESIAN_POINT('',(-22.,34.7896536343781,-27.5396536343781));
#53566=CARTESIAN_POINT('Origin',(-22.,34.7896536343781,-34.7896536343781));
#53567=CARTESIAN_POINT('',(-22.,-25.4,3.11060286983428E-15));
#53568=CARTESIAN_POINT('Origin',(-22.,0.,0.));
#53569=CARTESIAN_POINT('',(-22.,34.7896536343781,42.0396536343781));
#53570=CARTESIAN_POINT('Origin',(-22.,34.7896536343781,34.7896536343781));
#53571=CARTESIAN_POINT('Origin',(-21.75,-34.7896536343781,34.7896536343781));
#53572=CARTESIAN_POINT('',(-21.75,-34.7896536343781,41.7896536343781));
#53573=CARTESIAN_POINT('Origin',(-21.75,34.7896536343781,34.7896536343781));
#53574=CARTESIAN_POINT('',(-21.75,34.7896536343781,41.7896536343781));
#53575=CARTESIAN_POINT('Origin',(-21.75,34.7896536343781,-34.7896536343781));
#53576=CARTESIAN_POINT('',(-21.75,34.7896536343781,-27.7896536343781));
#53577=CARTESIAN_POINT('Origin',(-21.75,50.8232233047034,44.8232233047034));
#53578=CARTESIAN_POINT('',(-21.5,51.,45.));
#53579=CARTESIAN_POINT('Origin',(-21.5,-54.,41.5));
#53580=CARTESIAN_POINT('Origin',(-14.25,-44.8232233047034,50.8232233047034));
#53581=CARTESIAN_POINT('Origin',(-22.,54.,-42.));
#53582=CARTESIAN_POINT('Origin',(-22.,54.,42.));
#53583=CARTESIAN_POINT('Origin',(-22.,42.,54.));
#53584=CARTESIAN_POINT('Origin',(-44.1267766952966,0.,-7.66826266755626E-16));
#53585=CARTESIAN_POINT('',(-43.7,25.4,-3.11060286983428E-15));
#53586=CARTESIAN_POINT('',(-43.7,-25.4,-3.11060286983428E-15));
#53587=CARTESIAN_POINT('Origin',(-43.7,0.,0.));
#53588=CARTESIAN_POINT('Origin',(-43.7,0.,0.));
#53589=CARTESIAN_POINT('',(-44.5535533905933,25.0464466094067,3.0673050670225E-15));
#53590=CARTESIAN_POINT('',(-44.1267766952966,25.2232233047034,3.08895396842839E-15));
#53591=CARTESIAN_POINT('',(-44.5535533905933,-25.0464466094067,-3.0673050670225E-15));
#53592=CARTESIAN_POINT('Origin',(-44.5535533905933,0.,-1.53365253351125E-15));
#53593=CARTESIAN_POINT('Origin',(-44.5535533905933,0.,-1.53365253351125E-15));
#53594=CARTESIAN_POINT('Origin',(-44.6,0.,0.));
#53595=CARTESIAN_POINT('',(-44.6464466094067,-24.9535533905933,-3.05592892871426E-15));
#53596=CARTESIAN_POINT('',(-44.6,-25.,-3.06161699786838E-15));
#53597=CARTESIAN_POINT('',(-44.6464466094067,24.9535533905933,-3.05592892871426E-15));
#53598=CARTESIAN_POINT('Origin',(-44.6464466094067,0.,-1.52796446435713E-15));
#53599=CARTESIAN_POINT('Origin',(-44.6464466094067,0.,-1.52796446435713E-15));
#53600=CARTESIAN_POINT('Origin',(-29.1,0.,0.));
#53601=CARTESIAN_POINT('',(-29.1,-25.4,-3.11060286983428E-15));
#53602=CARTESIAN_POINT('Origin',(-44.8232233047034,0.,-7.63982232178566E-16));
#53603=CARTESIAN_POINT('',(-45.,24.1,2.95139878594512E-15));
#53604=CARTESIAN_POINT('',(-44.8232233047034,24.5267766952966,3.00366385732969E-15));
#53605=CARTESIAN_POINT('Origin',(-45.,0.,0.));
#53606=CARTESIAN_POINT('Origin',(-45.,24.6,0.));
#53607=CARTESIAN_POINT('Ctrl Pts',(110.283043754069,-1.58298314962059,11.4890999611639));
#53608=CARTESIAN_POINT('Ctrl Pts',(110.314848605759,-2.84845815047358,11.3147411681003));
#53609=CARTESIAN_POINT('Ctrl Pts',(110.410263160827,-6.56679889300614,10.166830914177));
#53610=CARTESIAN_POINT('Ctrl Pts',(110.537482567584,-10.3238350595526,6.31146214230268));
#53611=CARTESIAN_POINT('Ctrl Pts',(110.696506826031,-12.0956797652182,0.0747112542218324));
#53612=CARTESIAN_POINT('Ctrl Pts',(110.855531084478,-10.6569271560527,-6.51026421705393));
#53613=CARTESIAN_POINT('Ctrl Pts',(111.014555342924,-5.44549032378077,-10.8066656409731));
#53614=CARTESIAN_POINT('Ctrl Pts',(111.109969897992,-1.63327529727618,-11.552899780549));
#53615=CARTESIAN_POINT('Ctrl Pts',(111.141774749681,-0.356448559383722,
-11.5921610579785));
#53616=CARTESIAN_POINT('Ctrl Pts',(110.478573045235,-1.62920838395028,11.8245971128989));
#53617=CARTESIAN_POINT('Ctrl Pts',(110.510377896924,-2.93163695469239,11.6451468088683));
#53618=CARTESIAN_POINT('Ctrl Pts',(110.605792451992,-6.75855824161194,10.4637160335864));
#53619=CARTESIAN_POINT('Ctrl Pts',(110.73301185875,-10.6253049109047,6.49576531480387));
#53620=CARTESIAN_POINT('Ctrl Pts',(110.892036117196,-12.448889862027,0.0768929232018998));
#53621=CARTESIAN_POINT('Ctrl Pts',(111.051060375643,-10.9681237440525,-6.70037267718105));
#53622=CARTESIAN_POINT('Ctrl Pts',(111.21008463409,-5.60450595595427,-11.1222347938706));
#53623=CARTESIAN_POINT('Ctrl Pts',(111.305499189158,-1.68096912987296,-11.8902599727099));
#53624=CARTESIAN_POINT('Ctrl Pts',(111.337304040847,-0.366857336121472,
-11.9306677321785));
#53625=CARTESIAN_POINT('Ctrl Pts',(110.674102336401,-1.67543361827996,12.1600942646339));
#53626=CARTESIAN_POINT('Ctrl Pts',(110.70590718809,-3.0148157589112,11.9755524496363));
#53627=CARTESIAN_POINT('Ctrl Pts',(110.801321743158,-6.95031759021774,10.7606011529959));
#53628=CARTESIAN_POINT('Ctrl Pts',(110.928541149915,-10.9267747622568,6.68006848730506));
#53629=CARTESIAN_POINT('Ctrl Pts',(111.087565408362,-12.8020999588358,0.0790745921819644));
#53630=CARTESIAN_POINT('Ctrl Pts',(111.246589666809,-11.2793203320523,-6.89048113730818));
#53631=CARTESIAN_POINT('Ctrl Pts',(111.405613925255,-5.76352158812776,-11.437803946768));
#53632=CARTESIAN_POINT('Ctrl Pts',(111.501028480323,-1.72866296246974,-12.2276201648708));
#53633=CARTESIAN_POINT('Ctrl Pts',(111.532833332013,-0.377266112859221,
-12.2691744063785));
#53634=CARTESIAN_POINT('Ctrl Pts',(110.869631627566,-1.72165885260965,12.4955914163688));
#53635=CARTESIAN_POINT('Ctrl Pts',(110.901436479255,-3.09799456313001,12.3059580904043));
#53636=CARTESIAN_POINT('Ctrl Pts',(110.996851034323,-7.14207693882354,11.0574862724054));
#53637=CARTESIAN_POINT('Ctrl Pts',(111.124070441081,-11.2282446136089,6.86437165980624));
#53638=CARTESIAN_POINT('Ctrl Pts',(111.283094699527,-13.1553100556447,0.0812562611620312));
#53639=CARTESIAN_POINT('Ctrl Pts',(111.442118957974,-11.5905169200521,-7.0805895974353));
#53640=CARTESIAN_POINT('Ctrl Pts',(111.601143216421,-5.92253722030125,-11.7533730996655));
#53641=CARTESIAN_POINT('Ctrl Pts',(111.696557771489,-1.77635679506652,-12.5649803570316));
#53642=CARTESIAN_POINT('Ctrl Pts',(111.728362623178,-0.387674889596971,
-12.6076810805785));
#53643=CARTESIAN_POINT('',(110.294852708433,-2.05149138653157,11.4148109645546));
#53644=CARTESIAN_POINT('',(110.869631627566,-1.72165885261005,12.4955914163688));
#53645=CARTESIAN_POINT('Ctrl Pts',(110.294852708433,-2.05151014872391,11.4148181175828));
#53646=CARTESIAN_POINT('Ctrl Pts',(110.295777713638,-2.05115143980387,11.4165390179275));
#53647=CARTESIAN_POINT('Ctrl Pts',(110.296702621574,-2.05079204924444,11.4182598296616));
#53648=CARTESIAN_POINT('Ctrl Pts',(110.297627431306,-2.05043197673464,11.4199805509081));
#53649=CARTESIAN_POINT('Ctrl Pts',(110.362289477104,-2.02525596017536,11.5402921698508));
#53650=CARTESIAN_POINT('Ctrl Pts',(110.426669089208,-1.99667407529724,11.6605286357912));
#53651=CARTESIAN_POINT('Ctrl Pts',(110.490401576393,-1.96452355069117,11.7799729158333));
#53652=CARTESIAN_POINT('Ctrl Pts',(110.52225910097,-1.94845268678713,11.8396787151069));
#53653=CARTESIAN_POINT('Ctrl Pts',(110.553954932835,-1.93149088670665,11.8991863079254));
#53654=CARTESIAN_POINT('Ctrl Pts',(110.585443522995,-1.91362250664267,11.9584045796434));
#53655=CARTESIAN_POINT('Ctrl Pts',(110.642821112822,-1.88106326607426,12.0663103857662));
#53656=CARTESIAN_POINT('Ctrl Pts',(110.69991007705,-1.8452663989536,12.1740075423432));
#53657=CARTESIAN_POINT('Ctrl Pts',(110.756284866846,-1.80604384761692,12.2806792435686));
#53658=CARTESIAN_POINT('Ctrl Pts',(110.794438206198,-1.77949880298167,12.3528725347709));
#53659=CARTESIAN_POINT('Ctrl Pts',(110.832264431244,-1.75138558612517,12.4245957776382));
#53660=CARTESIAN_POINT('Ctrl Pts',(110.869631627566,-1.72165885260991,12.4955914163688));
#53661=CARTESIAN_POINT('',(111.113306560609,-1.49574126823376,-11.5007830876033));
#53662=CARTESIAN_POINT('Ctrl Pts',(110.294852708433,-2.05151014872383,11.4148181175829));
#53663=CARTESIAN_POINT('Ctrl Pts',(110.322721242001,-3.15372498702172,11.2170597406403));
#53664=CARTESIAN_POINT('Ctrl Pts',(110.414199478948,-6.68304601222112,10.047541268463));
#53665=CARTESIAN_POINT('Ctrl Pts',(110.537482567584,-10.3238350595526,6.31146214230268));
#53666=CARTESIAN_POINT('Ctrl Pts',(110.696506826031,-12.0956797652182,0.0747112542218324));
#53667=CARTESIAN_POINT('Ctrl Pts',(110.855531084478,-10.6569271560527,-6.51026421705393));
#53668=CARTESIAN_POINT('Ctrl Pts',(111.005065946567,-5.75647048603604,-10.5502880516584));
#53669=CARTESIAN_POINT('Ctrl Pts',(111.090991105277,-2.3847793900036,-11.3863505147081));
#53670=CARTESIAN_POINT('Ctrl Pts',(111.113306560609,-1.49583592206305,-11.5012322968872));
#53671=CARTESIAN_POINT('',(111.666163538309,-0.384363792912494,-12.5));
#53672=CARTESIAN_POINT('Ctrl Pts',(111.666163538309,-0.384363792912482,
-12.5));
#53673=CARTESIAN_POINT('Ctrl Pts',(111.665943629296,-0.385603136713582,
-12.4996308352661));
#53674=CARTESIAN_POINT('Ctrl Pts',(111.665722752094,-0.3868417540112,-12.4992598048037));
#53675=CARTESIAN_POINT('Ctrl Pts',(111.646927229217,-0.491721570729726,
-12.4676667904319));
#53676=CARTESIAN_POINT('Ctrl Pts',(111.621715678588,-0.589568826402512,
-12.4236261787122));
#53677=CARTESIAN_POINT('Ctrl Pts',(111.547301296044,-0.818118357277709,
-12.2914776069231));
#53678=CARTESIAN_POINT('Ctrl Pts',(111.492284046241,-0.941416122263338,
-12.192147571922));
#53679=CARTESIAN_POINT('Ctrl Pts',(111.337452105661,-1.22626137196524,-11.9109461347845));
#53680=CARTESIAN_POINT('Ctrl Pts',(111.226277414691,-1.37389090285344,-11.7075353508788));
#53681=CARTESIAN_POINT('Ctrl Pts',(111.113306560609,-1.49574126823374,-11.5007830876033));
#53682=CARTESIAN_POINT('',(111.698449331144,-1.68935314531931,-12.5));
#53683=CARTESIAN_POINT('Ctrl Pts',(111.698449331144,-1.68946588589014,-12.5005399240113));
#53684=CARTESIAN_POINT('Ctrl Pts',(111.697947425979,-1.68027860774559,-12.5005322965039));
#53685=CARTESIAN_POINT('Ctrl Pts',(111.697451254675,-1.67109103740135,-12.5005247411879));
#53686=CARTESIAN_POINT('Ctrl Pts',(111.696960821607,-1.66190315994946,-12.5005172591199));
#53687=CARTESIAN_POINT('Ctrl Pts',(111.683767253214,-1.41473204240369,-12.5003159774741));
#53688=CARTESIAN_POINT('Ctrl Pts',(111.67474429422,-1.16766800271047,-12.5001701868406));
#53689=CARTESIAN_POINT('Ctrl Pts',(111.669942717737,-0.920412235438467,
-12.5000872409516));
#53690=CARTESIAN_POINT('Ctrl Pts',(111.667814925534,-0.810842202392649,
-12.5000504839372));
#53691=CARTESIAN_POINT('Ctrl Pts',(111.666516115962,-0.701233850372462,
-12.5000258236701));
#53692=CARTESIAN_POINT('Ctrl Pts',(111.666050707469,-0.591558293419319,
-12.5000124326105));
#53693=CARTESIAN_POINT('Ctrl Pts',(111.665757586238,-0.522482986818619,
-12.5000039987208));
#53694=CARTESIAN_POINT('Ctrl Pts',(111.665795205982,-0.45342049399712,-12.4999999999378));
#53695=CARTESIAN_POINT('Ctrl Pts',(111.666163538309,-0.384363792912482,
-12.5));
#53696=CARTESIAN_POINT('Ctrl Pts',(110.869631627566,-1.72165885260965,12.4955914163688));
#53697=CARTESIAN_POINT('Ctrl Pts',(110.901436479255,-3.09799456313,12.3059580904043));
#53698=CARTESIAN_POINT('Ctrl Pts',(110.933241330945,-4.44602202169452,11.889800817738));
#53699=CARTESIAN_POINT('Ctrl Pts',(110.965046182634,-5.68522096696964,11.2629364182439));
#53700=CARTESIAN_POINT('Ctrl Pts',(111.028655886013,-8.16361885751988,10.0092076192556));
#53701=CARTESIAN_POINT('Ctrl Pts',(111.092265589392,-10.2067026949125,7.91265031295602));
#53702=CARTESIAN_POINT('Ctrl Pts',(111.15587529277,-11.4016147585863,5.40496710455104));
#53703=CARTESIAN_POINT('Ctrl Pts',(111.18768014446,-11.9990707904232,4.15112550034857));
#53704=CARTESIAN_POINT('Ctrl Pts',(111.219484996149,-12.3844838788303,2.79450242061976));
#53705=CARTESIAN_POINT('Ctrl Pts',(111.251289847838,-12.5371063953956,1.41263064356073));
#53706=CARTESIAN_POINT('Ctrl Pts',(111.314899551217,-12.8423514285262,-1.35111291055738));
#53707=CARTESIAN_POINT('Ctrl Pts',(111.378509254595,-12.2164341742891,-4.21585125399633));
#53708=CARTESIAN_POINT('Ctrl Pts',(111.442118957974,-10.7698796072204,-6.58277712616185));
#53709=CARTESIAN_POINT('Ctrl Pts',(111.505728661353,-9.32332504015176,-8.94970299832736));
#53710=CARTESIAN_POINT('Ctrl Pts',(111.569338364732,-7.05613316025142,-10.8188163992194));
#53711=CARTESIAN_POINT('Ctrl Pts',(111.63294806811,-4.45765567795809,-11.802568536124));
#53712=CARTESIAN_POINT('Ctrl Pts',(111.654781822455,-3.5657395707398,-12.1402371833971));
#53713=CARTESIAN_POINT('Ctrl Pts',(111.6766155768,-2.63479219550788,-12.3735947089856));
#53714=CARTESIAN_POINT('Ctrl Pts',(111.698449331144,-1.68946588589041,-12.5005399240113));
#53715=CARTESIAN_POINT('Ctrl Pts',(111.15742112713,0.271901404433829,-11.5944522594156));
#53716=CARTESIAN_POINT('Ctrl Pts',(111.204610057985,2.16670657813642,-11.5500171988943));
#53717=CARTESIAN_POINT('Ctrl Pts',(111.298987919696,5.93235416102211,-10.5144384800968));
#53718=CARTESIAN_POINT('Ctrl Pts',(111.440554712261,10.1848431574681,-6.48215877251662));
#53719=CARTESIAN_POINT('Ctrl Pts',(111.582121504826,12.0371931123728,-0.923170511755194));
#53720=CARTESIAN_POINT('Ctrl Pts',(111.723688297391,11.0540455303336,4.85356472268307));
#53721=CARTESIAN_POINT('Ctrl Pts',(111.865255089956,7.46653539266892,9.48674646633624));
#53722=CARTESIAN_POINT('Ctrl Pts',(112.006821882522,2.12006530550471,11.8850101815537));
#53723=CARTESIAN_POINT('Ctrl Pts',(112.148388675087,-3.72590191992946,11.4832747896718));
#53724=CARTESIAN_POINT('Ctrl Pts',(112.289955467652,-8.69407282986275,8.37622032266638));
#53725=CARTESIAN_POINT('Ctrl Pts',(112.431522260217,-11.6140252170778,3.29581715585153));
#53726=CARTESIAN_POINT('Ctrl Pts',(112.573089052782,-11.7978403519213,-2.56104100542157));
#53727=CARTESIAN_POINT('Ctrl Pts',(112.714655845348,-9.20221848328371,-7.81454784931888));
#53728=CARTESIAN_POINT('Ctrl Pts',(112.856222637913,-4.43865660418402,-11.2270344946451));
#53729=CARTESIAN_POINT('Ctrl Pts',(112.997789430478,1.37060254033464,-11.9945582342283));
#53730=CARTESIAN_POINT('Ctrl Pts',(113.139356223043,6.85696329237368,-9.9362987275659));
#53731=CARTESIAN_POINT('Ctrl Pts',(113.280923015609,10.7279004735232,-5.53715895830823));
#53732=CARTESIAN_POINT('Ctrl Pts',(113.422489808174,12.0714648968156,0.166473261964394));
#53733=CARTESIAN_POINT('Ctrl Pts',(113.564056600739,10.5711278304476,5.83088624039759));
#53734=CARTESIAN_POINT('Ctrl Pts',(113.705623393304,6.58035185125043,10.1216079525872));
#53735=CARTESIAN_POINT('Ctrl Pts',(113.847190185869,1.03931892093069,12.0277925731204));
#53736=CARTESIAN_POINT('Ctrl Pts',(113.988756978435,-4.74656586578709,11.1003644305775));
#53737=CARTESIAN_POINT('Ctrl Pts',(114.130323771,-9.41421307630654,7.55781517133264));
#53738=CARTESIAN_POINT('Ctrl Pts',(114.271890563565,-11.8639774806702,2.23472959112623));
#53739=CARTESIAN_POINT('Ctrl Pts',(114.41345735613,-11.5187221158893,-3.61483316724977));
#53740=CARTESIAN_POINT('Ctrl Pts',(114.555024148696,-8.45978526537628,-8.6127818545234));
#53741=CARTESIAN_POINT('Ctrl Pts',(114.696590941261,-3.40781807628825,-11.581655924795));
#53742=CARTESIAN_POINT('Ctrl Pts',(114.838157733826,2.44699275634759,-11.8220220132816));
#53743=CARTESIAN_POINT('Ctrl Pts',(114.979724526391,7.72531959196485,-9.2772525651793));
#53744=CARTESIAN_POINT('Ctrl Pts',(115.121291318956,11.1836479525214,-4.54686667674157));
#53745=CARTESIAN_POINT('Ctrl Pts',(115.262858111522,12.0072345239343,1.25470992130988));
#53746=CARTESIAN_POINT('Ctrl Pts',(115.404424904087,10.0020516002354,6.76069092494371));
#53747=CARTESIAN_POINT('Ctrl Pts',(115.545991696652,5.64049766960815,10.6739292014239));
#53748=CARTESIAN_POINT('Ctrl Pts',(115.687558489217,-0.0498940161182073,
12.0725095394857));
#53749=CARTESIAN_POINT('Ctrl Pts',(115.829125281783,-5.72853146574744,10.6269426623712));
#53750=CARTESIAN_POINT('Ctrl Pts',(115.970692074348,-10.0575907787097,6.67778673879954));
#53751=CARTESIAN_POINT('Ctrl Pts',(116.112258866913,-12.0171957981701,1.15542096924257));
#53752=CARTESIAN_POINT('Ctrl Pts',(116.253825659478,-11.1456822477808,-4.63915256230159));
#53753=CARTESIAN_POINT('Ctrl Pts',(116.395392452043,-7.64837610766902,-9.34078625853751));
#53754=CARTESIAN_POINT('Ctrl Pts',(116.536959244609,-2.34918804318456,-11.8418520279979));
#53755=CARTESIAN_POINT('Ctrl Pts',(116.678526037174,3.50341987815323,-11.5530757135873));
#53756=CARTESIAN_POINT('Ctrl Pts',(116.820092829739,8.53070918247288,-8.54259995247553));
#53757=CARTESIAN_POINT('Ctrl Pts',(116.961659622304,11.5481555073598,-3.51942696985816));
#53758=CARTESIAN_POINT('Ctrl Pts',(117.103226414869,11.8451994508802,2.33252276799301));
#53759=CARTESIAN_POINT('Ctrl Pts',(117.244793207435,9.35114240419514,7.63559939886844));
#53760=CARTESIAN_POINT('Ctrl Pts',(117.339171069145,6.22031361682587,9.97021630652136));
#53761=CARTESIAN_POINT('Ctrl Pts',(117.38636,4.47152467205382,10.7009682121205));
#53762=CARTESIAN_POINT('Ctrl Pts',(111.352950418296,0.279841290678049,-11.9330258397752));
#53763=CARTESIAN_POINT('Ctrl Pts',(111.400139349151,2.22997732067215,-11.8872932157988));
#53764=CARTESIAN_POINT('Ctrl Pts',(111.494517210861,6.10558687122862,-10.8214742073591));
#53765=CARTESIAN_POINT('Ctrl Pts',(111.636084003426,10.4822542585768,-6.67144651591031));
#53766=CARTESIAN_POINT('Ctrl Pts',(111.777650795992,12.3886953203557,-0.950128330758139));
#53767=CARTESIAN_POINT('Ctrl Pts',(111.919217588557,11.3768385082963,4.99529533219344));
#53768=CARTESIAN_POINT('Ctrl Pts',(112.060784381122,7.68456825564656,9.76377220633729));
#53769=CARTESIAN_POINT('Ctrl Pts',(112.202351173687,2.18197406022818,12.2320684435351));
#53770=CARTESIAN_POINT('Ctrl Pts',(112.343917966252,-3.83470326085307,11.8186018385745));
#53771=CARTESIAN_POINT('Ctrl Pts',(112.485484758818,-8.94795143491056,8.62081720754495));
#53772=CARTESIAN_POINT('Ctrl Pts',(112.627051551383,-11.9531703540927,3.39205944394766));
#53773=CARTESIAN_POINT('Ctrl Pts',(112.768618343948,-12.1423531377856,-2.6358268429284));
#53774=CARTESIAN_POINT('Ctrl Pts',(112.910185136513,-9.47093562398407,-8.04274314350251));
#53775=CARTESIAN_POINT('Ctrl Pts',(113.051751929078,-4.56827133930403,-11.5548789827352));
#53776=CARTESIAN_POINT('Ctrl Pts',(113.193318721644,1.41062597559042,-12.3448154464995));
#53777=CARTESIAN_POINT('Ctrl Pts',(113.334885514209,7.05719583120776,-10.2264519974613));
#53778=CARTESIAN_POINT('Ctrl Pts',(113.476452306774,11.0411695777288,-5.69885143774489));
#53779=CARTESIAN_POINT('Ctrl Pts',(113.618019099339,12.4239678869401,0.171334504830907));
#53780=CARTESIAN_POINT('Ctrl Pts',(113.759585891905,10.8798189628888,6.00115595102388));
#53781=CARTESIAN_POINT('Ctrl Pts',(113.90115268447,6.77250696444217,10.417172500772));
#53782=CARTESIAN_POINT('Ctrl Pts',(114.042719477035,1.06966842949927,12.3790202727297));
#53783=CARTESIAN_POINT('Ctrl Pts',(114.1842862696,-4.88517196494861,11.4245099826457));
#53784=CARTESIAN_POINT('Ctrl Pts',(114.325853062165,-9.6891207438874,7.7785135264599));
#53785=CARTESIAN_POINT('Ctrl Pts',(114.467419854731,-12.2104215595334,2.299986697014));
#53786=CARTESIAN_POINT('Ctrl Pts',(114.608986647296,-11.8550842743326,-3.72039115140071));
#53787=CARTESIAN_POINT('Ctrl Pts',(114.750553439861,-8.70682235883157,-8.86428665389625));
#53788=CARTESIAN_POINT('Ctrl Pts',(114.892120232426,-3.50733094170769,-11.9198558349948));
#53789=CARTESIAN_POINT('Ctrl Pts',(115.033687024992,2.51844823178479,-12.1672409361399));
#53790=CARTESIAN_POINT('Ctrl Pts',(115.175253817557,7.95090930117684,-9.54816080186144));
#53791=CARTESIAN_POINT('Ctrl Pts',(115.316820610122,11.510225495302,-4.67964129133471));
#53792=CARTESIAN_POINT('Ctrl Pts',(115.458387402687,12.3578619008925,1.29134913641601));
#53793=CARTESIAN_POINT('Ctrl Pts',(115.599954195252,10.294124942336,6.95811218132984));
#53794=CARTESIAN_POINT('Ctrl Pts',(115.741520987818,5.80520777822571,10.9856222719867));
#53795=CARTESIAN_POINT('Ctrl Pts',(115.883087780383,-0.0513509884095631,
12.4250430345795));
#53796=CARTESIAN_POINT('Ctrl Pts',(116.024654572948,-5.89581227946469,10.9372636628784));
#53797=CARTESIAN_POINT('Ctrl Pts',(116.166221365513,-10.3512859394254,6.87278708158827));
#53798=CARTESIAN_POINT('Ctrl Pts',(116.307788158079,-12.3681140577166,1.1891608135773));
#53799=CARTESIAN_POINT('Ctrl Pts',(116.449354950644,-11.4711511409851,-4.77462204871715));
#53800=CARTESIAN_POINT('Ctrl Pts',(116.590921743209,-7.87171896378435,-9.61354976440806));
#53801=CARTESIAN_POINT('Ctrl Pts',(116.732488535774,-2.4177874896201,-12.1876500139228));
#53802=CARTESIAN_POINT('Ctrl Pts',(116.874055328339,3.60572444460535,-11.8904410432293));
#53803=CARTESIAN_POINT('Ctrl Pts',(117.015622120905,8.77981734957677,-8.79205534603593));
#53804=CARTESIAN_POINT('Ctrl Pts',(117.15718891347,11.8853771603708,-3.6221989648898));
#53805=CARTESIAN_POINT('Ctrl Pts',(117.298755706035,12.1910951860497,2.40063556600711));
#53806=CARTESIAN_POINT('Ctrl Pts',(117.4403224986,9.62420832342993,7.8585691579243));
#53807=CARTESIAN_POINT('Ctrl Pts',(117.53470036031,6.4019551299468,10.2613600152824));
#53808=CARTESIAN_POINT('Ctrl Pts',(117.581889291165,4.60209919890604,11.0134508581162));
#53809=CARTESIAN_POINT('Ctrl Pts',(111.548479709461,0.287781176922269,-12.2715994201348));
#53810=CARTESIAN_POINT('Ctrl Pts',(111.595668640316,2.29324806320787,-12.2245692327033));
#53811=CARTESIAN_POINT('Ctrl Pts',(111.690046502027,6.27881958143513,-11.1285099346214));
#53812=CARTESIAN_POINT('Ctrl Pts',(111.831613294592,10.7796653596855,-6.86073425930401));
#53813=CARTESIAN_POINT('Ctrl Pts',(111.973180087157,12.7401975283385,-0.977086149761075));
#53814=CARTESIAN_POINT('Ctrl Pts',(112.114746879722,11.6996314862591,5.13702594170381));
#53815=CARTESIAN_POINT('Ctrl Pts',(112.256313672287,7.9026011186242,10.0407979463383));
#53816=CARTESIAN_POINT('Ctrl Pts',(112.397880464853,2.24388281495165,12.5791267055165));
#53817=CARTESIAN_POINT('Ctrl Pts',(112.539447257418,-3.94350460177667,12.1539288874771));
#53818=CARTESIAN_POINT('Ctrl Pts',(112.681014049983,-9.20183003995837,8.86541409242353));
#53819=CARTESIAN_POINT('Ctrl Pts',(112.822580842548,-12.2923154911077,3.4883017320438));
#53820=CARTESIAN_POINT('Ctrl Pts',(112.964147635114,-12.4868659236498,-2.71061268043522));
#53821=CARTESIAN_POINT('Ctrl Pts',(113.105714427679,-9.73965276468443,-8.27093843768614));
#53822=CARTESIAN_POINT('Ctrl Pts',(113.247281220244,-4.69788607442404,-11.8827234708253));
#53823=CARTESIAN_POINT('Ctrl Pts',(113.388848012809,1.4506494108462,-12.6950726587707));
#53824=CARTESIAN_POINT('Ctrl Pts',(113.530414805374,7.25742837004184,-10.5166052673566));
#53825=CARTESIAN_POINT('Ctrl Pts',(113.67198159794,11.3544386819345,-5.86054391718156));
#53826=CARTESIAN_POINT('Ctrl Pts',(113.813548390505,12.7764708770647,0.176195747697426));
#53827=CARTESIAN_POINT('Ctrl Pts',(113.95511518307,11.1885100953299,6.17142566165016));
#53828=CARTESIAN_POINT('Ctrl Pts',(114.096681975635,6.96466207763389,10.7127370489567));
#53829=CARTESIAN_POINT('Ctrl Pts',(114.238248768201,1.10001793806786,12.730247972339));
#53830=CARTESIAN_POINT('Ctrl Pts',(114.379815560766,-5.02377806411015,11.748655534714));
#53831=CARTESIAN_POINT('Ctrl Pts',(114.521382353331,-9.96402841146824,7.99921188158716));
#53832=CARTESIAN_POINT('Ctrl Pts',(114.662949145896,-12.5568656383966,2.36524380290177));
#53833=CARTESIAN_POINT('Ctrl Pts',(114.804515938461,-12.1914464327759,-3.82594913555166));
#53834=CARTESIAN_POINT('Ctrl Pts',(114.946082731027,-8.95385945228687,-9.11579145326909));
#53835=CARTESIAN_POINT('Ctrl Pts',(115.087649523592,-3.60684380712713,-12.2580557451947));
#53836=CARTESIAN_POINT('Ctrl Pts',(115.229216316157,2.589903707222,-12.5124598589981));
#53837=CARTESIAN_POINT('Ctrl Pts',(115.370783108722,8.17649901038882,-9.81906903854357));
#53838=CARTESIAN_POINT('Ctrl Pts',(115.512349901287,11.8368030380826,-4.81241590592785));
#53839=CARTESIAN_POINT('Ctrl Pts',(115.653916693853,12.7084892778507,1.32798835152213));
#53840=CARTESIAN_POINT('Ctrl Pts',(115.795483486418,10.5861982844366,7.15553343771598));
#53841=CARTESIAN_POINT('Ctrl Pts',(115.937050278983,5.96991788684329,11.2973153425495));
#53842=CARTESIAN_POINT('Ctrl Pts',(116.078617071548,-0.0528079607009308,
12.7775765296732));
#53843=CARTESIAN_POINT('Ctrl Pts',(116.220183864114,-6.06309309318193,11.2475846633857));
#53844=CARTESIAN_POINT('Ctrl Pts',(116.361750656679,-10.6449811001411,7.06778742437699));
#53845=CARTESIAN_POINT('Ctrl Pts',(116.503317449244,-12.7190323172631,1.22290065791204));
#53846=CARTESIAN_POINT('Ctrl Pts',(116.644884241809,-11.7966200341894,-4.91009153513272));
#53847=CARTESIAN_POINT('Ctrl Pts',(116.786451034374,-8.09506181989969,-9.88631327027862));
#53848=CARTESIAN_POINT('Ctrl Pts',(116.92801782694,-2.48638693605563,-12.5334479998476));
#53849=CARTESIAN_POINT('Ctrl Pts',(117.069584619505,3.70802901105746,-12.2278063728712));
#53850=CARTESIAN_POINT('Ctrl Pts',(117.21115141207,9.02892551668066,-9.04151073959632));
#53851=CARTESIAN_POINT('Ctrl Pts',(117.352718204635,12.2225988133817,-3.72497095992145));
#53852=CARTESIAN_POINT('Ctrl Pts',(117.494284997201,12.5369909212193,2.46874836402119));
#53853=CARTESIAN_POINT('Ctrl Pts',(117.635851789766,9.89727424266471,8.08153891698017));
#53854=CARTESIAN_POINT('Ctrl Pts',(117.730229651476,6.58359664306774,10.5525037240434));
#53855=CARTESIAN_POINT('Ctrl Pts',(117.777418582331,4.73267372575826,11.3259335041118));
#53856=CARTESIAN_POINT('Ctrl Pts',(111.744009000627,0.295721063166489,-12.6101730004945));
#53857=CARTESIAN_POINT('Ctrl Pts',(111.791197931482,2.3565188057436,-12.5618452496078));
#53858=CARTESIAN_POINT('Ctrl Pts',(111.885575793192,6.45205229164162,-11.4355456618837));
#53859=CARTESIAN_POINT('Ctrl Pts',(112.027142585757,11.0770764607942,-7.05002200269771));
#53860=CARTESIAN_POINT('Ctrl Pts',(112.168709378323,13.0916997363214,-1.00404396876402));
#53861=CARTESIAN_POINT('Ctrl Pts',(112.310276170888,12.0224244642218,5.27875655121417));
#53862=CARTESIAN_POINT('Ctrl Pts',(112.451842963453,8.12063398160184,10.3178236863394));
#53863=CARTESIAN_POINT('Ctrl Pts',(112.593409756018,2.30579156967512,12.9261849674979));
#53864=CARTESIAN_POINT('Ctrl Pts',(112.734976548583,-4.05230594270028,12.4892559363798));
#53865=CARTESIAN_POINT('Ctrl Pts',(112.876543341149,-9.45570864500619,9.1100109773021));
#53866=CARTESIAN_POINT('Ctrl Pts',(113.018110133714,-12.6314606281227,3.58454402013992));
#53867=CARTESIAN_POINT('Ctrl Pts',(113.159676926279,-12.8313787095141,-2.78539851794204));
#53868=CARTESIAN_POINT('Ctrl Pts',(113.301243718844,-10.0083699053848,-8.49913373186977));
#53869=CARTESIAN_POINT('Ctrl Pts',(113.44281051141,-4.82750080954404,-12.2105679589154));
#53870=CARTESIAN_POINT('Ctrl Pts',(113.584377303975,1.49067284610198,-13.045329871042));
#53871=CARTESIAN_POINT('Ctrl Pts',(113.72594409654,7.45766090887593,-10.8067585372519));
#53872=CARTESIAN_POINT('Ctrl Pts',(113.867510889105,11.6677077861402,-6.02223639661823));
#53873=CARTESIAN_POINT('Ctrl Pts',(114.00907768167,13.1289738671892,0.18105699056394));
#53874=CARTESIAN_POINT('Ctrl Pts',(114.150644474236,11.4972012277711,6.34169537227645));
#53875=CARTESIAN_POINT('Ctrl Pts',(114.292211266801,7.15681719082563,11.0083015971415));
#53876=CARTESIAN_POINT('Ctrl Pts',(114.433778059366,1.13036744663645,13.0814756719483));
#53877=CARTESIAN_POINT('Ctrl Pts',(114.575344851931,-5.16238416327168,12.0728010867823));
#53878=CARTESIAN_POINT('Ctrl Pts',(114.716911644497,-10.2389360790491,8.21991023671442));
#53879=CARTESIAN_POINT('Ctrl Pts',(114.858478437062,-12.9033097172598,2.43050090878955));
#53880=CARTESIAN_POINT('Ctrl Pts',(115.000045229627,-12.5278085912191,-3.93150711970261));
#53881=CARTESIAN_POINT('Ctrl Pts',(115.141612022192,-9.20089654574217,-9.36729625264193));
#53882=CARTESIAN_POINT('Ctrl Pts',(115.283178814757,-3.70635667254657,-12.5962556553946));
#53883=CARTESIAN_POINT('Ctrl Pts',(115.424745607323,2.6613591826592,-12.8576787818564));
#53884=CARTESIAN_POINT('Ctrl Pts',(115.566312399888,8.4020887196008,-10.0899772752257));
#53885=CARTESIAN_POINT('Ctrl Pts',(115.707879192453,12.1633805808632,-4.94519052052099));
#53886=CARTESIAN_POINT('Ctrl Pts',(115.849445985018,13.0591166548089,1.36462756662826));
#53887=CARTESIAN_POINT('Ctrl Pts',(115.991012777583,10.8782716265372,7.35295469410212));
#53888=CARTESIAN_POINT('Ctrl Pts',(116.132579570149,6.13462799546086,11.6090084131123));
#53889=CARTESIAN_POINT('Ctrl Pts',(116.274146362714,-0.0542649329922895,
13.130110024767));
#53890=CARTESIAN_POINT('Ctrl Pts',(116.415713155279,-6.23037390689917,11.557905663893));
#53891=CARTESIAN_POINT('Ctrl Pts',(116.557279947844,-10.9386762608569,7.26278776716572));
#53892=CARTESIAN_POINT('Ctrl Pts',(116.69884674041,-13.0699505768096,1.25664050224678));
#53893=CARTESIAN_POINT('Ctrl Pts',(116.840413532975,-12.1220889273937,-5.04556102154829));
#53894=CARTESIAN_POINT('Ctrl Pts',(116.98198032554,-8.31840467601501,-10.1590767761492));
#53895=CARTESIAN_POINT('Ctrl Pts',(117.123547118105,-2.55498638249118,-12.8792459857725));
#53896=CARTESIAN_POINT('Ctrl Pts',(117.26511391067,3.81033357750957,-12.5651717025131));
#53897=CARTESIAN_POINT('Ctrl Pts',(117.406680703236,9.27803368378454,-9.29096613315673));
#53898=CARTESIAN_POINT('Ctrl Pts',(117.548247495801,12.5598204663927,-3.82774295495309));
#53899=CARTESIAN_POINT('Ctrl Pts',(117.689814288366,12.8828866563888,2.53686116203528));
#53900=CARTESIAN_POINT('Ctrl Pts',(117.831381080931,10.1703401618995,8.30450867603603));
#53901=CARTESIAN_POINT('Ctrl Pts',(117.925758942641,6.76523815618867,10.8436474328044));
#53902=CARTESIAN_POINT('Ctrl Pts',(117.972947873497,4.86324825261048,11.6384161501074));
#53903=CARTESIAN_POINT('',(117.141306474002,-1.68935314531914,-12.5));
#53904=CARTESIAN_POINT('',(117.218885227957,1.68935314531925,-12.5));
#53905=CARTESIAN_POINT('Ctrl Pts',(117.141306474002,-1.68966005362616,-12.500608264671));
#53906=CARTESIAN_POINT('Ctrl Pts',(117.140804568838,-1.68047463572448,-12.5006004763374));
#53907=CARTESIAN_POINT('Ctrl Pts',(117.140308397533,-1.67128889071667,-12.5005926219721));
#53908=CARTESIAN_POINT('Ctrl Pts',(117.139817964464,-1.66210280379621,-12.5005847053769));
#53909=CARTESIAN_POINT('Ctrl Pts',(117.126559275382,-1.41376010819252,-12.5003706829534));
#53910=CARTESIAN_POINT('Ctrl Pts',(117.117512467812,-1.16550008733763,-12.5001134860496));
#53911=CARTESIAN_POINT('Ctrl Pts',(117.112729070399,-0.917020752225694,
-12.4998770325662));
#53912=CARTESIAN_POINT('Ctrl Pts',(117.110643239224,-0.808669741663733,
-12.4997739255056));
#53913=CARTESIAN_POINT('Ctrl Pts',(117.10936807505,-0.700276366307754,-12.4996745527923));
#53914=CARTESIAN_POINT('Ctrl Pts',(117.108907850327,-0.591812800653879,
-12.4995829446679));
#53915=CARTESIAN_POINT('Ctrl Pts',(117.10815486932,-0.414353831801932,-12.4994330631552));
#53916=CARTESIAN_POINT('Ctrl Pts',(117.109584424463,-0.236967696978893,
-12.4993044175444));
#53917=CARTESIAN_POINT('Ctrl Pts',(117.113196032071,-0.0595349787923405,
-12.4992090581988));
#53918=CARTESIAN_POINT('Ctrl Pts',(117.113465330855,-0.0463047443763591,
-12.4992019477487));
#53919=CARTESIAN_POINT('Ctrl Pts',(117.113746751044,-0.0330747720332224,
-12.4991950195628));
#53920=CARTESIAN_POINT('Ctrl Pts',(117.114040289568,-0.0198450123812237,
-12.4991882770983));
#53921=CARTESIAN_POINT('Ctrl Pts',(117.114120941615,-0.0162100305813574,
-12.4991864245525));
#53922=CARTESIAN_POINT('Ctrl Pts',(117.114202508421,-0.0125750683061462,
-12.4991845860277));
#53923=CARTESIAN_POINT('Ctrl Pts',(117.114284989917,-0.00894012455784924,
-12.4991827615927));
#53924=CARTESIAN_POINT('Ctrl Pts',(117.114333443178,-0.00680479866143413,
-12.4991816898394));
#53925=CARTESIAN_POINT('Ctrl Pts',(117.11438221208,-0.00466947955864029,
-12.4991806229485));
#53926=CARTESIAN_POINT('Ctrl Pts',(117.114431296611,-0.00253416694871591,
-12.4991795609337));
#53927=CARTESIAN_POINT('Ctrl Pts',(117.114473674849,-0.000690596637058661,
-12.4991786440194));
#53928=CARTESIAN_POINT('Ctrl Pts',(117.114516288354,0.00115296855477631,
-12.4991777307399));
#53929=CARTESIAN_POINT('Ctrl Pts',(117.114559137117,0.00299652874669277,
-12.499176821104));
#53930=CARTESIAN_POINT('Ctrl Pts',(117.114611320797,0.00524172200240544,
-12.4991757132974));
#53931=CARTESIAN_POINT('Ctrl Pts',(117.114663853399,0.00748690754199927,
-12.4991746108951));
#53932=CARTESIAN_POINT('Ctrl Pts',(117.114716734904,0.00973208555912489,
-12.4991735139129));
#53933=CARTESIAN_POINT('Ctrl Pts',(117.11481650341,0.0139679342504296,-12.4991714442994));
#53934=CARTESIAN_POINT('Ctrl Pts',(117.114917513772,0.0182037545289113,
-12.499169393979));
#53935=CARTESIAN_POINT('Ctrl Pts',(117.115019765873,0.0224395480908287,
-12.4991673630552));
#53936=CARTESIAN_POINT('Ctrl Pts',(117.115602197855,0.0465667943806478,
-12.4991557948337));
#53937=CARTESIAN_POINT('Ctrl Pts',(117.116224911658,0.070692915173029,-12.4991448562447));
#53938=CARTESIAN_POINT('Ctrl Pts',(117.116887882688,0.0948182088186656,
-12.4991345650034));
#53939=CARTESIAN_POINT('Ctrl Pts',(117.117735535906,0.125664025393719,-12.4991214069566));
#53940=CARTESIAN_POINT('Ctrl Pts',(117.118648976774,0.15650768043098,-12.4991093076991));
#53941=CARTESIAN_POINT('Ctrl Pts',(117.119628143454,0.187349795104028,-12.4990982985367));
#53942=CARTESIAN_POINT('Ctrl Pts',(117.124449939474,0.339228314825474,-12.4990440851568));
#53943=CARTESIAN_POINT('Ctrl Pts',(117.130863523257,0.491005283256536,-12.4990166205082));
#53944=CARTESIAN_POINT('Ctrl Pts',(117.13885739767,0.642753325474625,-12.4990173756166));
#53945=CARTESIAN_POINT('Ctrl Pts',(117.151510948311,0.882956190529511,-12.4990185708822));
#53946=CARTESIAN_POINT('Ctrl Pts',(117.168102434924,1.12266909663543,-12.4990921998159));
#53947=CARTESIAN_POINT('Ctrl Pts',(117.188543046603,1.36216112185186,-12.4992236134943));
#53948=CARTESIAN_POINT('Ctrl Pts',(117.197860187627,1.47132522163686,-12.4992835138434));
#53949=CARTESIAN_POINT('Ctrl Pts',(117.207977051648,1.58044277825126,-12.4993551794546));
#53950=CARTESIAN_POINT('Ctrl Pts',(117.218885227957,1.68953572661318,-12.499436378717));
#53951=CARTESIAN_POINT('',(115.404599513671,1.68935314531934,-12.5));
#53952=CARTESIAN_POINT('Ctrl Pts',(115.404599513671,1.6896686969101,-12.5005137686862));
#53953=CARTESIAN_POINT('Ctrl Pts',(115.411314878222,1.98036881708519,-12.4614884428392));
#53954=CARTESIAN_POINT('Ctrl Pts',(115.418030242772,2.26967326198219,-12.4122686062437));
#53955=CARTESIAN_POINT('Ctrl Pts',(115.424745607323,2.55686146294845,-12.352824676341));
#53956=CARTESIAN_POINT('Ctrl Pts',(115.471934538178,4.57493569497303,-11.9351116129795));
#53957=CARTESIAN_POINT('Ctrl Pts',(115.519123469033,6.48851220728691,-11.0125444441026));
#53958=CARTESIAN_POINT('Ctrl Pts',(115.566312399888,8.07218244032092,-9.69379640054671));
#53959=CARTESIAN_POINT('Ctrl Pts',(115.613501330743,9.65585267335493,-8.3750483569908));
#53960=CARTESIAN_POINT('Ctrl Pts',(115.660690261598,10.9096166271091,-6.66011943875589));
#53961=CARTESIAN_POINT('Ctrl Pts',(115.707879192453,11.6857879496437,-4.75101863178023));
#53962=CARTESIAN_POINT('Ctrl Pts',(115.755068123308,12.4619592721784,-2.84191782480457));
#53963=CARTESIAN_POINT('Ctrl Pts',(115.802257054163,12.7605379634937,-0.738645129088155));
#53964=CARTESIAN_POINT('Ctrl Pts',(115.849445985018,12.5463531377727,1.31104574001571));
#53965=CARTESIAN_POINT('Ctrl Pts',(115.896634915873,12.3321683120517,3.36073660911957));
#53966=CARTESIAN_POINT('Ctrl Pts',(115.943823846728,11.6052199692944,5.35684565161087));
#53967=CARTESIAN_POINT('Ctrl Pts',(115.991012777583,10.4511385260698,7.06424245935823));
#53968=CARTESIAN_POINT('Ctrl Pts',(116.038201708439,9.2970570828451,8.77163926710553));
#53969=CARTESIAN_POINT('Ctrl Pts',(116.085390639294,7.715842539153,10.1903238401089));
#53970=CARTESIAN_POINT('Ctrl Pts',(116.132579570149,5.89375311256478,11.1531830618864));
#53971=CARTESIAN_POINT('Ctrl Pts',(116.179768501004,4.07166368597657,12.1160422836638));
#53972=CARTESIAN_POINT('Ctrl Pts',(116.226957431859,2.00869937649223,12.6230761542154));
#53973=CARTESIAN_POINT('Ctrl Pts',(116.274146362714,-0.0521342739010579,
12.6145590293455));
#53974=CARTESIAN_POINT('Ctrl Pts',(116.321335293569,-2.11296792429447,12.6060419044757));
#53975=CARTESIAN_POINT('Ctrl Pts',(116.368524224424,-4.17167091559683,12.0819737841843));
#53976=CARTESIAN_POINT('Ctrl Pts',(116.415713155279,-5.98573947024097,11.1040867412508));
#53977=CARTESIAN_POINT('Ctrl Pts',(116.462902086134,-7.79980802488507,10.1261996983172));
#53978=CARTESIAN_POINT('Ctrl Pts',(116.510091016989,-9.36924214287096,8.69449373274147));
#53979=CARTESIAN_POINT('Ctrl Pts',(116.557279947844,-10.509171587856,6.97761620580043));
#53980=CARTESIAN_POINT('Ctrl Pts',(116.604468878699,-11.6491010328411,5.26073867885939));
#53981=CARTESIAN_POINT('Ctrl Pts',(116.651657809554,-12.3595258048254,3.25868959055305));
#53982=CARTESIAN_POINT('Ctrl Pts',(116.69884674041,-12.5567612492482,1.20729812576737));
#53983=CARTESIAN_POINT('Ctrl Pts',(116.746035671265,-12.753996693671,-0.844093339018264));
#53984=CARTESIAN_POINT('Ctrl Pts',(116.79322460212,-12.4380428105324,-2.94482718028324));
#53985=CARTESIAN_POINT('Ctrl Pts',(116.840413532975,-11.6461184937333,-4.84744672668254));
#53986=CARTESIAN_POINT('Ctrl Pts',(116.88760246383,-10.8541941769342,-6.75006627308188));
#53987=CARTESIAN_POINT('Ctrl Pts',(116.934791394685,-9.58629942647459,-8.45457152461553));
#53988=CARTESIAN_POINT('Ctrl Pts',(116.98198032554,-7.9917823356575,-9.76018568531958));
#53989=CARTESIAN_POINT('Ctrl Pts',(117.029169256395,-6.3972652448404,-11.0657998460236));
#53990=CARTESIAN_POINT('Ctrl Pts',(117.07635818725,-4.47612581366579,-11.9725229158981));
#53991=CARTESIAN_POINT('Ctrl Pts',(117.123547118105,-2.45466943807836,-12.3735387369587));
#53992=CARTESIAN_POINT('Ctrl Pts',(117.129466903404,-2.20108056633454,-12.4238456101826));
#53993=CARTESIAN_POINT('Ctrl Pts',(117.135386688703,-1.94591297160764,-12.4661939908398));
#53994=CARTESIAN_POINT('Ctrl Pts',(117.141306474002,-1.68966005362669,-12.5006082646709));
#53995=CARTESIAN_POINT('',(115.327020759716,-1.68935314531923,-12.5));
#53996=CARTESIAN_POINT('Ctrl Pts',(115.327020759716,-1.68956493984068,-12.4995253250381));
#53997=CARTESIAN_POINT('Ctrl Pts',(115.326518854553,-1.68037728524638,-12.4995179807198));
#53998=CARTESIAN_POINT('Ctrl Pts',(115.326022683248,-1.67118932027433,-12.4995106941419));
#53999=CARTESIAN_POINT('Ctrl Pts',(115.325532250178,-1.66200103015941,-12.4995034672907));
#54000=CARTESIAN_POINT('Ctrl Pts',(115.312311851236,-1.41431613999935,-12.4993086560875));
#54001=CARTESIAN_POINT('Ctrl Pts',(115.303279041712,-1.16672568500685,-12.4991596530256));
#54002=CARTESIAN_POINT('Ctrl Pts',(115.298484905107,-0.918930641817005,
-12.4990826397731));
#54003=CARTESIAN_POINT('Ctrl Pts',(115.296374451076,-0.809847382263608,
-12.499048737333));
#54004=CARTESIAN_POINT('Ctrl Pts',(115.295085408755,-0.70072381008354,-12.4990285536869));
#54005=CARTESIAN_POINT('Ctrl Pts',(115.294622136041,-0.591531575591215,
-12.4990229307716));
#54006=CARTESIAN_POINT('Ctrl Pts',(115.293869155035,-0.414055812104477,
-12.4990137915577));
#54007=CARTESIAN_POINT('Ctrl Pts',(115.295298710178,-0.236659403045372,
-12.4990433559505));
#54008=CARTESIAN_POINT('Ctrl Pts',(115.298910317785,-0.0592230017119202,
-12.4991092977448));
#54009=CARTESIAN_POINT('Ctrl Pts',(115.299179616569,-0.0459924926625598,
-12.4991142146813));
#54010=CARTESIAN_POINT('Ctrl Pts',(115.299461036758,-0.0327622823487279,
-12.4991193305549));
#54011=CARTESIAN_POINT('Ctrl Pts',(115.299754575282,-0.0195323214148313,
-12.4991246428424));
#54012=CARTESIAN_POINT('Ctrl Pts',(115.299835227329,-0.0158972842946123,
-12.4991261024357));
#54013=CARTESIAN_POINT('Ctrl Pts',(115.299916794136,-0.0122622694687753,
-12.4991275768541));
#54014=CARTESIAN_POINT('Ctrl Pts',(115.299999275632,-0.00862727598571485,
-12.4991290660423));
#54015=CARTESIAN_POINT('Ctrl Pts',(115.300047728892,-0.00649192084135235,
-12.499129940857));
#54016=CARTESIAN_POINT('Ctrl Pts',(115.300096497795,-0.0043565734465251,
-12.4991308207685));
#54017=CARTESIAN_POINT('Ctrl Pts',(115.300145582325,-0.00222123354126288,
-12.4991317057653));
#54018=CARTESIAN_POINT('Ctrl Pts',(115.300187960563,-0.000377639640268286,
-12.4991324698473));
#54019=CARTESIAN_POINT('Ctrl Pts',(115.300230574068,0.00146594842845679,
-12.4991332377199));
#54020=CARTESIAN_POINT('Ctrl Pts',(115.300273422832,0.00330953078475597,
-12.4991340093757));
#54021=CARTESIAN_POINT('Ctrl Pts',(115.300325606511,0.0055547510331301,
-12.4991349491423));
#54022=CARTESIAN_POINT('Ctrl Pts',(115.300378139113,0.00779996250852122,
-12.49913589452));
#54023=CARTESIAN_POINT('Ctrl Pts',(115.300431020618,0.0100451654044689,
-12.4991368454951));
#54024=CARTESIAN_POINT('Ctrl Pts',(115.300530789124,0.0142810610559831,
-12.4991386396453));
#54025=CARTESIAN_POINT('Ctrl Pts',(115.300631799487,0.0185169245314509,
-12.4991404537185));
#54026=CARTESIAN_POINT('Ctrl Pts',(115.300734051588,0.0227527574583523,
-12.4991422876221));
#54027=CARTESIAN_POINT('Ctrl Pts',(115.301316483569,0.0468802282284872,
-12.4991527336089));
#54028=CARTESIAN_POINT('Ctrl Pts',(115.301939197372,0.0710064513896376,
-12.4991638230625));
#54029=CARTESIAN_POINT('Ctrl Pts',(115.302602168403,0.0951317251787609,
-12.4991755374429));
#54030=CARTESIAN_POINT('Ctrl Pts',(115.303449821618,0.125977516261023,-12.499190515069));
#54031=CARTESIAN_POINT('Ctrl Pts',(115.304363262483,0.156820945974577,-12.4992065140888));
#54032=CARTESIAN_POINT('Ctrl Pts',(115.305342429159,0.18766263524768,-12.4992234901137));
#54033=CARTESIAN_POINT('Ctrl Pts',(115.310164225167,0.339539060211866,-12.4993070866366));
#54034=CARTESIAN_POINT('Ctrl Pts',(115.31657780893,0.491309083351229,-12.4994146211685));
#54035=CARTESIAN_POINT('Ctrl Pts',(115.324571683316,0.643045308941025,-12.4995385978385));
#54036=CARTESIAN_POINT('Ctrl Pts',(115.337251836494,0.883734427911741,-12.4997352538142));
#54037=CARTESIAN_POINT('Ctrl Pts',(115.353886501112,1.12391931965973,-12.4999745588541));
#54038=CARTESIAN_POINT('Ctrl Pts',(115.374386304944,1.36387073326171,-12.500207396726));
#54039=CARTESIAN_POINT('Ctrl Pts',(115.383667815097,1.47251135732339,-12.5003128166164));
#54040=CARTESIAN_POINT('Ctrl Pts',(115.393741649628,1.58110346898439,-12.5004166949864));
#54041=CARTESIAN_POINT('Ctrl Pts',(115.404599513671,1.68966869690974,-12.5005137686862));
#54042=CARTESIAN_POINT('',(113.590313799386,1.68935314531925,-12.5));
#54043=CARTESIAN_POINT('Ctrl Pts',(113.590313799386,1.68940030131958,-12.5009781087056));
#54044=CARTESIAN_POINT('Ctrl Pts',(113.635523898437,3.64596800314944,-12.2358114053962));
#54045=CARTESIAN_POINT('Ctrl Pts',(113.680733997489,5.53979258690265,-11.5038643043075));
#54046=CARTESIAN_POINT('Ctrl Pts',(113.72594409654,7.16483737795765,-10.382433402778));
#54047=CARTESIAN_POINT('Ctrl Pts',(113.773133027395,8.86100986796402,-9.21191782370736));
#54048=CARTESIAN_POINT('Ctrl Pts',(113.82032195825,10.2643588270521,-7.61707711016277));
#54049=CARTESIAN_POINT('Ctrl Pts',(113.867510889105,11.2095776534377,-5.78577452219343));
#54050=CARTESIAN_POINT('Ctrl Pts',(113.91469981996,12.1547964798232,-3.95447193422415));
#54051=CARTESIAN_POINT('Ctrl Pts',(113.961888750815,12.6418851735062,-1.88670747183014));
#54052=CARTESIAN_POINT('Ctrl Pts',(114.00907768167,12.613467413778,0.173947822985603));
#54053=CARTESIAN_POINT('Ctrl Pts',(114.056266612526,12.5850496540499,2.23460311780141));
#54054=CARTESIAN_POINT('Ctrl Pts',(114.103455543381,12.0411254409105,4.28814924503892));
#54055=CARTESIAN_POINT('Ctrl Pts',(114.150644474236,11.0457659948499,6.09269001280186));
#54056=CARTESIAN_POINT('Ctrl Pts',(114.197833405091,10.0504065487893,7.8972307805648));
#54057=CARTESIAN_POINT('Ctrl Pts',(114.245022335946,8.60361186980746,9.45276618885315));
#54058=CARTESIAN_POINT('Ctrl Pts',(114.292211266801,6.87580623961835,10.5760629054651));
#54059=CARTESIAN_POINT('Ctrl Pts',(114.339400197656,5.14800060942926,11.6993596220771));
#54060=CARTESIAN_POINT('Ctrl Pts',(114.386589128511,3.13918402803281,12.3904176470127));
#54061=CARTESIAN_POINT('Ctrl Pts',(114.433778059366,1.08598380234995,12.5678342286195));
#54062=CARTESIAN_POINT('Ctrl Pts',(114.480966990221,-0.967216423332948,
12.7452508102263));
#54063=CARTESIAN_POINT('Ctrl Pts',(114.528155921076,-3.06480029330234,12.4090259485043));
#54064=CARTESIAN_POINT('Ctrl Pts',(114.575344851931,-4.95968421424995,11.5987650426319));
#54065=CARTESIAN_POINT('Ctrl Pts',(114.622533782786,-6.8545681351975,10.7885041367596));
#54066=CARTESIAN_POINT('Ctrl Pts',(114.669722713641,-8.54675210712326,9.50420718673705));
#54067=CARTESIAN_POINT('Ctrl Pts',(114.716911644497,-9.83690636612127,7.89715715707163));
#54068=CARTESIAN_POINT('Ctrl Pts',(114.764100575352,-11.1270606251194,6.29010712740612));
#54069=CARTESIAN_POINT('Ctrl Pts',(114.811289506207,-12.0151851711896,4.36030401809775));
#54070=CARTESIAN_POINT('Ctrl Pts',(114.858478437062,-12.3966639232179,2.33506779202817));
#54071=CARTESIAN_POINT('Ctrl Pts',(114.905667367917,-12.7781426752463,0.309831565958702));
#54072=CARTESIAN_POINT('Ctrl Pts',(114.952856298772,-12.6529756332327,-1.81083777687195));
#54073=CARTESIAN_POINT('Ctrl Pts',(115.000045229627,-12.0359067713131,-3.77713730377714));
#54074=CARTESIAN_POINT('Ctrl Pts',(115.047234160482,-11.4188379093935,-5.74343683068239));
#54075=CARTESIAN_POINT('Ctrl Pts',(115.094423091337,-10.3098672275678,-7.55536654166215));
#54076=CARTESIAN_POINT('Ctrl Pts',(115.141612022192,-8.83962524112239,-8.99949129761083));
#54077=CARTESIAN_POINT('Ctrl Pts',(115.188800953047,-7.36938325467695,-10.4436160535595));
#54078=CARTESIAN_POINT('Ctrl Pts',(115.235989883902,-5.53786996361174,-11.5199358544771));
#54079=CARTESIAN_POINT('Ctrl Pts',(115.283178814757,-3.56082734221149,-12.1016662760128));
#54080=CARTESIAN_POINT('Ctrl Pts',(115.29779279641,-2.94855526754347,-12.2818228837843));
#54081=CARTESIAN_POINT('Ctrl Pts',(115.312406778063,-2.32232570141222,-12.4145441943231));
#54082=CARTESIAN_POINT('Ctrl Pts',(115.327020759716,-1.68956493984086,-12.4995253250381));
#54083=CARTESIAN_POINT('',(113.51273504543,-1.68935314531931,-12.5));
#54084=CARTESIAN_POINT('Ctrl Pts',(113.51273504543,-1.68923172356653,-12.4990204999488));
#54085=CARTESIAN_POINT('Ctrl Pts',(113.512233140265,-1.6800439586769,-12.4990205731998));
#54086=CARTESIAN_POINT('Ctrl Pts',(113.511736968961,-1.670855904336,-12.4990207456443));
#54087=CARTESIAN_POINT('Ctrl Pts',(113.511246535892,-1.66166754556756,-12.4990210174009));
#54088=CARTESIAN_POINT('Ctrl Pts',(113.498080335484,-1.41499622421194,-12.4990283129998));
#54089=CARTESIAN_POINT('Ctrl Pts',(113.489067459873,-1.16843347430942,-12.4991094506017));
#54090=CARTESIAN_POINT('Ctrl Pts',(113.484258366864,-0.921681029186322,
-12.4992529586073));
#54091=CARTESIAN_POINT('Ctrl Pts',(113.48211281744,-0.811593832833913,-12.4993169838857));
#54092=CARTESIAN_POINT('Ctrl Pts',(113.480804008808,-0.70146820779939,-12.4993931672618));
#54093=CARTESIAN_POINT('Ctrl Pts',(113.480336421755,-0.591274738865397,
-12.4994789473658));
#54094=CARTESIAN_POINT('Ctrl Pts',(113.479583440748,-0.413824168452118,
-12.4996170837591));
#54095=CARTESIAN_POINT('Ctrl Pts',(113.481012995891,-0.236458362509808,
-12.4997801223198));
#54096=CARTESIAN_POINT('Ctrl Pts',(113.484624603499,-0.059056775375869,
-12.4999513037557));
#54097=CARTESIAN_POINT('Ctrl Pts',(113.484893902283,-0.0458288622444513,
-12.4999640678645));
#54098=CARTESIAN_POINT('Ctrl Pts',(113.485175322472,-0.0326012711593641,
-12.4999768735535));
#54099=CARTESIAN_POINT('Ctrl Pts',(113.485468860997,-0.0193739522482943,
-12.4999897123243));
#54100=CARTESIAN_POINT('Ctrl Pts',(113.485549513044,-0.0157396410409706,
-12.4999932398788));
#54101=CARTESIAN_POINT('Ctrl Pts',(113.485631079851,-0.0121053538488512,
-12.4999967699262));
#54102=CARTESIAN_POINT('Ctrl Pts',(113.485713561346,-0.00847108973138637,
-12.5000003022872));
#54103=CARTESIAN_POINT('Ctrl Pts',(113.485762014607,-0.00633616302775324,
-12.5000023773515));
#54104=CARTESIAN_POINT('Ctrl Pts',(113.485810783509,-0.00420124466411693,
-12.5000044532139));
#54105=CARTESIAN_POINT('Ctrl Pts',(113.48585986804,-0.00206633441641477,
-12.5000065298378));
#54106=CARTESIAN_POINT('Ctrl Pts',(113.485902246277,-0.000223111464762653,
-12.5000083227379));
#54107=CARTESIAN_POINT('Ctrl Pts',(113.485944859782,0.00162010521623557,
-12.5000101162055));
#54108=CARTESIAN_POINT('Ctrl Pts',(113.485987708546,0.00346331579858671,
-12.500011910217));
#54109=CARTESIAN_POINT('Ctrl Pts',(113.486039892225,0.00570808321031068,
-12.500014095067));
#54110=CARTESIAN_POINT('Ctrl Pts',(113.486092424826,0.00795284120093064,
-12.5000162807233));
#54111=CARTESIAN_POINT('Ctrl Pts',(113.486145306333,0.0101975900499408,
-12.5000184671433));
#54112=CARTESIAN_POINT('Ctrl Pts',(113.486245074839,0.0144326289741938,
-12.5000225921365));
#54113=CARTESIAN_POINT('Ctrl Pts',(113.486346085202,0.018667633424933,-12.5000267198462));
#54114=CARTESIAN_POINT('Ctrl Pts',(113.486448337302,0.0229026050402846,
-12.5000308499837));
#54115=CARTESIAN_POINT('Ctrl Pts',(113.487030769284,0.0470251697744376,
-12.5000543754093));
#54116=CARTESIAN_POINT('Ctrl Pts',(113.487653483087,0.0711464129353356,
-12.5000779795403));
#54117=CARTESIAN_POINT('Ctrl Pts',(113.488316454118,0.0952666358180398,
-12.5001016076708));
#54118=CARTESIAN_POINT('Ctrl Pts',(113.489164107301,0.126105967784969,-12.5001318178294));
#54119=CARTESIAN_POINT('Ctrl Pts',(113.49007754813,0.156942822632197,-12.5001620666217));
#54120=CARTESIAN_POINT('Ctrl Pts',(113.491056714763,0.187777827657472,-12.5001922342553));
#54121=CARTESIAN_POINT('Ctrl Pts',(113.495878510601,0.339621338049009,-12.5003407913702));
#54122=CARTESIAN_POINT('Ctrl Pts',(113.502292094098,0.491355809643231,-12.5004875912149));
#54123=CARTESIAN_POINT('Ctrl Pts',(113.510285968124,0.643054608681126,-12.5006162471355));
#54124=CARTESIAN_POINT('Ctrl Pts',(113.523057368732,0.885415962900539,-12.5008217940703));
#54125=CARTESIAN_POINT('Ctrl Pts',(113.539840399663,1.12726119776551,-12.5009822132088));
#54126=CARTESIAN_POINT('Ctrl Pts',(113.560543745381,1.36886981331526,-12.5010129660893));
#54127=CARTESIAN_POINT('Ctrl Pts',(113.562246397364,1.3887398089245,-12.5010154952193));
#54128=CARTESIAN_POINT('Ctrl Pts',(113.563975564349,1.4086081755581,-12.5010171404161));
#54129=CARTESIAN_POINT('Ctrl Pts',(113.565731195542,1.42847505288237,-12.5010178514909));
#54130=CARTESIAN_POINT('Ctrl Pts',(113.573419321789,1.51547456714083,-12.5010209653754));
#54131=CARTESIAN_POINT('Ctrl Pts',(113.581614944879,1.60244560010039,-12.5010061863381));
#54132=CARTESIAN_POINT('Ctrl Pts',(113.590313799386,1.68940030132012,-12.5009781087056));
#54133=CARTESIAN_POINT('',(111.7760280851,1.68935314531926,-12.5));
#54134=CARTESIAN_POINT('Ctrl Pts',(111.7760280851,1.68925638115339,-12.4991303417189));
#54135=CARTESIAN_POINT('Ctrl Pts',(111.812543987797,3.26988754097161,-12.284116080938));
#54136=CARTESIAN_POINT('Ctrl Pts',(111.849059890495,4.81020923824029,-11.7696927456239));
#54137=CARTESIAN_POINT('Ctrl Pts',(111.885575793192,6.19900628169252,-10.9861999489504));
#54138=CARTESIAN_POINT('Ctrl Pts',(111.932764724047,7.99372701469248,-9.97370444215502));
#54139=CARTESIAN_POINT('Ctrl Pts',(111.979953654902,9.53540173774336,-8.51186322242636));
#54140=CARTESIAN_POINT('Ctrl Pts',(112.027142585757,10.64200964519,-6.77327960690641));
#54141=CARTESIAN_POINT('Ctrl Pts',(112.074331516612,11.7486175526366,-5.03469599138647));
#54142=CARTESIAN_POINT('Ctrl Pts',(112.121520447468,12.420158644479,-3.01936998007523));
#54143=CARTESIAN_POINT('Ctrl Pts',(112.168709378323,12.5777166450503,-0.964573554423232));
#54144=CARTESIAN_POINT('Ctrl Pts',(112.215898309178,12.7352746456215,1.0902228712287));
#54145=CARTESIAN_POINT('Ctrl Pts',(112.263087240033,12.3788495549217,3.18448971122139));
#54146=CARTESIAN_POINT('Ctrl Pts',(112.310276170888,11.5503385958018,5.07146765373859));
#54147=CARTESIAN_POINT('Ctrl Pts',(112.357465101743,10.7218276366819,6.95844559625586));
#54148=CARTESIAN_POINT('Ctrl Pts',(112.404654032598,9.42123080914186,8.63813464129762));
#54149=CARTESIAN_POINT('Ctrl Pts',(112.451842963453,7.80179199338407,9.91270604401158));
#54150=CARTESIAN_POINT('Ctrl Pts',(112.499031894308,6.18235317762629,11.1872774467255));
#54151=CARTESIAN_POINT('Ctrl Pts',(112.546220825163,4.2440723736507,12.0567312071117));
#54152=CARTESIAN_POINT('Ctrl Pts',(112.593409756018,2.21524905293368,12.4186365821184));
#54153=CARTESIAN_POINT('Ctrl Pts',(112.640598686873,0.186425732216652,12.7805419571252));
#54154=CARTESIAN_POINT('Ctrl Pts',(112.687787617728,-1.93294010524181,12.6348989467525));
#54155=CARTESIAN_POINT('Ctrl Pts',(112.734976548583,-3.89319014102203,11.9988699483865));
#54156=CARTESIAN_POINT('Ctrl Pts',(112.782165479439,-5.85344017680225,11.3628409500206));
#54157=CARTESIAN_POINT('Ctrl Pts',(112.829354410294,-7.65457441090422,10.2364259636613));
#54158=CARTESIAN_POINT('Ctrl Pts',(112.876543341149,-9.08443352514128,8.75230731095469));
#54159=CARTESIAN_POINT('Ctrl Pts',(112.923732272004,-10.5142926393783,7.26818865824804));
#54160=CARTESIAN_POINT('Ctrl Pts',(112.970921202859,-11.5728766337505,5.42636633919398));
#54161=CARTESIAN_POINT('Ctrl Pts',(113.018110133714,-12.1354883111685,3.44379808998662));
#54162=CARTESIAN_POINT('Ctrl Pts',(113.065299064569,-12.6980999885865,1.46122984077925));
#54163=CARTESIAN_POINT('Ctrl Pts',(113.112487995424,-12.7647393490503,-0.662084338581423));
#54164=CARTESIAN_POINT('Ctrl Pts',(113.159676926279,-12.3275575619273,-2.67603063058306));
#54165=CARTESIAN_POINT('Ctrl Pts',(113.206865857134,-11.8903757748043,-4.68997692258463));
#54166=CARTESIAN_POINT('Ctrl Pts',(113.254054787989,-10.9493728400946,-6.59455532722717));
#54167=CARTESIAN_POINT('Ctrl Pts',(113.301243718844,-9.6153931900996,-8.1654169007227));
#54168=CARTESIAN_POINT('Ctrl Pts',(113.348432649699,-8.28141354010458,-9.73627847421828));
#54169=CARTESIAN_POINT('Ctrl Pts',(113.395621580554,-6.55445717482431,-10.9734232165668));
#54170=CARTESIAN_POINT('Ctrl Pts',(113.44281051141,-4.6379500495765,-11.7311225730955));
#54171=CARTESIAN_POINT('Ctrl Pts',(113.466118689416,-3.69132361796918,-12.1053754149728));
#54172=CARTESIAN_POINT('Ctrl Pts',(113.489426867423,-2.6984524927118,-12.3626579793741));
#54173=CARTESIAN_POINT('Ctrl Pts',(113.51273504543,-1.68923172356706,-12.4990204999487));
#54174=CARTESIAN_POINT('',(111.680383100847,0.293137397039349,-12.5));
#54175=CARTESIAN_POINT('Ctrl Pts',(111.680383100847,0.293137397039376,-12.5));
#54176=CARTESIAN_POINT('Ctrl Pts',(111.68465314286,0.409731183256787,-12.5000000034602));
#54177=CARTESIAN_POINT('Ctrl Pts',(111.689860597525,0.526270087563317,-12.4999689964682));
#54178=CARTESIAN_POINT('Ctrl Pts',(111.696000254414,0.642788658290244,-12.4999174059816));
#54179=CARTESIAN_POINT('Ctrl Pts',(111.708516098598,0.880314680028347,-12.499812237484));
#54180=CARTESIAN_POINT('Ctrl Pts',(111.724884633411,1.11734811706522,-12.4996240015796));
#54181=CARTESIAN_POINT('Ctrl Pts',(111.74501991605,1.35416465501358,-12.499421500197));
#54182=CARTESIAN_POINT('Ctrl Pts',(111.754520404583,1.46590248574335,-12.4993259533851));
#54183=CARTESIAN_POINT('Ctrl Pts',(111.764859470146,1.57759136494832,-12.4992269184326));
#54184=CARTESIAN_POINT('Ctrl Pts',(111.7760280851,1.68925638115339,-12.4991303417189));
#54185=CARTESIAN_POINT('',(111.185928218469,1.41330412150968,-11.5105178568576));
#54186=CARTESIAN_POINT('Ctrl Pts',(111.185928218469,1.4133810675711,-11.5111948783535));
#54187=CARTESIAN_POINT('Ctrl Pts',(111.194692020162,1.40292731174206,-11.5283132100807));
#54188=CARTESIAN_POINT('Ctrl Pts',(111.203416294175,1.39232321605708,-11.5453647146798));
#54189=CARTESIAN_POINT('Ctrl Pts',(111.296332057201,1.27717818405291,-11.7270809017656));
#54190=CARTESIAN_POINT('Ctrl Pts',(111.378208707921,1.1561743340081,-11.8882169128781));
#54191=CARTESIAN_POINT('Ctrl Pts',(111.492960338586,0.936239464533711,-12.1161930051839));
#54192=CARTESIAN_POINT('Ctrl Pts',(111.532910695054,0.847236652983905,-12.1960892434571));
#54193=CARTESIAN_POINT('Ctrl Pts',(111.617582618094,0.614009366313158,-12.3672109959224));
#54194=CARTESIAN_POINT('Ctrl Pts',(111.657833646957,0.460862322932455,-12.4502435215011));
#54195=CARTESIAN_POINT('Ctrl Pts',(111.680383100847,0.293137397039347,-12.5));
#54196=CARTESIAN_POINT('Ctrl Pts',(111.185928218469,1.41330412150968,-11.5105178568576));
#54197=CARTESIAN_POINT('Ctrl Pts',(111.223614785545,2.91555500390263,-11.3247312662987));
#54198=CARTESIAN_POINT('Ctrl Pts',(111.308490283475,6.2177932578697,-10.2437804539548));
#54199=CARTESIAN_POINT('Ctrl Pts',(111.440554712261,10.1848431574681,-6.48215877251662));
#54200=CARTESIAN_POINT('Ctrl Pts',(111.582121504826,12.0371931123728,-0.923170511755194));
#54201=CARTESIAN_POINT('Ctrl Pts',(111.723688297391,11.0540455303336,4.85356472268307));
#54202=CARTESIAN_POINT('Ctrl Pts',(111.865255089956,7.46653539266892,9.48674646633624));
#54203=CARTESIAN_POINT('Ctrl Pts',(112.006821882522,2.12006530550471,11.8850101815537));
#54204=CARTESIAN_POINT('Ctrl Pts',(112.148388675087,-3.72590191992946,11.4832747896718));
#54205=CARTESIAN_POINT('Ctrl Pts',(112.289955467652,-8.69407282986275,8.37622032266638));
#54206=CARTESIAN_POINT('Ctrl Pts',(112.41094761607,-11.1896532283784,4.03417878282034));
#54207=CARTESIAN_POINT('Ctrl Pts',(112.484750833632,-11.5964486036021,1.06906004117227));
#54208=CARTESIAN_POINT('Ctrl Pts',(112.51136512034,-11.5967929078458,-0.000103121459272826));
#54209=CARTESIAN_POINT('',(117.38636,8.26359861637683,-9.5301578966699));
#54210=CARTESIAN_POINT('Ctrl Pts',(117.38636,8.26387335187489,-9.53028995448194));
#54211=CARTESIAN_POINT('Ctrl Pts',(117.38636,8.47976957198238,-9.32791670058071));
#54212=CARTESIAN_POINT('Ctrl Pts',(117.38636,8.68824929570293,-9.11813352201538));
#54213=CARTESIAN_POINT('Ctrl Pts',(117.38636,8.88884239823733,-8.90122282433969));
#54214=CARTESIAN_POINT('Ctrl Pts',(117.38636,9.08931532045339,-8.68444208325957));
#54215=CARTESIAN_POINT('Ctrl Pts',(117.38636,9.28191144627861,-8.46054188219358));
#54216=CARTESIAN_POINT('Ctrl Pts',(117.38636,9.46637461395972,-8.23002395669524));
#54217=CARTESIAN_POINT('Ctrl Pts',(117.38636,9.60235548331953,-8.06009286255685));
#54218=CARTESIAN_POINT('Ctrl Pts',(117.38636,9.73391591056565,-7.88656480486491));
#54219=CARTESIAN_POINT('Ctrl Pts',(117.38636,9.86093772130342,-7.70963148326641));
#54220=CARTESIAN_POINT('Ctrl Pts',(117.38636,9.93324774835431,-7.60890820435329));
#54221=CARTESIAN_POINT('Ctrl Pts',(117.38636,10.0040866925942,-7.50708124723151));
#54222=CARTESIAN_POINT('Ctrl Pts',(117.38636,10.0734307086138,-7.40418509686393));
#54223=CARTESIAN_POINT('Ctrl Pts',(117.38636,10.1027826310885,-7.3606312330717));
#54224=CARTESIAN_POINT('Ctrl Pts',(117.38636,10.1318666948828,-7.31688579952516));
#54225=CARTESIAN_POINT('Ctrl Pts',(117.38636,10.1606810083502,-7.27295138321782));
#54226=CARTESIAN_POINT('Ctrl Pts',(117.38636,10.1819607036973,-7.24050532146012));
#54227=CARTESIAN_POINT('Ctrl Pts',(117.38636,10.2030931380199,-7.20795631949656));
#54228=CARTESIAN_POINT('Ctrl Pts',(117.38636,10.2240699550889,-7.17531745591445));
#54229=CARTESIAN_POINT('Ctrl Pts',(117.38636,10.3828565791808,-6.92825352122177));
#54230=CARTESIAN_POINT('Ctrl Pts',(117.38636,10.5328439411404,-6.67587035946744));
#54231=CARTESIAN_POINT('Ctrl Pts',(117.38636,10.6737840324592,-6.41866348831899));
#54232=CARTESIAN_POINT('Ctrl Pts',(117.38636,10.8143371275405,-6.16216286115299));
#54233=CARTESIAN_POINT('Ctrl Pts',(117.38636,10.9458928173572,-5.90086440777249));
#54234=CARTESIAN_POINT('Ctrl Pts',(117.38636,11.0681586584076,-5.63523743592315));
#54235=CARTESIAN_POINT('Ctrl Pts',(117.38636,11.1894667796723,-5.37169114502583));
#54236=CARTESIAN_POINT('Ctrl Pts',(117.38636,11.3016302228804,-5.10388332829134));
#54237=CARTESIAN_POINT('Ctrl Pts',(117.38636,11.4043142401143,-4.83225891361791));
#54238=CARTESIAN_POINT('Ctrl Pts',(117.38636,11.4301093636643,-4.76402448410825));
#54239=CARTESIAN_POINT('Ctrl Pts',(117.38636,11.455306027814,-4.69554916125278));
#54240=CARTESIAN_POINT('Ctrl Pts',(117.38636,11.4798984095742,-4.62683992670232));
#54241=CARTESIAN_POINT('Ctrl Pts',(117.38636,11.4917596009721,-4.59370066472471));
#54242=CARTESIAN_POINT('Ctrl Pts',(117.38636,11.5034804972838,-4.56050606622592));
#54243=CARTESIAN_POINT('Ctrl Pts',(117.38636,11.5150549867001,-4.5272728997837));
#54244=CARTESIAN_POINT('Ctrl Pts',(117.38636,11.6106843556848,-4.25269778705742));
#54245=CARTESIAN_POINT('Ctrl Pts',(117.38636,11.6964150816106,-3.97523906689843));
#54246=CARTESIAN_POINT('Ctrl Pts',(117.38636,11.7720112400975,-3.6953694569451));
#54247=CARTESIAN_POINT('Ctrl Pts',(117.38636,11.780970475401,-3.6622008708682));
#54248=CARTESIAN_POINT('Ctrl Pts',(117.38636,11.7897873083534,-3.62899839917189));
#54249=CARTESIAN_POINT('Ctrl Pts',(117.38636,11.7984613009022,-3.59576281126187));
#54250=CARTESIAN_POINT('Ctrl Pts',(117.38636,11.8714983117827,-3.31591152223404));
#54251=CARTESIAN_POINT('Ctrl Pts',(117.38636,11.9344121502825,-3.03371329005597));
#54252=CARTESIAN_POINT('Ctrl Pts',(117.38636,11.9872470138898,-2.74972118066531));
#54253=CARTESIAN_POINT('Ctrl Pts',(117.38636,12.0403084305658,-2.46451132830214));
#54254=CARTESIAN_POINT('Ctrl Pts',(117.38636,12.083204263492,-2.1774915497814));
#54255=CARTESIAN_POINT('Ctrl Pts',(117.38636,12.1159270329586,-1.88921534265928));
#54256=CARTESIAN_POINT('Ctrl Pts',(117.38636,12.1485656405205,-1.60168057261786));
#54257=CARTESIAN_POINT('Ctrl Pts',(117.38636,12.1710834102292,-1.31289520014115));
#54258=CARTESIAN_POINT('Ctrl Pts',(117.38636,12.1834213208703,-1.02341125602325));
#54259=CARTESIAN_POINT('Ctrl Pts',(117.38636,12.1954299880651,-0.741652338792809));
#54260=CARTESIAN_POINT('Ctrl Pts',(117.38636,12.1977946382116,-0.45923111551291));
#54261=CARTESIAN_POINT('Ctrl Pts',(117.38636,12.1904140997534,-0.176667623965072));
#54262=CARTESIAN_POINT('Ctrl Pts',(117.38636,12.188541218074,-0.104964456292086));
#54263=CARTESIAN_POINT('Ctrl Pts',(117.38636,12.1860405744826,-0.0332522057484106));
#54264=CARTESIAN_POINT('Ctrl Pts',(117.38636,12.1829100435733,0.038460452303122));
#54265=CARTESIAN_POINT('Ctrl Pts',(117.38636,12.1810033822858,0.0821373086886409));
#54266=CARTESIAN_POINT('Ctrl Pts',(117.38636,12.178862664041,0.125820640607877));
#54267=CARTESIAN_POINT('Ctrl Pts',(117.38636,12.1764894055144,0.169474133586869));
#54268=CARTESIAN_POINT('Ctrl Pts',(117.38636,12.1608830020532,0.456536843476998));
#54269=CARTESIAN_POINT('Ctrl Pts',(117.38636,12.135218529062,0.742528071737549));
#54270=CARTESIAN_POINT('Ctrl Pts',(117.38636,12.0995281849933,1.0269159598467));
#54271=CARTESIAN_POINT('Ctrl Pts',(117.38636,12.0639225554078,1.31062882580099));
#54272=CARTESIAN_POINT('Ctrl Pts',(117.38636,12.0183385342614,1.59274657006241));
#54273=CARTESIAN_POINT('Ctrl Pts',(117.38636,11.9627566092262,1.8727375600685));
#54274=CARTESIAN_POINT('Ctrl Pts',(117.38636,11.93197934801,2.02777637587353));
#54275=CARTESIAN_POINT('Ctrl Pts',(117.38636,11.8981356764896,2.18216298153699));
#54276=CARTESIAN_POINT('Ctrl Pts',(117.38636,11.8612155579909,2.33580559846095));
#54277=CARTESIAN_POINT('Ctrl Pts',(117.38636,11.7942814757869,2.61435095447361));
#54278=CARTESIAN_POINT('Ctrl Pts',(117.38636,11.7172385264076,2.89045234807707));
#54279=CARTESIAN_POINT('Ctrl Pts',(117.38636,11.6303372664751,3.16361450639462));
#54280=CARTESIAN_POINT('Ctrl Pts',(117.38636,11.5436997487744,3.43594762728112));
#54281=CARTESIAN_POINT('Ctrl Pts',(117.38636,11.4472633370757,3.70535986996651));
#54282=CARTESIAN_POINT('Ctrl Pts',(117.38636,11.3412316896956,3.97133458703356));
#54283=CARTESIAN_POINT('Ctrl Pts',(117.38636,11.2770779669014,4.13226076983449));
#54284=CARTESIAN_POINT('Ctrl Pts',(117.38636,11.209410806186,4.29192801665162));
#54285=CARTESIAN_POINT('Ctrl Pts',(117.38636,11.138268112713,4.45021599479794));
#54286=CARTESIAN_POINT('Ctrl Pts',(117.38636,11.1166612236889,4.49828995166837));
#54287=CARTESIAN_POINT('Ctrl Pts',(117.38636,11.0947337121375,4.54623664889386));
#54288=CARTESIAN_POINT('Ctrl Pts',(117.38636,11.072486547347,4.59405262188719));
#54289=CARTESIAN_POINT('Ctrl Pts',(117.38636,11.0566186236401,4.62815765138553));
#54290=CARTESIAN_POINT('Ctrl Pts',(117.38636,11.0405865692041,4.66219923462761));
#54291=CARTESIAN_POINT('Ctrl Pts',(117.38636,11.0244019262929,4.69615293251817));
#54292=CARTESIAN_POINT('Ctrl Pts',(117.38636,10.9021816861498,4.95255828744005));
#54293=CARTESIAN_POINT('Ctrl Pts',(117.38636,10.7711447000552,5.20421392423024));
#54294=CARTESIAN_POINT('Ctrl Pts',(117.38636,10.6315896890138,5.45066746458217));
#54295=CARTESIAN_POINT('Ctrl Pts',(117.38636,10.491931120956,5.69730388617308));
#54296=CARTESIAN_POINT('Ctrl Pts',(117.38636,10.3437415528983,5.93873103356036));
#54297=CARTESIAN_POINT('Ctrl Pts',(117.38636,10.1872735402806,6.17447234971671));
#54298=CARTESIAN_POINT('Ctrl Pts',(117.38636,10.0322804114542,6.40799154366195));
#54299=CARTESIAN_POINT('Ctrl Pts',(117.38636,9.86916379395795,6.63593206668975));
#54300=CARTESIAN_POINT('Ctrl Pts',(117.38636,9.69812859331579,6.85780045134778));
#54301=CARTESIAN_POINT('Ctrl Pts',(117.38636,9.5309508879448,7.07466485880448));
#54302=CARTESIAN_POINT('Ctrl Pts',(117.38636,9.3562073581532,7.28572828240745));
#54303=CARTESIAN_POINT('Ctrl Pts',(117.38636,9.1740562320771,7.4904949660174));
#54304=CARTESIAN_POINT('Ctrl Pts',(117.38636,9.01491680449495,7.6693928598683));
#54305=CARTESIAN_POINT('Ctrl Pts',(117.38636,8.85012236963218,7.84348396232437));
#54306=CARTESIAN_POINT('Ctrl Pts',(117.38636,8.67992675680234,8.01255267463112));
#54307=CARTESIAN_POINT('Ctrl Pts',(117.38636,8.60546617618929,8.08652023626532));
#54308=CARTESIAN_POINT('Ctrl Pts',(117.38636,8.52997160945683,8.15952617938624));
#54309=CARTESIAN_POINT('Ctrl Pts',(117.38636,8.45346361051115,8.23155099082254));
#54310=CARTESIAN_POINT('Ctrl Pts',(117.38636,8.42152310743143,8.26161985608107));
#54311=CARTESIAN_POINT('Ctrl Pts',(117.38636,8.38940596978659,8.29151770990631));
#54312=CARTESIAN_POINT('Ctrl Pts',(117.38636,8.35711367457556,8.32124308435686));
#54313=CARTESIAN_POINT('Ctrl Pts',(117.38636,8.33422258085946,8.34231456062843));
#54314=CARTESIAN_POINT('Ctrl Pts',(117.38636,8.31124267485234,8.36330003679656));
#54315=CARTESIAN_POINT('Ctrl Pts',(117.38636,8.28818716392733,8.38418763817203));
#54316=CARTESIAN_POINT('Ctrl Pts',(117.38636,8.0816610990473,8.57129405845009));
#54317=CARTESIAN_POINT('Ctrl Pts',(117.38636,7.86883968089771,8.75076473777949));
#54318=CARTESIAN_POINT('Ctrl Pts',(117.38636,7.65020289170389,8.92236157727182));
#54319=CARTESIAN_POINT('Ctrl Pts',(117.38636,7.43004610510815,9.09515138502521));
#54320=CARTESIAN_POINT('Ctrl Pts',(117.38636,7.2039922968932,9.25995785654159));
#54321=CARTESIAN_POINT('Ctrl Pts',(117.38636,6.97249670012354,9.41649834374283));
#54322=CARTESIAN_POINT('Ctrl Pts',(117.38636,6.74151605838306,9.57269061131363));
#54323=CARTESIAN_POINT('Ctrl Pts',(117.38636,6.50511726314233,9.72065393525675));
#54324=CARTESIAN_POINT('Ctrl Pts',(117.38636,6.26372598957658,9.86006336558048));
#54325=CARTESIAN_POINT('Ctrl Pts',(117.38636,6.02418010005166,9.99840704098249));
#54326=CARTESIAN_POINT('Ctrl Pts',(117.38636,5.77971723647088,10.1283273663033));
#54327=CARTESIAN_POINT('Ctrl Pts',(117.38636,5.53073534339514,10.2494590853848));
#54328=CARTESIAN_POINT('Ctrl Pts',(117.38636,5.28612776267642,10.3684626658734));
#54329=CARTESIAN_POINT('Ctrl Pts',(117.38636,5.03715804284583,10.478983895787));
#54330=CARTESIAN_POINT('Ctrl Pts',(117.38636,4.78419373222444,10.5806272791542));
#54331=CARTESIAN_POINT('Ctrl Pts',(117.38636,4.68063194659597,10.6222393557866));
#54332=CARTESIAN_POINT('Ctrl Pts',(117.38636,4.57640058419126,10.6623628910523));
#54333=CARTESIAN_POINT('Ctrl Pts',(117.38636,4.47152467205382,10.7009682121205));
#54334=CARTESIAN_POINT('Ctrl Pts',(117.218885227957,1.68953572661212,-12.4994363787171));
#54335=CARTESIAN_POINT('Ctrl Pts',(117.234294788862,2.3567517695111,-12.4097921526067));
#54336=CARTESIAN_POINT('Ctrl Pts',(117.249704349766,3.01671750224669,-12.267108816008));
#54337=CARTESIAN_POINT('Ctrl Pts',(117.26511391067,3.66073026855528,-12.0718164881636));
#54338=CARTESIAN_POINT('Ctrl Pts',(117.30552927378,5.34981212877998,-11.559614330598));
#54339=CARTESIAN_POINT('Ctrl Pts',(117.34594463689,6.92915678414743,-10.6855256438983));
#54340=CARTESIAN_POINT('Ctrl Pts',(117.38636,8.26387335187462,-9.53028995448217));
#54341=CARTESIAN_POINT('Ctrl Pts',(95.8594371265034,-5.05456119273957,10.438230919004));
#54342=CARTESIAN_POINT('Ctrl Pts',(95.9067535451842,-6.76502131585771,9.60996553312322));
#54343=CARTESIAN_POINT('Ctrl Pts',(96.001386382546,-9.76939938124694,7.09734914354963));
#54344=CARTESIAN_POINT('Ctrl Pts',(96.1433356385887,-11.962745016736,1.64472530342245));
#54345=CARTESIAN_POINT('Ctrl Pts',(96.2852848946312,-11.3224897112199,-4.19650321983491));
#54346=CARTESIAN_POINT('Ctrl Pts',(96.427234150674,-8.00081238047729,-9.04430323897844));
#54347=CARTESIAN_POINT('Ctrl Pts',(96.5691834067165,-2.78415884399867,-11.7498524979654));
#54348=CARTESIAN_POINT('Ctrl Pts',(96.7111326627592,3.091848831559,-11.6726995174351));
#54349=CARTESIAN_POINT('Ctrl Pts',(96.8530819188018,8.23560924484923,-8.83096106044612));
#54350=CARTESIAN_POINT('Ctrl Pts',(96.9950311748445,11.4288580805009,-3.8977427059358));
#54351=CARTESIAN_POINT('Ctrl Pts',(97.136980430887,11.915327242442,1.95861959274003));
#54352=CARTESIAN_POINT('Ctrl Pts',(97.2789296869297,9.5797960279637,7.35110139990983));
#54353=CARTESIAN_POINT('Ctrl Pts',(97.4208789429723,4.97540930776886,11.0025682116464));
#54354=CARTESIAN_POINT('Ctrl Pts',(97.562828199015,-0.807342216722395,12.0482111751727));
#54355=CARTESIAN_POINT('Ctrl Pts',(97.7047774550576,-6.39888446344168,10.2403845654334));
#54356=CARTESIAN_POINT('Ctrl Pts',(97.8467267111003,-10.474929971616,6.00724889591607));
#54357=CARTESIAN_POINT('Ctrl Pts',(97.9886759671429,-12.0701174780218,0.351370572132009));
#54358=CARTESIAN_POINT('Ctrl Pts',(98.1306252231855,-10.8066465790285,-5.38772560594593));
#54359=CARTESIAN_POINT('Ctrl Pts',(98.2725744792281,-6.98375473307958,-9.85080540269698));
#54360=CARTESIAN_POINT('Ctrl Pts',(98.4145237352708,-1.50684673412838,-11.9808434723489));
#54361=CARTESIAN_POINT('Ctrl Pts',(98.5564729913134,4.32693932863066,-11.2733665501931));
#54362=CARTESIAN_POINT('Ctrl Pts',(98.6984222473561,9.13594318590594,-7.89593182926991));
#54363=CARTESIAN_POINT('Ctrl Pts',(98.8403715033986,11.781211598614,-2.64844305476444));
#54364=CARTESIAN_POINT('Ctrl Pts',(98.9823207594414,11.6362453734974,3.22629678599122));
#54365=CARTESIAN_POINT('Ctrl Pts',(99.124270015484,8.73537797318143,8.33692803205455));
#54366=CARTESIAN_POINT('Ctrl Pts',(99.2662192715265,3.76564405694391,11.4730607154675));
#54367=CARTESIAN_POINT('Ctrl Pts',(99.4081685275693,-2.0959362022484,11.8919404968782));
#54368=CARTESIAN_POINT('Ctrl Pts',(99.5501177836118,-7.46111982681854,9.49436086710135));
#54369=CARTESIAN_POINT('Ctrl Pts',(99.6920670396545,-11.0592292586176,4.84815898566623));
#54370=CARTESIAN_POINT('Ctrl Pts',(99.8340162956972,-12.0380966639746,-0.946269546045479));
#54371=CARTESIAN_POINT('Ctrl Pts',(99.9759655517397,-10.1658893729505,-6.51658580867914));
#54372=CARTESIAN_POINT('Ctrl Pts',(100.117914807782,-5.88601658741872,-10.5435291092497));
#54373=CARTESIAN_POINT('Ctrl Pts',(100.259864063825,-0.212113381356825,
-12.0733676022228));
#54374=CARTESIAN_POINT('Ctrl Pts',(100.401813319868,5.51202626250981,-10.7437779121853));
#54375=CARTESIAN_POINT('Ctrl Pts',(100.54376257591,9.93071048086492,-6.8696569557873));
#54376=CARTESIAN_POINT('Ctrl Pts',(100.685711831953,11.997428424203,-1.36854249151505));
#54377=CARTESIAN_POINT('Ctrl Pts',(100.827661087996,11.2227034420802,4.45669437992771));
#54378=CARTESIAN_POINT('Ctrl Pts',(100.969610344038,7.7900195897285,9.22641816397909));
#54379=CARTESIAN_POINT('Ctrl Pts',(101.111559600081,2.51236569298111,11.8109786203214));
#54380=CARTESIAN_POINT('Ctrl Pts',(101.253508856124,-3.3603110263314,11.5982544872611));
#54381=CARTESIAN_POINT('Ctrl Pts',(101.395458112166,-8.43713953088349,8.63862685161016));
#54382=CARTESIAN_POINT('Ctrl Pts',(101.537407368209,-11.5157356156619,3.63304700976087));
#54383=CARTESIAN_POINT('Ctrl Pts',(101.679356624251,-11.866971774659,-2.23297520013184));
#54384=CARTESIAN_POINT('Ctrl Pts',(101.821305880294,-9.40766205636401,-7.57014477921035));
#54385=CARTESIAN_POINT('Ctrl Pts',(101.963255136337,-4.72026363022087,-11.1144189504522));
#54386=CARTESIAN_POINT('Ctrl Pts',(102.105204392379,1.08507100893144,-12.0263800975411));
#54387=CARTESIAN_POINT('Ctrl Pts',(102.247153648422,6.63341996474086,-10.0900414724784));
#54388=CARTESIAN_POINT('Ctrl Pts',(102.389102904465,10.610725229854,-5.76400099249621));
#54389=CARTESIAN_POINT('Ctrl Pts',(102.531052160507,12.0750111151176,-0.0728279804925511));
#54390=CARTESIAN_POINT('Ctrl Pts',(102.67300141655,10.6794795716148,5.63559344030584));
#54391=CARTESIAN_POINT('Ctrl Pts',(102.814950672592,6.75464503055027,10.0092940738206));
#54392=CARTESIAN_POINT('Ctrl Pts',(102.956899928635,1.23005613734974,12.0124168777114));
#54393=CARTESIAN_POINT('Ctrl Pts',(103.098849184678,-4.58585637836471,11.1705469258209));
#54394=CARTESIAN_POINT('Ctrl Pts',(103.24079844072,-9.31566538066349,7.68307073119021));
#54395=CARTESIAN_POINT('Ctrl Pts',(103.382747696763,-11.8391739529085,2.37595401001747));
#54396=CARTESIAN_POINT('Ctrl Pts',(103.524696952806,-11.5587202190389,-3.49387810934367));
#54397=CARTESIAN_POINT('Ctrl Pts',(103.666646208848,-8.54072618632016,-8.53622829798181));
#54398=CARTESIAN_POINT('Ctrl Pts',(103.808595464891,-3.49996651231003,-11.5568781146813));
#54399=CARTESIAN_POINT('Ctrl Pts',(103.950544720934,2.36971705558015,-11.8404239122457));
#54400=CARTESIAN_POINT('Ctrl Pts',(104.092493976976,7.67816237096933,-9.3197113662083));
#54401=CARTESIAN_POINT('Ctrl Pts',(104.234443233019,11.168129644454,-4.59174014842598));
#54402=CARTESIAN_POINT('Ctrl Pts',(104.376392489061,12.0130631783326,1.22372808128535));
#54403=CARTESIAN_POINT('Ctrl Pts',(104.518341745104,10.0128508883889,6.74937141017876));
#54404=CARTESIAN_POINT('Ctrl Pts',(104.660291001147,5.64121838056578,10.6765093795372));
#54405=CARTESIAN_POINT('Ctrl Pts',(104.802240257189,-0.0664671110029323,
12.0750478032933));
#54406=CARTESIAN_POINT('Ctrl Pts',(104.944189513232,-5.75841068985474,10.6137601120454));
#54407=CARTESIAN_POINT('Ctrl Pts',(105.086138769275,-10.0865457254805,6.63873426049027));
#54408=CARTESIAN_POINT('Ctrl Pts',(105.228088025317,-12.0258068420377,1.09140610544123));
#54409=CARTESIAN_POINT('Ctrl Pts',(105.37003728136,-11.1169039314122,-4.71440814863962));
#54410=CARTESIAN_POINT('Ctrl Pts',(105.511986537402,-7.57509950853803,-9.40367293367282));
#54411=CARTESIAN_POINT('Ctrl Pts',(105.653935793445,-2.23922610928576,-11.8657938991006));
#54412=CARTESIAN_POINT('Ctrl Pts',(105.795885049488,3.6269801590525,-11.5176477156709));
#54413=CARTESIAN_POINT('Ctrl Pts',(105.93783430553,8.63418136051829,-8.44168924241129));
#54414=CARTESIAN_POINT('Ctrl Pts',(106.079783561573,11.5964822941979,-3.36641977915706));
#54415=CARTESIAN_POINT('Ctrl Pts',(106.221732817616,11.8123013659403,2.50614254258396));
#54416=CARTESIAN_POINT('Ctrl Pts',(106.363682073658,9.23051857694247,7.78516037256956));
#54417=CARTESIAN_POINT('Ctrl Pts',(106.505631329701,4.46260964811663,11.2203497277713));
#54418=CARTESIAN_POINT('Ctrl Pts',(106.647580585744,-1.36223065258046,11.9981569780826));
#54419=CARTESIAN_POINT('Ctrl Pts',(106.789529841786,-6.86440734641473,9.9343085302927));
#54420=CARTESIAN_POINT('Ctrl Pts',(106.931479097829,-10.7409089746491,5.51772545751394));
#54421=CARTESIAN_POINT('Ctrl Pts',(107.073428353871,-12.0734023240826,-0.205836963644071));
#54422=CARTESIAN_POINT('Ctrl Pts',(107.215377609914,-10.5467853781223,-5.88028127277808));
#54423=CARTESIAN_POINT('Ctrl Pts',(107.357326865957,-6.5216081564048,-10.1627828959428));
#54424=CARTESIAN_POINT('Ctrl Pts',(107.451959703319,-2.80945746568101,-11.4115686783349));
#54425=CARTESIAN_POINT('Ctrl Pts',(107.499276121999,-0.914933857717795,
-11.5614942635285));
#54426=CARTESIAN_POINT('Ctrl Pts',(96.0549664176689,-5.20216116916647,10.7430412831157));
#54427=CARTESIAN_POINT('Ctrl Pts',(96.1022828363498,-6.96256902547539,9.89058943538993));
#54428=CARTESIAN_POINT('Ctrl Pts',(96.1969156737116,-10.0546789660402,7.30460127213921));
#54429=CARTESIAN_POINT('Ctrl Pts',(96.3388649297541,-12.312073240323,1.69275349157906));
#54430=CARTESIAN_POINT('Ctrl Pts',(96.4808141857969,-11.6531216198553,-4.3190467508565));
#54431=CARTESIAN_POINT('Ctrl Pts',(96.6227634418394,-8.23444684917279,-9.30840904242357));
#54432=CARTESIAN_POINT('Ctrl Pts',(96.7647126978821,-2.86546002209765,-12.0929639740338));
#54433=CARTESIAN_POINT('Ctrl Pts',(96.9066619539248,3.1821349706029,-12.0135580228354));
#54434=CARTESIAN_POINT('Ctrl Pts',(97.0486112099673,8.47610009737803,-9.08883698570373));
#54435=CARTESIAN_POINT('Ctrl Pts',(97.19056046601,11.7625960883999,-4.01156202863798));
#54436=CARTESIAN_POINT('Ctrl Pts',(97.3325097220526,12.2632708033251,2.01581391578688));
#54437=CARTESIAN_POINT('Ctrl Pts',(97.4744589780952,9.85953894015421,7.56576343524082));
#54438=CARTESIAN_POINT('Ctrl Pts',(97.6164082341379,5.12069794283293,11.3238579827559));
#54439=CARTESIAN_POINT('Ctrl Pts',(97.7583574901805,-0.830917693922621,
12.4000351253895));
#54440=CARTESIAN_POINT('Ctrl Pts',(97.9003067462231,-6.58574048515116,10.5394175502613));
#54441=CARTESIAN_POINT('Ctrl Pts',(98.0422560022659,-10.7808119973604,6.18266863298474));
#54442=CARTESIAN_POINT('Ctrl Pts',(98.1842052583084,-12.4225811217076,0.361631064820941));
#54443=CARTESIAN_POINT('Ctrl Pts',(98.3261545143511,-11.1222151752916,-5.54505443076548));
#54444=CARTESIAN_POINT('Ctrl Pts',(98.4681037703937,-7.1876897522964,-10.1384621526662));
#54445=CARTESIAN_POINT('Ctrl Pts',(98.6100530264363,-1.55084868285458,-12.3307001951508));
#54446=CARTESIAN_POINT('Ctrl Pts',(98.7520022824789,4.45329176923893,-11.6025639965412));
#54447=CARTESIAN_POINT('Ctrl Pts',(98.8939515385216,9.40272499889778,-8.12650364498813));
#54448=CARTESIAN_POINT('Ctrl Pts',(99.0359007945642,12.125238802545,-2.72578114951593));
#54449=CARTESIAN_POINT('Ctrl Pts',(99.1778500506069,11.9760393689273,3.32050898590334));
#54450=CARTESIAN_POINT('Ctrl Pts',(99.3197993066495,8.99046274389779,8.58037752926741));
#54451=CARTESIAN_POINT('Ctrl Pts',(99.4617485626922,3.87560592165246,11.8080894996832));
#54452=CARTESIAN_POINT('Ctrl Pts',(99.6036978187347,-2.15714035474506,12.2392011333763));
#54453=CARTESIAN_POINT('Ctrl Pts',(99.7456470747775,-7.67899454799881,9.77160895783289));
#54454=CARTESIAN_POINT('Ctrl Pts',(99.8875963308201,-11.3821736084093,4.98973174039441));
#54455=CARTESIAN_POINT('Ctrl Pts',(100.029545586863,-12.389625256878,-0.973901887877716));
#54456=CARTESIAN_POINT('Ctrl Pts',(100.171494842905,-10.4627469980914,-6.70687886777328));
#54457=CARTESIAN_POINT('Ctrl Pts',(100.313444098948,-6.05789617823254,-10.8514143219596));
#54458=CARTESIAN_POINT('Ctrl Pts',(100.455393354991,-0.218307377016261,
-12.4259261539011));
#54459=CARTESIAN_POINT('Ctrl Pts',(100.597342611033,5.67298483346935,-11.0575106589274));
#54460=CARTESIAN_POINT('Ctrl Pts',(100.739291867076,10.2207005664501,-7.07026016664399));
#54461=CARTESIAN_POINT('Ctrl Pts',(100.881241123118,12.3477694498769,-1.40850577057814));
#54462=CARTESIAN_POINT('Ctrl Pts',(101.023190379161,11.5504214576176,4.58683584232886));
#54463=CARTESIAN_POINT('Ctrl Pts',(101.165139635204,8.01749862578424,9.49584196786224));
#54464=CARTESIAN_POINT('Ctrl Pts',(101.307088891246,2.58573014598101,12.155875061271));
#54465=CARTESIAN_POINT('Ctrl Pts',(101.449038147289,-3.45843662207766,11.9369390977812));
#54466=CARTESIAN_POINT('Ctrl Pts',(101.590987403332,-8.68351533847242,8.89088635961457));
#54467=CARTESIAN_POINT('Ctrl Pts',(101.732936659374,-11.8520105642869,3.73913686257913));
#54468=CARTESIAN_POINT('Ctrl Pts',(101.874885915417,-12.2135032909288,-2.29818107544593));
#54469=CARTESIAN_POINT('Ctrl Pts',(102.01683517146,-9.68237842536282,-7.79120317544952));
#54470=CARTESIAN_POINT('Ctrl Pts',(102.158784427502,-4.85810166877311,-11.4389749133797));
#54471=CARTESIAN_POINT('Ctrl Pts',(102.300733683545,1.11675653992664,-12.3775665509662));
#54472=CARTESIAN_POINT('Ctrl Pts',(102.442682939587,6.82712473813086,-10.384684237042));
#54473=CARTESIAN_POINT('Ctrl Pts',(102.58463219563,10.9205726595475,-5.93231756403941));
#54474=CARTESIAN_POINT('Ctrl Pts',(102.726581451673,12.4276176595801,-0.0749546553499881));
#54475=CARTESIAN_POINT('Ctrl Pts',(102.868530707715,10.9913347204428,5.80016033884008));
#54476=CARTESIAN_POINT('Ctrl Pts',(103.010479963758,6.95188973869892,10.3015789058784));
#54477=CARTESIAN_POINT('Ctrl Pts',(103.152429219801,1.26597542884778,12.3631955863612));
#54478=CARTESIAN_POINT('Ctrl Pts',(103.294378475843,-4.71976954461859,11.4967419010237));
#54479=CARTESIAN_POINT('Ctrl Pts',(103.436327731886,-9.58769532315621,7.90742671691631));
#54480=CARTESIAN_POINT('Ctrl Pts',(103.578276987929,-12.1848937354434,2.44533505863823));
#54481=CARTESIAN_POINT('Ctrl Pts',(103.720226243971,-11.8962503758221,-3.59590404332945));
#54482=CARTESIAN_POINT('Ctrl Pts',(103.862175500014,-8.79012686339186,-8.78549763067218));
#54483=CARTESIAN_POINT('Ctrl Pts',(104.004124756056,-3.60217023584078,-11.8943544795427));
#54484=CARTESIAN_POINT('Ctrl Pts',(104.146074012099,2.43891597675345,-12.1861801952723));
#54485=CARTESIAN_POINT('Ctrl Pts',(104.288023268142,7.90237502598375,-9.59185945691376));
#54486=CARTESIAN_POINT('Ctrl Pts',(104.429972524184,11.4942540317939,-4.72582512866913));
#54487=CARTESIAN_POINT('Ctrl Pts',(104.571921780227,12.3638607598287,1.25946258504604));
#54488=CARTESIAN_POINT('Ctrl Pts',(104.71387103627,10.3052395842098,6.94646212152869));
#54489=CARTESIAN_POINT('Ctrl Pts',(104.855820292312,5.80594953491142,10.9882777947668));
#54490=CARTESIAN_POINT('Ctrl Pts',(104.997769548355,-0.0684080399269323,
12.4276554190998));
#54491=CARTESIAN_POINT('Ctrl Pts',(105.139718804398,-5.92656401705154,10.9236961643755));
#54492=CARTESIAN_POINT('Ctrl Pts',(105.28166806044,-10.3810864095359,6.83259421845467));
#54493=CARTESIAN_POINT('Ctrl Pts',(105.423617316483,-12.376976555632,1.12327662976425));
#54494=CARTESIAN_POINT('Ctrl Pts',(105.565566572526,-11.4415324591217,-4.85207519926421));
#54495=CARTESIAN_POINT('Ctrl Pts',(105.707515828568,-7.79630258952909,-9.6782728149306));
#54496=CARTESIAN_POINT('Ctrl Pts',(105.849465084611,-2.30461451954379,-12.2122910198219));
#54497=CARTESIAN_POINT('Ctrl Pts',(105.991414340653,3.73289285168067,-11.8539785001846));
#54498=CARTESIAN_POINT('Ctrl Pts',(106.133363596696,8.88631105421133,-8.68819790768832));
#54499=CARTESIAN_POINT('Ctrl Pts',(106.275312852739,11.9351151543,-3.46472375869151));
#54500=CARTESIAN_POINT('Ctrl Pts',(106.417262108781,12.1572364328389,2.57932527123291));
#54501=CARTESIAN_POINT('Ctrl Pts',(106.559211364824,9.5000621183921,8.01249751295703));
#54502=CARTESIAN_POINT('Ctrl Pts',(106.701160620867,4.59292384429468,11.5479990116893));
#54503=CARTESIAN_POINT('Ctrl Pts',(106.843109876909,-1.40200961746818,12.3485192785084));
#54504=CARTESIAN_POINT('Ctrl Pts',(106.985059132952,-7.06485726162612,10.2244036837543));
#54505=CARTESIAN_POINT('Ctrl Pts',(107.127008388994,-11.0545579445614,5.67885045262314));
#54506=CARTESIAN_POINT('Ctrl Pts',(107.268957645037,-12.4259618896858,-0.211847679475389));
#54507=CARTESIAN_POINT('Ctrl Pts',(107.41090690108,-10.8547656782573,-6.05199338470034));
#54508=CARTESIAN_POINT('Ctrl Pts',(107.552856157122,-6.71204787479888,-10.4595498077822));
#54509=CARTESIAN_POINT('Ctrl Pts',(107.647488994484,-2.89149739751578,-11.7448018124665));
#54510=CARTESIAN_POINT('Ctrl Pts',(107.694805413165,-0.941651155358861,
-11.899105426137));
#54511=CARTESIAN_POINT('Ctrl Pts',(96.2504957088345,-5.34976114559336,11.0478516472273));
#54512=CARTESIAN_POINT('Ctrl Pts',(96.2978121275154,-7.16011673509306,10.1712133376566));
#54513=CARTESIAN_POINT('Ctrl Pts',(96.3924449648771,-10.3399585508335,7.51185340072878));
#54514=CARTESIAN_POINT('Ctrl Pts',(96.5343942209198,-12.6614014639099,1.74078167973567));
#54515=CARTESIAN_POINT('Ctrl Pts',(96.6763434769622,-11.9837535284907,-4.44159028187809));
#54516=CARTESIAN_POINT('Ctrl Pts',(96.8182927330052,-8.46808131786831,-9.57251484586868));
#54517=CARTESIAN_POINT('Ctrl Pts',(96.9602419890475,-2.94676120019661,-12.4360754501023));
#54518=CARTESIAN_POINT('Ctrl Pts',(97.1021912450904,3.2724211096468,-12.3544165282358));
#54519=CARTESIAN_POINT('Ctrl Pts',(97.2441405011329,8.71659094990683,-9.34671291096133));
#54520=CARTESIAN_POINT('Ctrl Pts',(97.3860897571755,12.0963340962989,-4.12538135134016));
#54521=CARTESIAN_POINT('Ctrl Pts',(97.5280390132182,12.6112143642082,2.07300823883373));
#54522=CARTESIAN_POINT('Ctrl Pts',(97.6699882692608,10.1392818523447,7.7804254705718));
#54523=CARTESIAN_POINT('Ctrl Pts',(97.8119375253035,5.26598657789702,11.6451477538654));
#54524=CARTESIAN_POINT('Ctrl Pts',(97.9538867813461,-0.854493171122856,
12.7518590756063));
#54525=CARTESIAN_POINT('Ctrl Pts',(98.0958360373887,-6.77259650686064,10.8384505350893));
#54526=CARTESIAN_POINT('Ctrl Pts',(98.2377852934314,-11.0866940231047,6.35808837005341));
#54527=CARTESIAN_POINT('Ctrl Pts',(98.379734549474,-12.7750447653935,0.371891557509875));
#54528=CARTESIAN_POINT('Ctrl Pts',(98.5216838055166,-11.4377837715547,-5.70238325558503));
#54529=CARTESIAN_POINT('Ctrl Pts',(98.6636330615593,-7.39162477151322,-10.4261189026355));
#54530=CARTESIAN_POINT('Ctrl Pts',(98.8055823176019,-1.59485063158079,-12.6805569179526));
#54531=CARTESIAN_POINT('Ctrl Pts',(98.9475315736445,4.5796442098472,-11.9317614428894));
#54532=CARTESIAN_POINT('Ctrl Pts',(99.0894808296872,9.66950681188962,-8.35707546070634));
#54533=CARTESIAN_POINT('Ctrl Pts',(99.2314300857298,12.4692660064759,-2.80311924426744));
#54534=CARTESIAN_POINT('Ctrl Pts',(99.3733793417725,12.3158333643572,3.41472118581547));
#54535=CARTESIAN_POINT('Ctrl Pts',(99.5153285978151,9.24554751461416,8.82382702648026));
#54536=CARTESIAN_POINT('Ctrl Pts',(99.6572778538577,3.98556778636102,12.143118283899));
#54537=CARTESIAN_POINT('Ctrl Pts',(99.7992271099004,-2.21834450724171,12.5864617698744));
#54538=CARTESIAN_POINT('Ctrl Pts',(99.941176365943,-7.89686926917907,10.0488570485644));
#54539=CARTESIAN_POINT('Ctrl Pts',(100.083125621986,-11.7051179582011,5.1313044951226));
#54540=CARTESIAN_POINT('Ctrl Pts',(100.225074878028,-12.7411538497813,-1.00153422970996));
#54541=CARTESIAN_POINT('Ctrl Pts',(100.367024134071,-10.7596046232323,-6.89717192686741));
#54542=CARTESIAN_POINT('Ctrl Pts',(100.508973390114,-6.22977576904636,-11.1592995346694));
#54543=CARTESIAN_POINT('Ctrl Pts',(100.650922646156,-0.224501372675697,
-12.7784847055794));
#54544=CARTESIAN_POINT('Ctrl Pts',(100.792871902199,5.83394340442888,-11.3712434056696));
#54545=CARTESIAN_POINT('Ctrl Pts',(100.934821158242,10.5106906520353,-7.2708633775007));
#54546=CARTESIAN_POINT('Ctrl Pts',(101.076770414284,12.6981104755508,-1.44846904964124));
#54547=CARTESIAN_POINT('Ctrl Pts',(101.218719670327,11.8781394731551,4.71697730473001));
#54548=CARTESIAN_POINT('Ctrl Pts',(101.360668926369,8.24497766183999,9.76526577174539));
#54549=CARTESIAN_POINT('Ctrl Pts',(101.502618182412,2.65909459898092,12.5007715022207));
#54550=CARTESIAN_POINT('Ctrl Pts',(101.644567438455,-3.55656221782393,12.2756237083013));
#54551=CARTESIAN_POINT('Ctrl Pts',(101.786516694497,-8.92989114606135,9.14314586761896));
#54552=CARTESIAN_POINT('Ctrl Pts',(101.92846595054,-12.1882855129119,3.84522671539739));
#54553=CARTESIAN_POINT('Ctrl Pts',(102.070415206582,-12.5600348071986,-2.36338695076003));
#54554=CARTESIAN_POINT('Ctrl Pts',(102.212364462625,-9.95709479436164,-8.01226157168866));
#54555=CARTESIAN_POINT('Ctrl Pts',(102.354313718668,-4.99593970732534,-11.7635308763072));
#54556=CARTESIAN_POINT('Ctrl Pts',(102.49626297471,1.14844207092185,-12.7287530043913));
#54557=CARTESIAN_POINT('Ctrl Pts',(102.638212230753,7.02082951152085,-10.6793270016055));
#54558=CARTESIAN_POINT('Ctrl Pts',(102.780161486796,11.230420089241,-6.1006341355826));
#54559=CARTESIAN_POINT('Ctrl Pts',(102.922110742838,12.7802242040426,-0.0770813302074385));
#54560=CARTESIAN_POINT('Ctrl Pts',(103.064059998881,11.3031898692709,5.96472723737434));
#54561=CARTESIAN_POINT('Ctrl Pts',(103.206009254924,7.14913444684757,10.5938637379362));
#54562=CARTESIAN_POINT('Ctrl Pts',(103.347958510966,1.30189472034582,12.713974295011));
#54563=CARTESIAN_POINT('Ctrl Pts',(103.489907767009,-4.85368271087248,11.8229368762265));
#54564=CARTESIAN_POINT('Ctrl Pts',(103.631857023051,-9.85972526564893,8.13178270264242));
#54565=CARTESIAN_POINT('Ctrl Pts',(103.773806279094,-12.5306135179784,2.51471610725899));
#54566=CARTESIAN_POINT('Ctrl Pts',(103.915755535137,-12.2337805326052,-3.69792997731523));
#54567=CARTESIAN_POINT('Ctrl Pts',(104.057704791179,-9.03952754046357,-9.03476696336253));
#54568=CARTESIAN_POINT('Ctrl Pts',(104.199654047222,-3.70437395937153,-12.2318308444042));
#54569=CARTESIAN_POINT('Ctrl Pts',(104.341603303265,2.50811489792676,-12.5319364782989));
#54570=CARTESIAN_POINT('Ctrl Pts',(104.483552559307,8.12658768099816,-9.86400754761923));
#54571=CARTESIAN_POINT('Ctrl Pts',(104.62550181535,11.8203784191338,-4.85991010891227));
#54572=CARTESIAN_POINT('Ctrl Pts',(104.767451071393,12.7146583413247,1.29519708880673));
#54573=CARTESIAN_POINT('Ctrl Pts',(104.909400327435,10.5976282800308,7.14355283287862));
#54574=CARTESIAN_POINT('Ctrl Pts',(105.051349583478,5.97068068925705,11.3000462099963));
#54575=CARTESIAN_POINT('Ctrl Pts',(105.19329883952,-0.0703489688509323,
12.7802630349062));
#54576=CARTESIAN_POINT('Ctrl Pts',(105.335248095563,-6.09471734424833,11.2336322167057));
#54577=CARTESIAN_POINT('Ctrl Pts',(105.477197351606,-10.6756270935914,7.02645417641905));
#54578=CARTESIAN_POINT('Ctrl Pts',(105.619146607648,-12.7281462692263,1.15514715408727));
#54579=CARTESIAN_POINT('Ctrl Pts',(105.761095863691,-11.7661609868312,-4.9897422498888));
#54580=CARTESIAN_POINT('Ctrl Pts',(105.903045119734,-8.01750567052013,-9.95287269618837));
#54581=CARTESIAN_POINT('Ctrl Pts',(106.044994375776,-2.37000292980183,-12.5587881405432));
#54582=CARTESIAN_POINT('Ctrl Pts',(106.186943631819,3.83880554430886,-12.1903092846983));
#54583=CARTESIAN_POINT('Ctrl Pts',(106.328892887862,9.13844074790435,-8.93470657296535));
#54584=CARTESIAN_POINT('Ctrl Pts',(106.470842143904,12.2737480144022,-3.56302773822597));
#54585=CARTESIAN_POINT('Ctrl Pts',(106.612791399947,12.5021714997374,2.65250799988186));
#54586=CARTESIAN_POINT('Ctrl Pts',(106.754740655989,9.76960565984174,8.23983465334451));
#54587=CARTESIAN_POINT('Ctrl Pts',(106.896689912032,4.72323804047272,11.8756482956073));
#54588=CARTESIAN_POINT('Ctrl Pts',(107.038639168075,-1.4417885823559,12.6988815789343));
#54589=CARTESIAN_POINT('Ctrl Pts',(107.180588424117,-7.26530717683752,10.5144988372159));
#54590=CARTESIAN_POINT('Ctrl Pts',(107.32253768016,-11.3682069144738,5.83997544773233));
#54591=CARTESIAN_POINT('Ctrl Pts',(107.464486936203,-12.7785214552891,-0.217858395306709));
#54592=CARTESIAN_POINT('Ctrl Pts',(107.606436192245,-11.1627459783923,-6.22370549662259));
#54593=CARTESIAN_POINT('Ctrl Pts',(107.748385448288,-6.90248759319296,-10.7563167196217));
#54594=CARTESIAN_POINT('Ctrl Pts',(107.84301828565,-2.97353732935054,-12.078034946598));
#54595=CARTESIAN_POINT('Ctrl Pts',(107.890334704331,-0.968368452999927,
-12.2367165887455));
#54596=CARTESIAN_POINT('Ctrl Pts',(96.446025,-5.49736112202026,11.352662011339));
#54597=CARTESIAN_POINT('Ctrl Pts',(96.4933414186809,-7.35766444471074,10.4518372399234));
#54598=CARTESIAN_POINT('Ctrl Pts',(96.5879742560426,-10.6252381356268,7.71910552931836));
#54599=CARTESIAN_POINT('Ctrl Pts',(96.7299235120854,-13.0107296874969,1.78880986789227));
#54600=CARTESIAN_POINT('Ctrl Pts',(96.8718727681279,-12.3143854371262,-4.56413381289968));
#54601=CARTESIAN_POINT('Ctrl Pts',(97.0138220241706,-8.70171578656381,-9.8366206493138));
#54602=CARTESIAN_POINT('Ctrl Pts',(97.1557712802131,-3.02806237829558,-12.7791869261708));
#54603=CARTESIAN_POINT('Ctrl Pts',(97.2977205362559,3.36270724869071,-12.6952750336362));
#54604=CARTESIAN_POINT('Ctrl Pts',(97.4396697922984,8.95708180243563,-9.60458883621892));
#54605=CARTESIAN_POINT('Ctrl Pts',(97.5816190483411,12.4300721041979,-4.23920067404235));
#54606=CARTESIAN_POINT('Ctrl Pts',(97.7235683043837,12.9591579250913,2.13020256188059));
#54607=CARTESIAN_POINT('Ctrl Pts',(97.8655175604264,10.4190247645352,7.99508750590277));
#54608=CARTESIAN_POINT('Ctrl Pts',(98.007466816469,5.41127521296109,11.966437524975));
#54609=CARTESIAN_POINT('Ctrl Pts',(98.1494160725116,-0.878068648323085,
13.103683025823));
#54610=CARTESIAN_POINT('Ctrl Pts',(98.2913653285542,-6.95945252857012,11.1374835199173));
#54611=CARTESIAN_POINT('Ctrl Pts',(98.4333145845969,-11.3925760488491,6.53350810712207));
#54612=CARTESIAN_POINT('Ctrl Pts',(98.5752638406395,-13.1275084090793,0.38215205019881));
#54613=CARTESIAN_POINT('Ctrl Pts',(98.7172130966822,-11.7533523678177,-5.85971208040458));
#54614=CARTESIAN_POINT('Ctrl Pts',(98.8591623527249,-7.59555979073004,-10.7137756526047));
#54615=CARTESIAN_POINT('Ctrl Pts',(99.0011116087674,-1.63885258030699,-13.0304136407544));
#54616=CARTESIAN_POINT('Ctrl Pts',(99.1430608648101,4.70599665045546,-12.2609588892376));
#54617=CARTESIAN_POINT('Ctrl Pts',(99.2850101208528,9.93628862488146,-8.58764727642455));
#54618=CARTESIAN_POINT('Ctrl Pts',(99.4269593768953,12.8132932104068,-2.88045733901893));
#54619=CARTESIAN_POINT('Ctrl Pts',(99.5689086329381,12.6556273597872,3.50893338572759));
#54620=CARTESIAN_POINT('Ctrl Pts',(99.7108578889806,9.50063228533051,9.06727652369311));
#54621=CARTESIAN_POINT('Ctrl Pts',(99.8528071450232,4.09552965106957,12.4781470681147));
#54622=CARTESIAN_POINT('Ctrl Pts',(99.9947564010659,-2.27954865973836,12.9337224063726));
#54623=CARTESIAN_POINT('Ctrl Pts',(100.136705657109,-8.11474399035933,10.326105139296));
#54624=CARTESIAN_POINT('Ctrl Pts',(100.278654913151,-12.0280623079928,5.27287724985078));
#54625=CARTESIAN_POINT('Ctrl Pts',(100.420604169194,-13.0926824426846,-1.02916657154219));
#54626=CARTESIAN_POINT('Ctrl Pts',(100.562553425236,-11.0564622483732,-7.08746498596154));
#54627=CARTESIAN_POINT('Ctrl Pts',(100.704502681279,-6.40165535986017,-11.4671847473793));
#54628=CARTESIAN_POINT('Ctrl Pts',(100.846451937322,-0.230695368335135,
-13.1310432572577));
#54629=CARTESIAN_POINT('Ctrl Pts',(100.988401193364,5.99490197538842,-11.6849761524118));
#54630=CARTESIAN_POINT('Ctrl Pts',(101.130350449407,10.8006807376205,-7.4714665883574));
#54631=CARTESIAN_POINT('Ctrl Pts',(101.27229970545,13.0484515012247,-1.48843232870433));
#54632=CARTESIAN_POINT('Ctrl Pts',(101.414248961492,12.2058574886926,4.84711876713115));
#54633=CARTESIAN_POINT('Ctrl Pts',(101.556198217535,8.47245669789572,10.0346895756286));
#54634=CARTESIAN_POINT('Ctrl Pts',(101.698147473577,2.73245905198082,12.8456679431704));
#54635=CARTESIAN_POINT('Ctrl Pts',(101.84009672962,-3.6546878135702,12.6143083188215));
#54636=CARTESIAN_POINT('Ctrl Pts',(101.982045985663,-9.17626695365029,9.39540537562336));
#54637=CARTESIAN_POINT('Ctrl Pts',(102.123995241705,-12.5245604615368,3.95131656821565));
#54638=CARTESIAN_POINT('Ctrl Pts',(102.265944497748,-12.9065663234684,-2.42859282607413));
#54639=CARTESIAN_POINT('Ctrl Pts',(102.407893753791,-10.2318111633605,-8.23331996792782));
#54640=CARTESIAN_POINT('Ctrl Pts',(102.549843009833,-5.13377774587759,-12.0880868392347));
#54641=CARTESIAN_POINT('Ctrl Pts',(102.691792265876,1.18012760191706,-13.0799394578163));
#54642=CARTESIAN_POINT('Ctrl Pts',(102.833741521919,7.21453428491085,-10.9739697661691));
#54643=CARTESIAN_POINT('Ctrl Pts',(102.975690777961,11.5402675189345,-6.26895070712579));
#54644=CARTESIAN_POINT('Ctrl Pts',(103.117640034004,13.1328307485051,-0.0792080050648763));
#54645=CARTESIAN_POINT('Ctrl Pts',(103.259589290047,11.6150450180989,6.12929413590858));
#54646=CARTESIAN_POINT('Ctrl Pts',(103.401538546089,7.34637915499623,10.886148569994));
#54647=CARTESIAN_POINT('Ctrl Pts',(103.543487802132,1.33781401184385,13.0647530036607));
#54648=CARTESIAN_POINT('Ctrl Pts',(103.685437058174,-4.98759587712636,12.1491318514294));
#54649=CARTESIAN_POINT('Ctrl Pts',(103.827386314217,-10.1317552081416,8.35613868836854));
#54650=CARTESIAN_POINT('Ctrl Pts',(103.96933557026,-12.8763333005133,2.58409715587975));
#54651=CARTESIAN_POINT('Ctrl Pts',(104.111284826302,-12.5713106893884,-3.79995591130102));
#54652=CARTESIAN_POINT('Ctrl Pts',(104.253234082345,-9.28892821753527,-9.28403629605289));
#54653=CARTESIAN_POINT('Ctrl Pts',(104.395183338388,-3.80657768290228,-12.5693072092657));
#54654=CARTESIAN_POINT('Ctrl Pts',(104.53713259443,2.57731381910005,-12.8776927613255));
#54655=CARTESIAN_POINT('Ctrl Pts',(104.679081850473,8.35080033601259,-10.1361556383247));
#54656=CARTESIAN_POINT('Ctrl Pts',(104.821031106516,12.1465028064736,-4.99399508915542));
#54657=CARTESIAN_POINT('Ctrl Pts',(104.962980362558,13.0654559228208,1.33093159256742));
#54658=CARTESIAN_POINT('Ctrl Pts',(105.104929618601,10.8900169758518,7.34064354422855));
#54659=CARTESIAN_POINT('Ctrl Pts',(105.246878874643,6.13541184360268,11.6118146252259));
#54660=CARTESIAN_POINT('Ctrl Pts',(105.388828130686,-0.0722898977749296,
13.1328706507127));
#54661=CARTESIAN_POINT('Ctrl Pts',(105.530777386729,-6.26287067144513,11.5435682690358));
#54662=CARTESIAN_POINT('Ctrl Pts',(105.672726642771,-10.9701677776469,7.22031413438345));
#54663=CARTESIAN_POINT('Ctrl Pts',(105.814675898814,-13.0793159828206,1.18701767841028));
#54664=CARTESIAN_POINT('Ctrl Pts',(105.956625154857,-12.0907895145407,-5.12740930051339));
#54665=CARTESIAN_POINT('Ctrl Pts',(106.098574410899,-8.23870875151118,-10.2274725774461));
#54666=CARTESIAN_POINT('Ctrl Pts',(106.240523666942,-2.43539134005986,-12.9052852612645));
#54667=CARTESIAN_POINT('Ctrl Pts',(106.382472922984,3.94471823693704,-12.526640069212));
#54668=CARTESIAN_POINT('Ctrl Pts',(106.524422179027,9.39057044159739,-9.18121523824236));
#54669=CARTESIAN_POINT('Ctrl Pts',(106.66637143507,12.6123808745043,-3.66133171776043));
#54670=CARTESIAN_POINT('Ctrl Pts',(106.808320691112,12.8471065666359,2.72569072853082));
#54671=CARTESIAN_POINT('Ctrl Pts',(106.950269947155,10.0391492012914,8.46717179373198));
#54672=CARTESIAN_POINT('Ctrl Pts',(107.092219203198,4.85355223665076,12.2032975795253));
#54673=CARTESIAN_POINT('Ctrl Pts',(107.23416845924,-1.48156754724362,13.0492438793601));
#54674=CARTESIAN_POINT('Ctrl Pts',(107.376117715283,-7.46575709204891,10.8045939906775));
#54675=CARTESIAN_POINT('Ctrl Pts',(107.518066971325,-11.6818558843861,6.00110044284153));
#54676=CARTESIAN_POINT('Ctrl Pts',(107.660016227368,-13.1310810208923,-0.223869111138029));
#54677=CARTESIAN_POINT('Ctrl Pts',(107.801965483411,-11.4707262785273,-6.39541760854485));
#54678=CARTESIAN_POINT('Ctrl Pts',(107.943914739453,-7.09292731158704,-11.0530836314612));
#54679=CARTESIAN_POINT('Ctrl Pts',(108.038547576815,-3.05557726118531,-12.4112680807296));
#54680=CARTESIAN_POINT('Ctrl Pts',(108.085863995496,-0.995085750640993,
-12.574327751354));
#54681=CARTESIAN_POINT('',(97.1841636168587,-1.68935314531928,-12.5));
#54682=CARTESIAN_POINT('',(97.2617423708143,1.68935314531928,-12.5));
#54683=CARTESIAN_POINT('Ctrl Pts',(97.1841636168587,-1.68966879435806,-12.5001504794836));
#54684=CARTESIAN_POINT('Ctrl Pts',(97.1836617116955,-1.68048229176406,-12.500141503016));
#54685=CARTESIAN_POINT('Ctrl Pts',(97.1831655403902,-1.67129546732837,-12.500132520818));
#54686=CARTESIAN_POINT('Ctrl Pts',(97.182675107321,-1.66210830628068,-12.5001235359673));
#54687=CARTESIAN_POINT('Ctrl Pts',(97.1694300033715,-1.41399105901218,-12.4998808825057));
#54688=CARTESIAN_POINT('Ctrl Pts',(97.1603881541905,-1.16596021025893,-12.499638689875));
#54689=CARTESIAN_POINT('Ctrl Pts',(97.1556009301936,-0.917715246001572,
-12.4994457080315));
#54690=CARTESIAN_POINT('Ctrl Pts',(97.1535063791998,-0.809100788663271,
-12.4993612728113));
#54691=CARTESIAN_POINT('Ctrl Pts',(97.1522262993178,-0.700444678977253,
-12.4992860395109));
#54692=CARTESIAN_POINT('Ctrl Pts',(97.1517649931838,-0.591718942494721,
-12.4992227758313));
#54693=CARTESIAN_POINT('Ctrl Pts',(97.151012012177,-0.41424804301112,-12.4991195117606));
#54694=CARTESIAN_POINT('Ctrl Pts',(97.15244156732,-0.236852374547013,-12.4990485185025));
#54695=CARTESIAN_POINT('Ctrl Pts',(97.1560531749278,-0.0594127045311677,
-12.4990160668234));
#54696=CARTESIAN_POINT('Ctrl Pts',(97.1563224737121,-0.0461819517430822,
-12.4990136470706));
#54697=CARTESIAN_POINT('Ctrl Pts',(97.1566038939014,-0.0329514754057439,
-12.4990114386038));
#54698=CARTESIAN_POINT('Ctrl Pts',(97.1568974324251,-0.0197212262430592,
-12.4990094424722));
#54699=CARTESIAN_POINT('Ctrl Pts',(97.1569780844716,-0.0160861099501589,
-12.4990088940192));
#54700=CARTESIAN_POINT('Ctrl Pts',(97.1570596512777,-0.0124510142730335,
-12.499008361595));
#54701=CARTESIAN_POINT('Ctrl Pts',(97.1571421327746,-0.00881593818621189,
-12.4990078452187));
#54702=CARTESIAN_POINT('Ctrl Pts',(97.1571905860349,-0.00668053455459407,
-12.4990075418765));
#54703=CARTESIAN_POINT('Ctrl Pts',(97.157239354937,-0.00454513809380544,
-12.4990072440723));
#54704=CARTESIAN_POINT('Ctrl Pts',(97.1572884394683,-0.00240974851892736,
-12.4990069518098));
#54705=CARTESIAN_POINT('Ctrl Pts',(97.1573308177058,-0.000566111752699424,
-12.4990066994783));
#54706=CARTESIAN_POINT('Ctrl Pts',(97.157373431211,0.00127751961241762,
-12.4990064512776));
#54707=CARTESIAN_POINT('Ctrl Pts',(97.1574162799744,0.00312114570776404,
-12.4990062072099));
#54708=CARTESIAN_POINT('Ctrl Pts',(97.1574684636542,0.00536641922499062,
-12.4990059099704));
#54709=CARTESIAN_POINT('Ctrl Pts',(97.1575209962562,0.00761168460872278,
-12.499005618861));
#54710=CARTESIAN_POINT('Ctrl Pts',(97.1575738777611,0.00985694202133178,
-12.4990053338855));
#54711=CARTESIAN_POINT('Ctrl Pts',(97.1576736462671,0.014092940556016,-12.4990047962387));
#54712=CARTESIAN_POINT('Ctrl Pts',(97.1577746566296,0.0183289091899971,
-12.4990042804258));
#54713=CARTESIAN_POINT('Ctrl Pts',(97.1578769087305,0.0225648495757296,
-12.4990037864712));
#54714=CARTESIAN_POINT('Ctrl Pts',(97.1584593407123,0.0466929323328523,
-12.4990009728865));
#54715=CARTESIAN_POINT('Ctrl Pts',(97.1590820545152,0.0708198412374658,
-12.4989988687095));
#54716=CARTESIAN_POINT('Ctrl Pts',(97.1597450255452,0.0949458742036956,
-12.4989974770508));
#54717=CARTESIAN_POINT('Ctrl Pts',(97.1605926787677,0.125792636228222,-12.4989956977212));
#54718=CARTESIAN_POINT('Ctrl Pts',(97.1615061196423,0.15663715691193,-12.4989950834167));
#54719=CARTESIAN_POINT('Ctrl Pts',(97.1624852863278,0.187480056498351,-12.498995634938));
#54720=CARTESIAN_POINT('Ctrl Pts',(97.1673070823745,0.339362441268142,-12.4989983508425));
#54721=CARTESIAN_POINT('Ctrl Pts',(97.1737206661987,0.491141315565022,-12.4990296235006));
#54722=CARTESIAN_POINT('Ctrl Pts',(97.181714540668,0.642889198400638,-12.49908730495));
#54723=CARTESIAN_POINT('Ctrl Pts',(97.1943805598043,0.883328499177757,-12.4991786992227));
#54724=CARTESIAN_POINT('Ctrl Pts',(97.210992279406,1.12327169768875,-12.4993379199478));
#54725=CARTESIAN_POINT('Ctrl Pts',(97.231460625774,1.36298827907735,-12.4995363845337));
#54726=CARTESIAN_POINT('Ctrl Pts',(97.2407610752496,1.47191119417622,-12.4996265632819));
#54727=CARTESIAN_POINT('Ctrl Pts',(97.25085777569,1.58078667024217,-12.4997246141786));
#54728=CARTESIAN_POINT('Ctrl Pts',(97.2617423708143,1.68963646449083,-12.4998270697762));
#54729=CARTESIAN_POINT('',(96.446025,-5.49736112202046,11.3526620113389));
#54730=CARTESIAN_POINT('Ctrl Pts',(96.446025,-5.4973611220203,11.352662011339));
#54731=CARTESIAN_POINT('Ctrl Pts',(96.4933414186809,-7.35766444471076,10.4518372399233));
#54732=CARTESIAN_POINT('Ctrl Pts',(96.5406578373617,-8.9914512901688,9.08547138462084));
#54733=CARTESIAN_POINT('Ctrl Pts',(96.5879742560426,-10.2059266382095,7.41390584673193));
#54734=CARTESIAN_POINT('Ctrl Pts',(96.6352906747235,-11.4204019862502,5.742340308843));
#54735=CARTESIAN_POINT('Ctrl Pts',(96.6826070934045,-12.2155658368735,3.76557508836764));
#54736=CARTESIAN_POINT('Ctrl Pts',(96.7299235120853,-12.4970903871234,1.7183685313313));
#54737=CARTESIAN_POINT('Ctrl Pts',(96.7772399307662,-12.7786149373733,-0.328838025705044));
#54738=CARTESIAN_POINT('Ctrl Pts',(96.824556349447,-12.5465001872497,-2.44648591930237));
#54739=CARTESIAN_POINT('Ctrl Pts',(96.8718727681279,-11.8283312037609,-4.38405767217005));
#54740=CARTESIAN_POINT('Ctrl Pts',(96.9191891868088,-11.110162220272,-6.32162942503772));
#54741=CARTESIAN_POINT('Ctrl Pts',(96.9665056054897,-9.90593900341793,-8.07912503717576));
#54742=CARTESIAN_POINT('Ctrl Pts',(97.0138220241706,-8.35821849361283,-9.44830055605428));
#54743=CARTESIAN_POINT('Ctrl Pts',(97.0611384428514,-6.81049798380774,-10.8174760749328));
#54744=CARTESIAN_POINT('Ctrl Pts',(97.1084548615323,-4.91928018105167,-11.7983315005518));
#54745=CARTESIAN_POINT('Ctrl Pts',(97.1557712802132,-2.90854300850926,-12.2747738979388));
#54746=CARTESIAN_POINT('Ctrl Pts',(97.1652353924284,-2.50636036733103,-12.3700707196056));
#54747=CARTESIAN_POINT('Ctrl Pts',(97.1746995046436,-2.09939611424284,-12.4451874872138));
#54748=CARTESIAN_POINT('Ctrl Pts',(97.1841636168587,-1.68966879435857,-12.5001504794835));
#54749=CARTESIAN_POINT('',(96.446025,-7.10320028565243,-9.16786776036321));
#54750=CARTESIAN_POINT('Ctrl Pts',(96.446025,-7.10371691227606,-9.16818944635625));
#54751=CARTESIAN_POINT('Ctrl Pts',(96.446025,-7.30978227149857,-9.02256097481596));
#54752=CARTESIAN_POINT('Ctrl Pts',(96.446025,-7.51084480534185,-8.8703120063485));
#54753=CARTESIAN_POINT('Ctrl Pts',(96.446025,-7.70654954542632,-8.71164069364237));
#54754=CARTESIAN_POINT('Ctrl Pts',(96.446025,-7.92191546555672,-8.53702870803333));
#54755=CARTESIAN_POINT('Ctrl Pts',(96.446025,-8.13079395813826,-8.35463972061946));
#54756=CARTESIAN_POINT('Ctrl Pts',(96.446025,-8.33291957884125,-8.16495486798257));
#54757=CARTESIAN_POINT('Ctrl Pts',(96.446025,-8.4832417260981,-8.02388500137534));
#54758=CARTESIAN_POINT('Ctrl Pts',(96.446025,-8.62982836664002,-7.87877876499321));
#54759=CARTESIAN_POINT('Ctrl Pts',(96.446025,-8.77255919267182,-7.72981909737944));
#54760=CARTESIAN_POINT('Ctrl Pts',(96.446025,-8.84563001113479,-7.65355943341528));
#54761=CARTESIAN_POINT('Ctrl Pts',(96.446025,-8.91769009145714,-7.57628962582517));
#54762=CARTESIAN_POINT('Ctrl Pts',(96.446025,-8.98872220008187,-7.49803307925646));
#54763=CARTESIAN_POINT('Ctrl Pts',(96.446025,-9.03428838540755,-7.44783250978251));
#54764=CARTESIAN_POINT('Ctrl Pts',(96.446025,-9.07943153913389,-7.39722587640377));
#54765=CARTESIAN_POINT('Ctrl Pts',(96.446025,-9.12414693982324,-7.34621920411752));
#54766=CARTESIAN_POINT('Ctrl Pts',(96.446025,-9.15309102287457,-7.31320280851185));
#54767=CARTESIAN_POINT('Ctrl Pts',(96.446025,-9.18185686627777,-7.28001755106976));
#54768=CARTESIAN_POINT('Ctrl Pts',(96.446025,-9.21042952422747,-7.24668122873893));
#54769=CARTESIAN_POINT('Ctrl Pts',(96.446025,-9.39281579291678,-7.03388732442495));
#54770=CARTESIAN_POINT('Ctrl Pts',(96.446025,-9.56746197962767,-6.81479614168976));
#54771=CARTESIAN_POINT('Ctrl Pts',(96.446025,-9.73409922463371,-6.58989399404312));
#54772=CARTESIAN_POINT('Ctrl Pts',(96.446025,-9.90183700371478,-6.36350650932778));
#54773=CARTESIAN_POINT('Ctrl Pts',(96.446025,-10.0614601394372,-6.13123059900815));
#54774=CARTESIAN_POINT('Ctrl Pts',(96.446025,-10.2126589253177,-5.89352356979185));
#54775=CARTESIAN_POINT('Ctrl Pts',(96.446025,-10.3633936752713,-5.65654607422211));
#54776=CARTESIAN_POINT('Ctrl Pts',(96.446025,-10.5057560910357,-5.41417023874808));
#54777=CARTESIAN_POINT('Ctrl Pts',(96.446025,-10.6393980847918,-5.1668181108504));
#54778=CARTESIAN_POINT('Ctrl Pts',(96.446025,-10.6627641550139,-5.12357087225718));
#54779=CARTESIAN_POINT('Ctrl Pts',(96.446025,-10.6858635375631,-5.08017144590901));
#54780=CARTESIAN_POINT('Ctrl Pts',(96.446025,-10.7086942282531,-5.0366220075035));
#54781=CARTESIAN_POINT('Ctrl Pts',(96.446025,-10.727478568401,-5.00079096430983));
#54782=CARTESIAN_POINT('Ctrl Pts',(96.446025,-10.7460821600203,-4.96485601687245));
#54783=CARTESIAN_POINT('Ctrl Pts',(96.446025,-10.7644932211042,-4.92883954535707));
#54784=CARTESIAN_POINT('Ctrl Pts',(96.446025,-10.8987630685253,-4.66617537228287));
#54785=CARTESIAN_POINT('Ctrl Pts',(96.446025,-11.0229197835297,-4.39894687519522));
#54786=CARTESIAN_POINT('Ctrl Pts',(96.446025,-11.1366626238853,-4.12769733765066));
#54787=CARTESIAN_POINT('Ctrl Pts',(96.446025,-11.2450445015555,-3.86923241709514));
#54788=CARTESIAN_POINT('Ctrl Pts',(96.446025,-11.3439714533202,-3.60711590739578));
#54789=CARTESIAN_POINT('Ctrl Pts',(96.446025,-11.4334649925142,-3.34190306363835));
#54790=CARTESIAN_POINT('Ctrl Pts',(96.446025,-11.5238417961909,-3.0740726780187));
#54791=CARTESIAN_POINT('Ctrl Pts',(96.446025,-11.6045982489161,-2.80308398612925));
#54792=CARTESIAN_POINT('Ctrl Pts',(96.446025,-11.6757096849509,-2.52948279890396));
#54793=CARTESIAN_POINT('Ctrl Pts',(96.446025,-11.7471005597629,-2.25480647123063));
#54794=CARTESIAN_POINT('Ctrl Pts',(96.446025,-11.8087706245828,-1.97749647593278));
#54795=CARTESIAN_POINT('Ctrl Pts',(96.446025,-11.8606454191839,-1.69808769268104));
#54796=CARTESIAN_POINT('Ctrl Pts',(96.446025,-11.9117669507853,-1.42273614570025));
#54797=CARTESIAN_POINT('Ctrl Pts',(96.446025,-11.9533756270982,-1.1453457118012));
#54798=CARTESIAN_POINT('Ctrl Pts',(96.446025,-11.985351194423,-0.866420498375038));
#54799=CARTESIAN_POINT('Ctrl Pts',(96.446025,-11.9963079527002,-0.770843894217156));
#54800=CARTESIAN_POINT('Ctrl Pts',(96.446025,-12.0061332000131,-0.675087055171968));
#54801=CARTESIAN_POINT('Ctrl Pts',(96.446025,-12.0148207414527,-0.579170243646206));
#54802=CARTESIAN_POINT('Ctrl Pts',(96.446025,-12.0171896950221,-0.553015263596951));
#54803=CARTESIAN_POINT('Ctrl Pts',(96.446025,-12.0194738907792,-0.526849902756527));
#54804=CARTESIAN_POINT('Ctrl Pts',(96.446025,-12.0216724868579,-0.500684083298083));
#54805=CARTESIAN_POINT('Ctrl Pts',(96.446025,-12.0456996720184,-0.214732973353064));
#54806=CARTESIAN_POINT('Ctrl Pts',(96.446025,-12.0595364563262,0.071584871261912));
#54807=CARTESIAN_POINT('Ctrl Pts',(96.446025,-12.0631927104438,0.357708958361966));
#54808=CARTESIAN_POINT('Ctrl Pts',(96.446025,-12.0668701045469,0.645487377699364));
#54809=CARTESIAN_POINT('Ctrl Pts',(96.446025,-12.0602490557768,0.933070404419091));
#54810=CARTESIAN_POINT('Ctrl Pts',(96.446025,-12.0432896813139,1.21990410757687));
#54811=CARTESIAN_POINT('Ctrl Pts',(96.446025,-12.0347733144521,1.36394132131739));
#54812=CARTESIAN_POINT('Ctrl Pts',(96.446025,-12.0236491615489,1.50778977852785));
#54813=CARTESIAN_POINT('Ctrl Pts',(96.446025,-12.0099072778166,1.65138012858342));
#54814=CARTESIAN_POINT('Ctrl Pts',(96.446025,-11.9826587599829,1.93610268121525));
#54815=CARTESIAN_POINT('Ctrl Pts',(96.446025,-11.9451211361171,2.21981062774033));
#54816=CARTESIAN_POINT('Ctrl Pts',(96.446025,-11.8975263909157,2.50200891361867));
#54817=CARTESIAN_POINT('Ctrl Pts',(96.446025,-11.8497672155975,2.78518213689705));
#54818=CARTESIAN_POINT('Ctrl Pts',(96.446025,-11.7918811654255,3.06683584840972));
#54819=CARTESIAN_POINT('Ctrl Pts',(96.446025,-11.724050534956,3.34646281732963));
#54820=CARTESIAN_POINT('Ctrl Pts',(96.446025,-11.6817572389484,3.52081393402108));
#54821=CARTESIAN_POINT('Ctrl Pts',(96.446025,-11.6355967773695,3.69437694499245));
#54822=CARTESIAN_POINT('Ctrl Pts',(96.446025,-11.5856035149477,3.86702593820762));
#54823=CARTESIAN_POINT('Ctrl Pts',(96.446025,-11.570956641705,3.9176081126169));
#54824=CARTESIAN_POINT('Ctrl Pts',(96.446025,-11.5559807299102,3.9681118128852));
#54825=CARTESIAN_POINT('Ctrl Pts',(96.446025,-11.5406765247744,4.018533822066));
#54826=CARTESIAN_POINT('Ctrl Pts',(96.446025,-11.5313993558877,4.0490988524368));
#54827=CARTESIAN_POINT('Ctrl Pts',(96.446025,-11.5220010034243,4.07963561824385));
#54828=CARTESIAN_POINT('Ctrl Pts',(96.446025,-11.5124833492986,4.11013787574345));
#54829=CARTESIAN_POINT('Ctrl Pts',(96.446025,-11.4250037595175,4.39049319631259));
#54830=CARTESIAN_POINT('Ctrl Pts',(96.446025,-11.3276603568015,4.66726394819521));
#54831=CARTESIAN_POINT('Ctrl Pts',(96.446025,-11.2207605924677,4.93993847505352));
#54832=CARTESIAN_POINT('Ctrl Pts',(96.446025,-11.1145410184204,5.21087800683767));
#54833=CARTESIAN_POINT('Ctrl Pts',(96.446025,-10.998886044537,5.47777387765371));
#54834=CARTESIAN_POINT('Ctrl Pts',(96.446025,-10.8740437695655,5.74012050388206));
#54835=CARTESIAN_POINT('Ctrl Pts',(96.446025,-10.7480023299831,6.00498708410843));
#54836=CARTESIAN_POINT('Ctrl Pts',(96.446025,-10.6125961267233,6.26521724850586));
#54837=CARTESIAN_POINT('Ctrl Pts',(96.446025,-10.4680284180515,6.52027759435502));
#54838=CARTESIAN_POINT('Ctrl Pts',(96.446025,-10.3234607093797,6.77533794020419));
#54839=CARTESIAN_POINT('Ctrl Pts',(96.446025,-10.1697312994683,7.02522910650024));
#54840=CARTESIAN_POINT('Ctrl Pts',(96.446025,-10.0069941299641,7.26939502098643));
#54841=CARTESIAN_POINT('Ctrl Pts',(96.446025,-9.86517940602884,7.48216953256695));
#54842=CARTESIAN_POINT('Ctrl Pts',(96.446025,-9.71652325830122,7.69059612443967));
#54843=CARTESIAN_POINT('Ctrl Pts',(96.446025,-9.56129306948992,7.89443387712908));
#54844=CARTESIAN_POINT('Ctrl Pts',(96.446025,-9.49337986188497,7.9836128939307));
#54845=CARTESIAN_POINT('Ctrl Pts',(96.446025,-9.42420802625417,8.0719133244014));
#54846=CARTESIAN_POINT('Ctrl Pts',(96.446025,-9.3537985551078,8.15931373120115));
#54847=CARTESIAN_POINT('Ctrl Pts',(96.446025,-9.32159971279966,8.19928267103827));
#54848=CARTESIAN_POINT('Ctrl Pts',(96.446025,-9.28914203146188,8.23906337680869));
#54849=CARTESIAN_POINT('Ctrl Pts',(96.446025,-9.25642746403099,8.27865373987974));
#54850=CARTESIAN_POINT('Ctrl Pts',(96.446025,-9.2389484729194,8.29980638405533));
#54851=CARTESIAN_POINT('Ctrl Pts',(96.446025,-9.22139800546104,8.32090241663264));
#54852=CARTESIAN_POINT('Ctrl Pts',(96.446025,-9.20378185908125,8.34193511893918));
#54853=CARTESIAN_POINT('Ctrl Pts',(96.446025,-9.017527891134,8.56431203252688));
#54854=CARTESIAN_POINT('Ctrl Pts',(96.446025,-8.82376074067442,8.77982359138969));
#54855=CARTESIAN_POINT('Ctrl Pts',(96.446025,-8.62297236676072,8.98819473876588));
#54856=CARTESIAN_POINT('Ctrl Pts',(96.446025,-8.41981989343368,9.19901926577589));
#54857=CARTESIAN_POINT('Ctrl Pts',(96.446025,-8.20947954225884,9.40253470020656));
#54858=CARTESIAN_POINT('Ctrl Pts',(96.446025,-7.99241348006684,9.59843173573151));
#54859=CARTESIAN_POINT('Ctrl Pts',(96.446025,-7.77381751752192,9.7957094704812));
#54860=CARTESIAN_POINT('Ctrl Pts',(96.446025,-7.54840030538829,9.985261502155));
#54861=CARTESIAN_POINT('Ctrl Pts',(96.446025,-7.31659176195654,10.1667404004619));
#54862=CARTESIAN_POINT('Ctrl Pts',(96.446025,-7.0853784788602,10.3477532797503));
#54863=CARTESIAN_POINT('Ctrl Pts',(96.446025,-6.84780618879341,10.5207348556717));
#54864=CARTESIAN_POINT('Ctrl Pts',(96.446025,-6.60426630301782,10.6853025304088));
#54865=CARTESIAN_POINT('Ctrl Pts',(96.446025,-6.36375524498132,10.8478235295608));
#54866=CARTESIAN_POINT('Ctrl Pts',(96.446025,-6.11742362339088,11.0021389485234));
#54867=CARTESIAN_POINT('Ctrl Pts',(96.446025,-5.86562108206444,11.1478377897083));
#54868=CARTESIAN_POINT('Ctrl Pts',(96.446025,-5.74412924799045,11.218135807134));
#54869=CARTESIAN_POINT('Ctrl Pts',(96.446025,-5.62136344491582,11.2864272585636));
#54870=CARTESIAN_POINT('Ctrl Pts',(96.446025,-5.49736112202026,11.352662011339));
#54871=CARTESIAN_POINT('Ctrl Pts',(96.446025,-7.10371691227614,-9.16818944635619));
#54872=CARTESIAN_POINT('Ctrl Pts',(96.4870778022389,-5.79962471393883,-10.1767945155287));
#54873=CARTESIAN_POINT('Ctrl Pts',(96.5754470231585,-2.52487563733554,-11.7464480653471));
#54874=CARTESIAN_POINT('Ctrl Pts',(96.7111326627592,3.091848831559,-11.6726995174351));
#54875=CARTESIAN_POINT('Ctrl Pts',(96.8530819188018,8.23560924484923,-8.83096106044612));
#54876=CARTESIAN_POINT('Ctrl Pts',(96.9950311748445,11.4288580805009,-3.8977427059358));
#54877=CARTESIAN_POINT('Ctrl Pts',(97.136980430887,11.915327242442,1.95861959274003));
#54878=CARTESIAN_POINT('Ctrl Pts',(97.2789296869297,9.5797960279637,7.35110139990983));
#54879=CARTESIAN_POINT('Ctrl Pts',(97.4208789429723,4.97540930776886,11.0025682116464));
#54880=CARTESIAN_POINT('Ctrl Pts',(97.562828199015,-0.807342216722395,12.0482111751727));
#54881=CARTESIAN_POINT('Ctrl Pts',(97.7047774550576,-6.39888446344168,10.2403845654334));
#54882=CARTESIAN_POINT('Ctrl Pts',(97.8467267111003,-10.474929971616,6.00724889591607));
#54883=CARTESIAN_POINT('Ctrl Pts',(97.9441606947658,-11.569866836913,2.12505344398514));
#54884=CARTESIAN_POINT('Ctrl Pts',(97.9942782597504,-11.5985505397983,0.112590341614262));
#54885=CARTESIAN_POINT('Ctrl Pts',(97.9970794060541,-11.5984942842416,0.000109136483176196));
#54886=CARTESIAN_POINT('',(108.068877059804,-1.6708941109609,-12.5));
#54887=CARTESIAN_POINT('Ctrl Pts',(108.068877059804,-1.67089411096091,-12.5));
#54888=CARTESIAN_POINT('Ctrl Pts',(108.030091668611,-1.63767437386533,-12.4356882468672));
#54889=CARTESIAN_POINT('Ctrl Pts',(107.991648922957,-1.60240740323059,-12.3720777992513));
#54890=CARTESIAN_POINT('Ctrl Pts',(107.763118153063,-1.3766207604813,-11.9946044607362));
#54891=CARTESIAN_POINT('Ctrl Pts',(107.609518024559,-1.15600440609235,-11.743732333501));
#54892=CARTESIAN_POINT('Ctrl Pts',(107.499276121999,-0.914933857717767,
-11.5614942635284));
#54893=CARTESIAN_POINT('',(108.069877902573,-1.6893531453193,-12.5));
#54894=CARTESIAN_POINT('Ctrl Pts',(108.069877902573,-1.6893024527008,-12.4997161179536));
#54895=CARTESIAN_POINT('Ctrl Pts',(108.069541715314,-1.68315033687534,-12.4997204364986));
#54896=CARTESIAN_POINT('Ctrl Pts',(108.069208100619,-1.67699808055201,-12.4997247234326));
#54897=CARTESIAN_POINT('Ctrl Pts',(108.068877059804,-1.67084567891917,-12.499728977557));
#54898=CARTESIAN_POINT('',(106.333170942243,1.68935314531927,-12.5));
#54899=CARTESIAN_POINT('Ctrl Pts',(106.333170942243,1.68950627976338,-12.4993304720331));
#54900=CARTESIAN_POINT('Ctrl Pts',(106.349604935823,2.40108951933161,-12.4036781514243));
#54901=CARTESIAN_POINT('Ctrl Pts',(106.366038929404,3.104440874311,-12.2477515181746));
#54902=CARTESIAN_POINT('Ctrl Pts',(106.382472922984,3.78900867488091,-12.0321767960591));
#54903=CARTESIAN_POINT('Ctrl Pts',(106.429789341665,5.76000230515714,-11.4114984588888));
#54904=CARTESIAN_POINT('Ctrl Pts',(106.477105760346,7.57528637337726,-10.2963568485656));
#54905=CARTESIAN_POINT('Ctrl Pts',(106.524422179027,9.01989681297181,-8.81880545665698));
#54906=CARTESIAN_POINT('Ctrl Pts',(106.571738597708,10.4645072525664,-7.34125406474839));
#54907=CARTESIAN_POINT('Ctrl Pts',(106.619055016389,11.5384440635353,-5.50129289125441));
#54908=CARTESIAN_POINT('Ctrl Pts',(106.66637143507,12.1145334177084,-3.51680856345888));
#54909=CARTESIAN_POINT('Ctrl Pts',(106.713687853751,12.6906227718815,-1.53232423566335));
#54910=CARTESIAN_POINT('Ctrl Pts',(106.761004272431,12.7688646692587,0.596683246433734));
#54911=CARTESIAN_POINT('Ctrl Pts',(106.808320691112,12.3399927237232,2.61810049834914));
#54912=CARTESIAN_POINT('Ctrl Pts',(106.855637109793,11.9111207781878,4.63951775026454));
#54913=CARTESIAN_POINT('Ctrl Pts',(106.902953528474,10.9751349897396,6.55334477199826));
#54914=CARTESIAN_POINT('Ctrl Pts',(106.950269947155,9.64287593474204,8.13294591383067));
#54915=CARTESIAN_POINT('Ctrl Pts',(106.997586365836,8.31061687974451,9.71254705566307));
#54916=CARTESIAN_POINT('Ctrl Pts',(107.044902784517,6.58208455819763,10.9579223175942));
#54917=CARTESIAN_POINT('Ctrl Pts',(107.092219203198,4.66196510010847,11.7216009985322));
#54918=CARTESIAN_POINT('Ctrl Pts',(107.139535621879,2.7418456420193,12.4852796794702));
#54919=CARTESIAN_POINT('Ctrl Pts',(107.186852040559,0.630139047387844,12.7672617794151));
#54920=CARTESIAN_POINT('Ctrl Pts',(107.23416845924,-1.4230791740621,12.5341445146072));
#54921=CARTESIAN_POINT('Ctrl Pts',(107.281484877921,-3.47629739551205,12.3010272497992));
#54922=CARTESIAN_POINT('Ctrl Pts',(107.328801296602,-5.47102724378048,11.5528106202384));
#54923=CARTESIAN_POINT('Ctrl Pts',(107.376117715283,-7.17107529997091,10.3781200474853));
#54924=CARTESIAN_POINT('Ctrl Pts',(107.423434133964,-8.87112335616133,9.2034294747322));
#54925=CARTESIAN_POINT('Ctrl Pts',(107.470750552645,-10.2764896202737,7.60226495878686));
#54926=CARTESIAN_POINT('Ctrl Pts',(107.518066971325,-11.220710275081,5.76418777515091));
#54927=CARTESIAN_POINT('Ctrl Pts',(107.565383390006,-12.1649309298882,3.92611059151499));
#54928=CARTESIAN_POINT('Ctrl Pts',(107.612699808687,-12.6480059753902,1.85112074018848));
#54929=CARTESIAN_POINT('Ctrl Pts',(107.660016227368,-12.6128177077471,-0.214965601709239));
#54930=CARTESIAN_POINT('Ctrl Pts',(107.707332646049,-12.5776294401039,-2.28105194360693));
#54931=CARTESIAN_POINT('Ctrl Pts',(107.75464906473,-12.0241778593156,-4.33823477607583));
#54932=CARTESIAN_POINT('Ctrl Pts',(107.801965483411,-11.0178189077648,-6.14310386279632));
#54933=CARTESIAN_POINT('Ctrl Pts',(107.849281902092,-10.0114599562139,-7.94797294951689));
#54934=CARTESIAN_POINT('Ctrl Pts',(107.896598320773,-8.55219363390049,-9.50052829048904));
#54935=CARTESIAN_POINT('Ctrl Pts',(107.943914739453,-6.81322296014332,-10.6163520732922));
#54936=CARTESIAN_POINT('Ctrl Pts',(107.985902460493,-5.27009231793075,-11.6065136076629));
#54937=CARTESIAN_POINT('Ctrl Pts',(108.027890181533,-3.50670955580399,-12.2527725498014));
#54938=CARTESIAN_POINT('Ctrl Pts',(108.069877902573,-1.68930245270044,-12.4997161179536));
#54939=CARTESIAN_POINT('',(106.255592188287,-1.6893531453193,-12.5));
#54940=CARTESIAN_POINT('Ctrl Pts',(106.255592188287,-1.68964924171336,-12.5007055298766));
#54941=CARTESIAN_POINT('Ctrl Pts',(106.255090283124,-1.68046412560261,-12.5006983493389));
#54942=CARTESIAN_POINT('Ctrl Pts',(106.254594111819,-1.67127868122275,-12.5006910846807));
#54943=CARTESIAN_POINT('Ctrl Pts',(106.25410367875,-1.66209289375809,-12.5006837399));
#54944=CARTESIAN_POINT('Ctrl Pts',(106.24084152639,-1.41369342681394,-12.5004851244185));
#54945=CARTESIAN_POINT('Ctrl Pts',(106.231793456185,-1.16537581297815,-12.5002301926239));
#54946=CARTESIAN_POINT('Ctrl Pts',(106.22701103717,-0.916837633820512,-12.4999869955818));
#54947=CARTESIAN_POINT('Ctrl Pts',(106.224927426093,-0.80855416859948,-12.4998810391508));
#54948=CARTESIAN_POINT('Ctrl Pts',(106.223653513649,-0.700228172921927,
-12.4997771026051));
#54949=CARTESIAN_POINT('Ctrl Pts',(106.223193564612,-0.591831854740231,
-12.4996795564133));
#54950=CARTESIAN_POINT('Ctrl Pts',(106.222440583606,-0.414376610795987,
-12.4995198638745));
#54951=CARTESIAN_POINT('Ctrl Pts',(106.22387013875,-0.236993616228443,-12.4993777643298));
#54952=CARTESIAN_POINT('Ctrl Pts',(106.227481746357,-0.0595633864188738,
-12.4992668820702));
#54953=CARTESIAN_POINT('Ctrl Pts',(106.227751045141,-0.04633333754566,-12.4992586141571));
#54954=CARTESIAN_POINT('Ctrl Pts',(106.22803246533,-0.033103547113014,-12.4992505170535));
#54955=CARTESIAN_POINT('Ctrl Pts',(106.228326003854,-0.0198739657211027,
-12.4992425948726));
#54956=CARTESIAN_POINT('Ctrl Pts',(106.2284066559,-0.016239032903646,-12.4992404181903));
#54957=CARTESIAN_POINT('Ctrl Pts',(106.228488222706,-0.0126041193345105,
-12.4992382547142));
#54958=CARTESIAN_POINT('Ctrl Pts',(106.228570704203,-0.00896922399477974,
-12.4992361045266));
#54959=CARTESIAN_POINT('Ctrl Pts',(106.228619157464,-0.00683392653775541,
-12.4992348414118));
#54960=CARTESIAN_POINT('Ctrl Pts',(106.228667926366,-0.0046986357788803,
-12.499233582883));
#54961=CARTESIAN_POINT('Ctrl Pts',(106.228717010897,-0.00256335143549926,
-12.4992323289566));
#54962=CARTESIAN_POINT('Ctrl Pts',(106.228759389134,-0.000719805535707577,
-12.499231246351));
#54963=CARTESIAN_POINT('Ctrl Pts',(106.228802002639,0.0011237353156715,
-12.4992301671762));
#54964=CARTESIAN_POINT('Ctrl Pts',(106.228844851403,0.00296727129289191,
-12.4992290914429));
#54965=CARTESIAN_POINT('Ctrl Pts',(106.228897035082,0.00521243500223122,
-12.4992277813532));
#54966=CARTESIAN_POINT('Ctrl Pts',(106.228949567684,0.00745759110152448,
-12.499226476368));
#54967=CARTESIAN_POINT('Ctrl Pts',(106.22900244919,0.00970273982115463,
-12.499225176506));
#54968=CARTESIAN_POINT('Ctrl Pts',(106.229102217696,0.0139385332193429,
-12.499222724131));
#54969=CARTESIAN_POINT('Ctrl Pts',(106.229203228059,0.0181742985818641,
-12.4992202899931));
#54970=CARTESIAN_POINT('Ctrl Pts',(106.229305480159,0.0224100375279641,
-12.4992178742175));
#54971=CARTESIAN_POINT('Ctrl Pts',(106.229887912142,0.0465369730381842,
-12.4992041138644));
#54972=CARTESIAN_POINT('Ctrl Pts',(106.230510625946,0.0706627953287636,
-12.4991909496053));
#54973=CARTESIAN_POINT('Ctrl Pts',(106.231173596977,0.0947878029303355,
-12.4991784031374));
#54974=CARTESIAN_POINT('Ctrl Pts',(106.232021250125,0.1256332511997,-12.4991623616326));
#54975=CARTESIAN_POINT('Ctrl Pts',(106.232934690913,0.15647655828141,-12.499147330676));
#54976=CARTESIAN_POINT('Ctrl Pts',(106.233913857501,0.187318345679374,-12.4991333498929));
#54977=CARTESIAN_POINT('Ctrl Pts',(106.238735653156,0.339195256385656,-12.4990645030998));
#54978=CARTESIAN_POINT('Ctrl Pts',(106.245149236366,0.49097111824434,-12.4990214443691));
#54979=CARTESIAN_POINT('Ctrl Pts',(106.253143110002,0.642718595914829,-12.4990066325146));
#54980=CARTESIAN_POINT('Ctrl Pts',(106.265792998464,0.882851071655931,-12.4989831935268));
#54981=CARTESIAN_POINT('Ctrl Pts',(106.282378544058,1.12249522883079,-12.4990322697312));
#54982=CARTESIAN_POINT('Ctrl Pts',(106.302811012959,1.36192005952878,-12.4991430117722));
#54983=CARTESIAN_POINT('Ctrl Pts',(106.312133054,1.471154440791,-12.4991935363494));
#54984=CARTESIAN_POINT('Ctrl Pts',(106.322255839342,1.58034251740705,-12.4992566534061));
#54985=CARTESIAN_POINT('Ctrl Pts',(106.333170942243,1.68950627976311,-12.4993304720331));
#54986=CARTESIAN_POINT('',(104.518885227957,1.68935314531927,-12.5));
#54987=CARTESIAN_POINT('Ctrl Pts',(104.518885227957,1.68966509259281,-12.5005876262282));
#54988=CARTESIAN_POINT('Ctrl Pts',(104.524967683448,1.95296088446919,-12.4652318044223));
#54989=CARTESIAN_POINT('Ctrl Pts',(104.531050138939,2.2151108340558,-12.4215019868369));
#54990=CARTESIAN_POINT('Ctrl Pts',(104.53713259443,2.47557965491845,-12.369372315482));
#54991=CARTESIAN_POINT('Ctrl Pts',(104.584449013111,4.50180932473757,-11.9638470536585));
#54992=CARTESIAN_POINT('Ctrl Pts',(104.631765431792,6.42630483037507,-11.0500013459916));
#54993=CARTESIAN_POINT('Ctrl Pts',(104.679081850473,8.02116966160399,-9.73605173396329));
#54994=CARTESIAN_POINT('Ctrl Pts',(104.726398269154,9.61603449283293,-8.42210212193495));
#54995=CARTESIAN_POINT('Ctrl Pts',(104.773714687835,10.8812686496533,-6.70804860554518));
#54996=CARTESIAN_POINT('Ctrl Pts',(104.821031106515,11.667044580788,-4.79686740039649));
#54997=CARTESIAN_POINT('Ctrl Pts',(104.868347525196,12.4528205119227,-2.8856861952478));
#54998=CARTESIAN_POINT('Ctrl Pts',(104.915663943877,12.7591382173717,-0.777377301340174));
#54999=CARTESIAN_POINT('Ctrl Pts',(104.962980362558,12.5497239122681,1.27839580422383));
#55000=CARTESIAN_POINT('Ctrl Pts',(105.010296781239,12.3403096071644,3.3341689097878));
#55001=CARTESIAN_POINT('Ctrl Pts',(105.05761319992,11.6151632915081,5.33740622700816));
#55002=CARTESIAN_POINT('Ctrl Pts',(105.104929618601,10.4601559449718,7.05088673245123));
#55003=CARTESIAN_POINT('Ctrl Pts',(105.152246037282,9.30514859843542,8.76436723789434));
#55004=CARTESIAN_POINT('Ctrl Pts',(105.199562455963,7.72028022101907,10.1880909315601));
#55005=CARTESIAN_POINT('Ctrl Pts',(105.246878874643,5.8932290754146,11.1534621159742));
#55006=CARTESIAN_POINT('Ctrl Pts',(105.294195293324,4.06617792981017,12.1188333003882));
#55007=CARTESIAN_POINT('Ctrl Pts',(105.341511712005,1.99694401601767,12.6258519755504));
#55008=CARTESIAN_POINT('Ctrl Pts',(105.388828130686,-0.0694364031569377,
12.6144775828521));
#55009=CARTESIAN_POINT('Ctrl Pts',(105.436144549367,-2.1358168223316,12.6031031901538));
#55010=CARTESIAN_POINT('Ctrl Pts',(105.483460968048,-4.19934374688837,12.0733357295948));
#55011=CARTESIAN_POINT('Ctrl Pts',(105.530777386729,-6.01565672686706,11.0879096435399));
#55012=CARTESIAN_POINT('Ctrl Pts',(105.57809380541,-7.8319697068457,10.1024835574851));
#55013=CARTESIAN_POINT('Ctrl Pts',(105.62541022409,-9.40106874224627,8.66139884593429));
#55014=CARTESIAN_POINT('Ctrl Pts',(105.672726642771,-10.5371429608089,6.93530708083006));
#55015=CARTESIAN_POINT('Ctrl Pts',(105.720043061452,-11.6732171793715,5.20921531572579));
#55016=CARTESIAN_POINT('Ctrl Pts',(105.767359480133,-12.3762665810961,3.19811649706804));
#55017=CARTESIAN_POINT('Ctrl Pts',(105.814675898814,-12.5630368705784,1.14016259125187));
#55018=CARTESIAN_POINT('Ctrl Pts',(105.861992317495,-12.7498071600607,-0.917791314564243));
#55019=CARTESIAN_POINT('Ctrl Pts',(105.909308736176,-12.4202983373007,-3.02260030753877));
#55020=CARTESIAN_POINT('Ctrl Pts',(105.956625154857,-11.6135304654158,-4.92501535018149));
#55021=CARTESIAN_POINT('Ctrl Pts',(106.003941573537,-10.8067625935309,-6.82743039282427));
#55022=CARTESIAN_POINT('Ctrl Pts',(106.051257992218,-9.52273567252103,-8.52745148513522));
#55023=CARTESIAN_POINT('Ctrl Pts',(106.098574410899,-7.91350264344085,-9.82376414526043));
#55024=CARTESIAN_POINT('Ctrl Pts',(106.14589082958,-6.30426961436072,-11.1200768053856));
#55025=CARTESIAN_POINT('Ctrl Pts',(106.193207248261,-4.36983047721028,-12.0126810333251));
#55026=CARTESIAN_POINT('Ctrl Pts',(106.240523666942,-2.33925931246893,-12.395875615286));
#55027=CARTESIAN_POINT('Ctrl Pts',(106.24554650739,-2.12370548857135,-12.4365533609729));
#55028=CARTESIAN_POINT('Ctrl Pts',(106.250569347839,-1.90706837865939,-12.4714907060993));
#55029=CARTESIAN_POINT('Ctrl Pts',(106.255592188287,-1.68964924171407,-12.5007055298765));
#55030=CARTESIAN_POINT('',(104.441306474002,-1.6893531453193,-12.5));
#55031=CARTESIAN_POINT('Ctrl Pts',(104.441306474002,-1.689543392924,-12.4994338659969));
#55032=CARTESIAN_POINT('Ctrl Pts',(104.440804568837,-1.68035562471557,-12.4994269115715));
#55033=CARTESIAN_POINT('Ctrl Pts',(104.440308397532,-1.67116754787944,-12.4994200217841));
#55034=CARTESIAN_POINT('Ctrl Pts',(104.439817964464,-1.66197914759247,-12.499413198474));
#55035=CARTESIAN_POINT('Ctrl Pts',(104.426601193732,-1.41435926262478,-12.4992293158366));
#55036=CARTESIAN_POINT('Ctrl Pts',(104.417569714248,-1.1668349916106,-12.4990961157117));
#55037=CARTESIAN_POINT('Ctrl Pts',(104.412774567463,-0.919107466037736,
-12.4990367636774));
#55038=CARTESIAN_POINT('Ctrl Pts',(104.410661772918,-0.809955986798895,
-12.4990106125166));
#55039=CARTESIAN_POINT('Ctrl Pts',(104.409371411855,-0.700764382308139,
-12.4989985641351));
#55040=CARTESIAN_POINT('Ctrl Pts',(104.408907850326,-0.591504241844385,
-12.4990011977212));
#55041=CARTESIAN_POINT('Ctrl Pts',(104.40815486932,-0.414028749507104,-12.4990054755574));
#55042=CARTESIAN_POINT('Ctrl Pts',(104.409584424463,-0.236633170009759,
-12.4990487087553));
#55043=CARTESIAN_POINT('Ctrl Pts',(104.413196032071,-0.059198115721675,
-12.4991274190233));
#55044=CARTESIAN_POINT('Ctrl Pts',(104.413465330855,-0.0459677071079966,
-12.4991332880383));
#55045=CARTESIAN_POINT('Ctrl Pts',(104.413746751044,-0.0327376001033777,
-12.4991393509431));
#55046=CARTESIAN_POINT('Ctrl Pts',(104.414040289568,-0.0195077453537486,
-12.4991456047362));
#55047=CARTESIAN_POINT('Ctrl Pts',(104.414120941615,-0.015872737397679,
-12.4991473230157));
#55048=CARTESIAN_POINT('Ctrl Pts',(104.414202508422,-0.0122377519513052,
-12.4991490557029));
#55049=CARTESIAN_POINT('Ctrl Pts',(104.414284989917,-0.00860278808548892,
-12.4991508027325));
#55050=CARTESIAN_POINT('Ctrl Pts',(104.414333443178,-0.00646745033113518,
-12.4991518290146));
#55051=CARTESIAN_POINT('Ctrl Pts',(104.41438221208,-0.0043321204006724,
-12.499152860246));
#55052=CARTESIAN_POINT('Ctrl Pts',(104.414431296611,-0.00219679803272295,
-12.4991538964133));
#55053=CARTESIAN_POINT('Ctrl Pts',(104.414473674849,-0.000353219273919923,
-12.4991547910117));
#55054=CARTESIAN_POINT('Ctrl Pts',(104.414516288354,0.00149035359713489,
-12.4991556892893));
#55055=CARTESIAN_POINT('Ctrl Pts',(104.414559137117,0.00333392070166297,
-12.4991565912373));
#55056=CARTESIAN_POINT('Ctrl Pts',(104.414611320797,0.00557912236092147,
-12.4991576896812));
#55057=CARTESIAN_POINT('Ctrl Pts',(104.414663853398,0.00782431516533509,
-12.499158793569));
#55058=CARTESIAN_POINT('Ctrl Pts',(104.414716734904,0.0100694993497503,
-12.4991599028846));
#55059=CARTESIAN_POINT('Ctrl Pts',(104.41481650341,0.0143053596477874,-12.4991619957667));
#55060=CARTESIAN_POINT('Ctrl Pts',(104.414917513773,0.0185411874785826,
-12.4991641079682));
#55061=CARTESIAN_POINT('Ctrl Pts',(104.415019765873,0.0227769844685048,
-12.4991662393806));
#55062=CARTESIAN_POINT('Ctrl Pts',(104.415602197855,0.0469042505477953,
-12.4991783799892));
#55063=CARTESIAN_POINT('Ctrl Pts',(104.416224911658,0.0710302595856344,
-12.4991911439495));
#55064=CARTESIAN_POINT('Ctrl Pts',(104.416887882689,0.0951553099302959,
-12.4992045098246));
#55065=CARTESIAN_POINT('Ctrl Pts',(104.417735535892,0.126000814885945,-12.4992215989979));
#55066=CARTESIAN_POINT('Ctrl Pts',(104.418648976744,0.15684394323554,-12.4992396718907));
#55067=CARTESIAN_POINT('Ctrl Pts',(104.419628143405,0.187685316122949,-12.49925867807));
#55068=CARTESIAN_POINT('Ctrl Pts',(104.42444993935,0.339560183550717,-12.4993522718595));
#55069=CARTESIAN_POINT('Ctrl Pts',(104.430863523015,0.491328285835151,-12.4994687385499));
#55070=CARTESIAN_POINT('Ctrl Pts',(104.438857397269,0.643062254578234,-12.4995998677619));
#55071=CARTESIAN_POINT('Ctrl Pts',(104.451539138457,0.883777940103603,-12.4998078953935));
#55072=CARTESIAN_POINT('Ctrl Pts',(104.468176381684,1.12398843422842,-12.5000540750527));
#55073=CARTESIAN_POINT('Ctrl Pts',(104.488679721142,1.36396469732121,-12.500286550178));
#55074=CARTESIAN_POINT('Ctrl Pts',(104.497959102239,1.47257291717617,-12.5003917635403));
#55075=CARTESIAN_POINT('Ctrl Pts',(104.508030367173,1.58113250880452,-12.5004939559224));
#55076=CARTESIAN_POINT('Ctrl Pts',(104.518885227957,1.6896650925929,-12.5005876262282));
#55077=CARTESIAN_POINT('',(102.704599513671,1.68935314531927,-12.5));
#55078=CARTESIAN_POINT('Ctrl Pts',(102.704599513671,1.68928977174207,-12.5008279278805));
#55079=CARTESIAN_POINT('Ctrl Pts',(102.747646849754,3.55224433648731,-12.2477504944552));
#55080=CARTESIAN_POINT('Ctrl Pts',(102.790694185836,5.35885448828508,-11.5735404103196));
#55081=CARTESIAN_POINT('Ctrl Pts',(102.833741521919,6.92975537674916,-10.540794871603));
#55082=CARTESIAN_POINT('Ctrl Pts',(102.881057940599,8.65644536291872,-9.40563007982129));
#55083=CARTESIAN_POINT('Ctrl Pts',(102.92837435928,10.0983564409266,-7.83729039347354));
#55084=CARTESIAN_POINT('Ctrl Pts',(102.975690777961,11.084739184859,-6.02149676662285));
#55085=CARTESIAN_POINT('Ctrl Pts',(103.023007196642,12.0711219287913,-4.20570313977216));
#55086=CARTESIAN_POINT('Ctrl Pts',(103.070323615323,12.6019763386482,-2.14245557241852));
#55087=CARTESIAN_POINT('Ctrl Pts',(103.117640034004,12.6144392551756,-0.0760814319127967));
#55088=CARTESIAN_POINT('Ctrl Pts',(103.164956452685,12.626902171703,1.99029270859294));
#55089=CARTESIAN_POINT('Ctrl Pts',(103.212272871366,12.1209735949009,4.05979342225078));
#55090=CARTESIAN_POINT('Ctrl Pts',(103.259589290047,11.1565649959828,5.88735285142727));
#55091=CARTESIAN_POINT('Ctrl Pts',(103.306905708727,10.1921563970646,7.71491228060374));
#55092=CARTESIAN_POINT('Ctrl Pts',(103.354222127408,8.76926777603044,9.30053042529888));
#55093=CARTESIAN_POINT('Ctrl Pts',(103.401538546089,7.05639594165463,10.4564402365909));
#55094=CARTESIAN_POINT('Ctrl Pts',(103.44885496477,5.34352410727879,11.6123500478829));
#55095=CARTESIAN_POINT('Ctrl Pts',(103.496171383451,3.34066905956132,12.3385515257718));
#55096=CARTESIAN_POINT('Ctrl Pts',(103.543487802132,1.28500655420755,12.5490487393444));
#55097=CARTESIAN_POINT('Ctrl Pts',(103.590804220813,-0.770655951146216,
12.7595459529169));
#55098=CARTESIAN_POINT('Ctrl Pts',(103.638120639494,-2.87912591413628,12.4543389021731));
#55099=CARTESIAN_POINT('Ctrl Pts',(103.685437058174,-4.79072078413387,11.6695698496244));
#55100=CARTESIAN_POINT('Ctrl Pts',(103.732753476855,-6.70231565413145,10.8848007970757));
#55101=CARTESIAN_POINT('Ctrl Pts',(103.780069895536,-8.41703543113655,9.62046974272214));
#55102=CARTESIAN_POINT('Ctrl Pts',(103.827386314217,-9.73182500170104,8.02629729346387));
#55103=CARTESIAN_POINT('Ctrl Pts',(103.874702732898,-11.0466145722655,6.43212484420561));
#55104=CARTESIAN_POINT('Ctrl Pts',(103.922019151579,-11.9614739363894,4.50811100004268));
#55105=CARTESIAN_POINT('Ctrl Pts',(103.96933557026,-12.3680665165972,2.48209523343109));
#55106=CARTESIAN_POINT('Ctrl Pts',(104.016651988941,-12.774659096805,0.456079466819497));
#55107=CARTESIAN_POINT('Ctrl Pts',(104.063968407621,-12.6729848930967,-1.67193822224076));
#55108=CARTESIAN_POINT('Ctrl Pts',(104.111284826302,-12.0750840459337,-3.64996046422953));
#55109=CARTESIAN_POINT('Ctrl Pts',(104.158601244983,-11.4771831987707,-5.62798270621831));
#55110=CARTESIAN_POINT('Ctrl Pts',(104.205917663664,-10.383055708153,-7.4560095011356));
#55111=CARTESIAN_POINT('Ctrl Pts',(104.253234082345,-8.92226687373862,-8.91756805079638));
#55112=CARTESIAN_POINT('Ctrl Pts',(104.300550501026,-7.46147803932427,-10.3791266004572));
#55113=CARTESIAN_POINT('Ctrl Pts',(104.347866919707,-5.63402786111328,-11.4742169048614));
#55114=CARTESIAN_POINT('Ctrl Pts',(104.395183338388,-3.65632085500738,-12.0731596490735));
#55115=CARTESIAN_POINT('Ctrl Pts',(104.410557716926,-3.01371059419662,-12.2677722746447));
#55116=CARTESIAN_POINT('Ctrl Pts',(104.425932095464,-2.35523659191329,-12.4100028771332));
#55117=CARTESIAN_POINT('Ctrl Pts',(104.441306474002,-1.68954339292365,-12.499433865997));
#55118=CARTESIAN_POINT('',(102.627020759716,-1.68935314531929,-12.5));
#55119=CARTESIAN_POINT('Ctrl Pts',(102.627020759716,-1.68914447211972,-12.499042498534));
#55120=CARTESIAN_POINT('Ctrl Pts',(102.626518854552,-1.67995707528232,-12.4990448625818));
#55121=CARTESIAN_POINT('Ctrl Pts',(102.626022683247,-1.67076939350443,-12.4990473235431));
#55122=CARTESIAN_POINT('Ctrl Pts',(102.625532250178,-1.66158141178441,-12.4990498810209));
#55123=CARTESIAN_POINT('Ctrl Pts',(102.612383688404,-1.4152506627532,-12.4991184472672));
#55124=CARTESIAN_POINT('Ctrl Pts',(102.603377330541,-1.1690313997046,-12.4992586077918));
#55125=CARTESIAN_POINT('Ctrl Pts',(102.598563431873,-0.92262521463345,-12.4994487371169));
#55126=CARTESIAN_POINT('Ctrl Pts',(102.596406399541,-0.812214475966295,
-12.4995339310792));
#55127=CARTESIAN_POINT('Ctrl Pts',(102.595091127173,-0.701765534330746,
-12.4996288943628));
#55128=CARTESIAN_POINT('Ctrl Pts',(102.594622136041,-0.591248584118155,
-12.499730091944));
#55129=CARTESIAN_POINT('Ctrl Pts',(102.593869155034,-0.41380991033001,-12.4998925680579));
#55130=CARTESIAN_POINT('Ctrl Pts',(102.595298710177,-0.236456608632446,
-12.500071092898));
#55131=CARTESIAN_POINT('Ctrl Pts',(102.598910317785,-0.059067595309641,
-12.5002449761604));
#55132=CARTESIAN_POINT('Ctrl Pts',(102.599179616569,-0.0458406197222311,
-12.5002579417304));
#55133=CARTESIAN_POINT('Ctrl Pts',(102.599461036759,-0.0326139665295593,
-12.5002708777699));
#55134=CARTESIAN_POINT('Ctrl Pts',(102.599754575282,-0.0193875856951232,
-12.5002837741577));
#55135=CARTESIAN_POINT('Ctrl Pts',(102.599835227328,-0.0157535322845329,
-12.5002873175429));
#55136=CARTESIAN_POINT('Ctrl Pts',(102.599916794133,-0.0121195028984813,
-12.5002908579301));
#55137=CARTESIAN_POINT('Ctrl Pts',(102.599999275632,-0.00848549640073772,
-12.5002943951067));
#55138=CARTESIAN_POINT('Ctrl Pts',(102.600047728893,-0.00635072106825237,
-12.5002964729999));
#55139=CARTESIAN_POINT('Ctrl Pts',(102.600096497797,-0.00421595407720239,
-12.5002985497847));
#55140=CARTESIAN_POINT('Ctrl Pts',(102.600145582325,-0.00208119532421411,
-12.5003006254177));
#55141=CARTESIAN_POINT('Ctrl Pts',(102.600187960563,-0.000238103086124358,
-12.5003024174623));
#55142=CARTESIAN_POINT('Ctrl Pts',(102.600230574068,0.00160498288079793,
-12.5003042086483));
#55143=CARTESIAN_POINT('Ctrl Pts',(102.600273422832,0.00344806271039932,
-12.5003059989476));
#55144=CARTESIAN_POINT('Ctrl Pts',(102.60032560651,0.00569267088955102,
-12.5003081792766));
#55145=CARTESIAN_POINT('Ctrl Pts',(102.60037813911,0.00793726964793562,
-12.5003103582903));
#55146=CARTESIAN_POINT('Ctrl Pts',(102.600431020618,0.0101818593436699,
-12.500312535938));
#55147=CARTESIAN_POINT('Ctrl Pts',(102.600530789125,0.014416597910145,-12.500316644381));
#55148=CARTESIAN_POINT('Ctrl Pts',(102.600631799488,0.0186513020079477,
-12.5003207479601));
#55149=CARTESIAN_POINT('Ctrl Pts',(102.600734051588,0.0228859732661158,
-12.5003248463334));
#55150=CARTESIAN_POINT('Ctrl Pts',(102.60131648357,0.0470068272114195,-12.5003481908287));
#55151=CARTESIAN_POINT('Ctrl Pts',(102.601939197373,0.0711263600042235,
-12.5003713663617));
#55152=CARTESIAN_POINT('Ctrl Pts',(102.602602168403,0.0952448742825837,
-12.5003943084139));
#55153=CARTESIAN_POINT('Ctrl Pts',(102.60344982162,0.126082022963942,-12.5004236413763));
#55154=CARTESIAN_POINT('Ctrl Pts',(102.604363262488,0.156916697488337,-12.5004525920831));
#55155=CARTESIAN_POINT('Ctrl Pts',(102.605342429167,0.187749527997318,-12.500481020301));
#55156=CARTESIAN_POINT('Ctrl Pts',(102.610164225186,0.339582328914088,-12.5006210118578));
#55157=CARTESIAN_POINT('Ctrl Pts',(102.616577808967,0.491306236465511,-12.5007485459572));
#55158=CARTESIAN_POINT('Ctrl Pts',(102.624571683377,0.642994952392699,-12.5008448327383));
#55159=CARTESIAN_POINT('Ctrl Pts',(102.633100273966,0.804830238842706,-12.5009475602136));
#55160=CARTESIAN_POINT('Ctrl Pts',(102.643417815241,0.966434895985585,-12.5010150028948));
#55161=CARTESIAN_POINT('Ctrl Pts',(102.655497113968,1.12789502530787,-12.501019908215));
#55162=CARTESIAN_POINT('Ctrl Pts',(102.669508357471,1.31517884361736,-12.5010255980848));
#55163=CARTESIAN_POINT('Ctrl Pts',(102.685889970392,1.50226880459108,-12.5009473534237));
#55164=CARTESIAN_POINT('Ctrl Pts',(102.704599513671,1.68928977174265,-12.5008279278804));
#55165=CARTESIAN_POINT('',(100.890313799386,1.68935314531927,-12.5));
#55166=CARTESIAN_POINT('Ctrl Pts',(100.890313799386,1.68901725126337,-12.4995884691532));
#55167=CARTESIAN_POINT('Ctrl Pts',(100.923009597379,3.10436959511541,-12.3070954004652));
#55168=CARTESIAN_POINT('Ctrl Pts',(100.955705395371,4.48781279745029,-11.8755333660407));
#55169=CARTESIAN_POINT('Ctrl Pts',(100.988401193364,5.75826554513978,-11.2237357425437));
#55170=CARTESIAN_POINT('Ctrl Pts',(101.035717612045,7.59682822946574,-10.2804729643937));
#55171=CARTESIAN_POINT('Ctrl Pts',(101.083034030726,9.1987544835431,-8.87596977637554));
#55172=CARTESIAN_POINT('Ctrl Pts',(101.130350449407,10.3743460711825,-7.17654580575761));
#55173=CARTESIAN_POINT('Ctrl Pts',(101.177666868088,11.5499376588219,-5.47712183513971));
#55174=CARTESIAN_POINT('Ctrl Pts',(101.224983286769,12.2991945800233,-3.48277708192202));
#55175=CARTESIAN_POINT('Ctrl Pts',(101.27229970545,12.533390705202,-1.42967952267392));
#55176=CARTESIAN_POINT('Ctrl Pts',(101.31961612413,12.7675868303807,0.62341803657417));
#55177=CARTESIAN_POINT('Ctrl Pts',(101.366932542811,12.4867221595366,2.73526840185267));
#55178=CARTESIAN_POINT('Ctrl Pts',(101.414248961492,11.7240563589818,4.65578871924149));
#55179=CARTESIAN_POINT('Ctrl Pts',(101.461565380173,10.9613905584269,6.57630903663028));
#55180=CARTESIAN_POINT('Ctrl Pts',(101.508881798854,9.71692362816134,8.3054993061294));
#55181=CARTESIAN_POINT('Ctrl Pts',(101.556198217535,8.13802388870941,9.63859083546926));
#55182=CARTESIAN_POINT('Ctrl Pts',(101.603514636216,6.55912414925745,10.9716823648091));
#55183=CARTESIAN_POINT('Ctrl Pts',(101.650831054897,4.64579160061914,11.9086751539898));
#55184=CARTESIAN_POINT('Ctrl Pts',(101.698147473577,2.62460084870815,12.3386116111886));
#55185=CARTESIAN_POINT('Ctrl Pts',(101.745463892258,0.603410096797157,12.7685480683874));
#55186=CARTESIAN_POINT('Ctrl Pts',(101.792780310939,-1.52563885838652,12.6914281936044));
#55187=CARTESIAN_POINT('Ctrl Pts',(101.84009672962,-3.51042652599171,12.1163844323466));
#55188=CARTESIAN_POINT('Ctrl Pts',(101.887413148301,-5.4952141935969,11.5413406710888));
#55189=CARTESIAN_POINT('Ctrl Pts',(101.934729566982,-7.3357405736236,10.4683730233561));
#55190=CARTESIAN_POINT('Ctrl Pts',(101.982045985663,-8.81405268161804,9.02454106492175));
#55191=CARTESIAN_POINT('Ctrl Pts',(102.029362404344,-10.2923647896125,7.58070910648745));
#55192=CARTESIAN_POINT('Ctrl Pts',(102.076678823025,-11.4084626255746,5.76601283735156));
#55193=CARTESIAN_POINT('Ctrl Pts',(102.123995241705,-12.030179187211,3.79534647040199));
#55194=CARTESIAN_POINT('Ctrl Pts',(102.171311660386,-12.6518957488473,1.8246801034524));
#55195=CARTESIAN_POINT('Ctrl Pts',(102.218628079067,-12.7792310361579,-0.301956361310865));
#55196=CARTESIAN_POINT('Ctrl Pts',(102.265944497748,-12.3971061531285,-2.33272911733478));
#55197=CARTESIAN_POINT('Ctrl Pts',(102.313260916429,-12.0149812700991,-4.3635018733587));
#55198=CARTESIAN_POINT('Ctrl Pts',(102.36057733511,-11.1233962167298,-6.29841092064327));
#55199=CARTESIAN_POINT('Ctrl Pts',(102.407893753791,-9.82793145379795,-7.90832658950336));
#55200=CARTESIAN_POINT('Ctrl Pts',(102.455210172472,-8.53246669086617,-9.51824225836343));
#55201=CARTESIAN_POINT('Ctrl Pts',(102.502526591152,-6.8331222183719,-10.803164548799));
#55202=CARTESIAN_POINT('Ctrl Pts',(102.549843009833,-4.93113242415901,-11.6109344637805));
#55203=CARTESIAN_POINT('Ctrl Pts',(102.575568926461,-3.89702138540229,-12.0501186215501));
#55204=CARTESIAN_POINT('Ctrl Pts',(102.601294843088,-2.80300652002858,-12.3482521351367));
#55205=CARTESIAN_POINT('Ctrl Pts',(102.627020759716,-1.68914447211892,-12.4990424985341));
#55206=CARTESIAN_POINT('',(100.81273504543,-1.68935314531929,-12.5));
#55207=CARTESIAN_POINT('Ctrl Pts',(100.81273504543,-1.68904687944112,-12.5000065800334));
#55208=CARTESIAN_POINT('Ctrl Pts',(100.812233140265,-1.67986234589066,-12.5000153813875));
#55209=CARTESIAN_POINT('Ctrl Pts',(100.811736968961,-1.67067753085417,-12.500024197569));
#55210=CARTESIAN_POINT('Ctrl Pts',(100.811246535893,-1.6614924188256,-12.5000330258491));
#55211=CARTESIAN_POINT('Ctrl Pts',(100.798193427403,-1.41702631010753,-12.5002679947065));
#55212=CARTESIAN_POINT('Ctrl Pts',(100.789222599649,-1.17267204576433,-12.5005136843555));
#55213=CARTESIAN_POINT('Ctrl Pts',(100.784383221339,-0.928128757686291,
-12.5007042010178));
#55214=CARTESIAN_POINT('Ctrl Pts',(100.782163525937,-0.81596319065912,-12.5007915859942));
#55215=CARTESIAN_POINT('Ctrl Pts',(100.780813011206,-0.70375717139188,-12.5008670670383));
#55216=CARTESIAN_POINT('Ctrl Pts',(100.780336421755,-0.591478528683606,
-12.500922451509));
#55217=CARTESIAN_POINT('Ctrl Pts',(100.779810184042,-0.467503363071267,
-12.5009836056052));
#55218=CARTESIAN_POINT('Ctrl Pts',(100.780349946661,-0.343566876696398,
-12.5010201462746));
#55219=CARTESIAN_POINT('Ctrl Pts',(100.781955544507,-0.219626668121229,
-12.5010194195077));
#55220=CARTESIAN_POINT('Ctrl Pts',(100.782647358368,-0.166223784873483,
-12.5010191063612));
#55221=CARTESIAN_POINT('Ctrl Pts',(100.783537049102,-0.112820200000195,
-12.5010118523632));
#55222=CARTESIAN_POINT('Ctrl Pts',(100.784624603499,-0.0594125214676394,
-12.500998703149));
#55223=CARTESIAN_POINT('Ctrl Pts',(100.784893902284,-0.046187782611698,
-12.5009954471579));
#55224=CARTESIAN_POINT('Ctrl Pts',(100.785175322473,-0.0329633147788684,
-12.5009918295968));
#55225=CARTESIAN_POINT('Ctrl Pts',(100.785468860997,-0.0197390670073646,
-12.5009878659091));
#55226=CARTESIAN_POINT('Ctrl Pts',(100.785549513043,-0.0161055996369931,
-12.5009867768544));
#55227=CARTESIAN_POINT('Ctrl Pts',(100.785631079849,-0.0124721523439735,
-12.5009856616697));
#55228=CARTESIAN_POINT('Ctrl Pts',(100.785713561346,-0.0088387240911394,
-12.5009845206726));
#55229=CARTESIAN_POINT('Ctrl Pts',(100.785762014606,-0.00670428845895918,
-12.5009838504007));
#55230=CARTESIAN_POINT('Ctrl Pts',(100.785810783508,-0.00456985979954622,
-12.5009831712213));
#55231=CARTESIAN_POINT('Ctrl Pts',(100.78585986804,-0.00243543782588915,
-12.5009824831985));
#55232=CARTESIAN_POINT('Ctrl Pts',(100.785902246277,-0.000592636453217514,
-12.5009818891786));
#55233=CARTESIAN_POINT('Ctrl Pts',(100.785944859783,0.00125015967138045,
-12.5009812885668));
#55234=CARTESIAN_POINT('Ctrl Pts',(100.785987708546,0.00309295067176889,
-12.5009806814044));
#55235=CARTESIAN_POINT('Ctrl Pts',(100.786039892226,0.00533720716887695,
-12.5009799419672));
#55236=CARTESIAN_POINT('Ctrl Pts',(100.786092424827,0.00758145576628483,
-12.5009791928144));
#55237=CARTESIAN_POINT('Ctrl Pts',(100.786145306333,0.00982569664479346,
-12.5009784340204));
#55238=CARTESIAN_POINT('Ctrl Pts',(100.786245074838,0.0140597773254563,
-12.5009770024471));
#55239=CARTESIAN_POINT('Ctrl Pts',(100.786346085201,0.0182938289677911,
-12.5009755365572));
#55240=CARTESIAN_POINT('Ctrl Pts',(100.786448337302,0.0225278532933111,
-12.5009740368479));
#55241=CARTESIAN_POINT('Ctrl Pts',(100.787030769284,0.0466450220426878,
-12.5009654944453));
#55242=CARTESIAN_POINT('Ctrl Pts',(100.787653483087,0.0707610468272474,
-12.5009558550683));
#55243=CARTESIAN_POINT('Ctrl Pts',(100.788316454117,0.0948762357697601,
-12.5009452092726));
#55244=CARTESIAN_POINT('Ctrl Pts',(100.789164107338,0.125709132916537,-12.5009315979041));
#55245=CARTESIAN_POINT('Ctrl Pts',(100.79007754821,0.156539854627723,-12.5009163418817));
#55246=CARTESIAN_POINT('Ctrl Pts',(100.791056714894,0.187369042442589,-12.5008996248898));
#55247=CARTESIAN_POINT('Ctrl Pts',(100.795878510932,0.339183905208656,-12.5008173039462));
#55248=CARTESIAN_POINT('Ctrl Pts',(100.802292094743,0.490897403440178,-12.5006999080129));
#55249=CARTESIAN_POINT('Ctrl Pts',(100.810285969195,0.642584577087836,-12.5005670786308));
#55250=CARTESIAN_POINT('Ctrl Pts',(100.822840468179,0.880811544388206,-12.500358468106));
#55251=CARTESIAN_POINT('Ctrl Pts',(100.839271492313,1.11856274394623,-12.5001140814977));
#55252=CARTESIAN_POINT('Ctrl Pts',(100.859492300037,1.3561101677418,-12.4998886286552));
#55253=CARTESIAN_POINT('Ctrl Pts',(100.868941507161,1.4671163570085,-12.499783274278));
#55254=CARTESIAN_POINT('Ctrl Pts',(100.879218290784,1.57807738894463,-12.49968175614));
#55255=CARTESIAN_POINT('Ctrl Pts',(100.890313799386,1.68901725126355,-12.4995884691532));
#55256=CARTESIAN_POINT('',(99.0760280851,1.68935314531928,-12.5));
#55257=CARTESIAN_POINT('Ctrl Pts',(99.0760280851,1.68926961768441,-12.4990067873254));
#55258=CARTESIAN_POINT('Ctrl Pts',(99.0983723450034,2.65676718946135,-12.3683919466809));
#55259=CARTESIAN_POINT('Ctrl Pts',(99.1207166049067,3.60921449755032,-12.1266511028957));
#55260=CARTESIAN_POINT('Ctrl Pts',(99.1430608648101,4.52023710773274,-11.7769827456882));
#55261=CARTESIAN_POINT('Ctrl Pts',(99.190377283491,6.44942730859747,-11.0365216849666));
#55262=CARTESIAN_POINT('Ctrl Pts',(99.2376937021719,8.19285796673946,-9.81208448069556));
#55263=CARTESIAN_POINT('Ctrl Pts',(99.2850101208527,9.54407406006468,-8.24866755565912));
#55264=CARTESIAN_POINT('Ctrl Pts',(99.3323265395336,10.8952901533899,-6.68525063062268));
#55265=CARTESIAN_POINT('Ctrl Pts',(99.3796429582144,11.8542916818983,-4.78285398482082));
#55266=CARTESIAN_POINT('Ctrl Pts',(99.4269593768953,12.3075148043826,-2.76675720779547));
#55267=CARTESIAN_POINT('Ctrl Pts',(99.4742757955762,12.7607379268669,-0.750660430770102));
#55268=CARTESIAN_POINT('Ctrl Pts',(99.5215922142571,12.708182643327,1.37913647747874));
#55269=CARTESIAN_POINT('Ctrl Pts',(99.568908632938,12.1560724891477,3.37042545459742));
#55270=CARTESIAN_POINT('Ctrl Pts',(99.6162250516189,11.6039623349683,5.3617144317161));
#55271=CARTESIAN_POINT('Ctrl Pts',(99.6635414702997,10.5522973101494,7.2144954777046));
#55272=CARTESIAN_POINT('Ctrl Pts',(99.7108578889806,9.12561435869646,8.70936442476912));
#55273=CARTESIAN_POINT('Ctrl Pts',(99.7581743076614,7.69893140724353,10.2042333718336));
#55274=CARTESIAN_POINT('Ctrl Pts',(99.8054907263423,5.89723052915655,11.3411902199742));
#55275=CARTESIAN_POINT('Ctrl Pts',(99.8528071450232,3.93386703831174,11.9855978670874));
#55276=CARTESIAN_POINT('Ctrl Pts',(99.9001235637041,1.97050354746692,12.6300055142007));
#55277=CARTESIAN_POINT('Ctrl Pts',(99.947439982385,-0.154522556135726,12.7818639602866));
#55278=CARTESIAN_POINT('Ctrl Pts',(99.9947564010659,-2.18956816304055,12.4231903054835));
#55279=CARTESIAN_POINT('Ctrl Pts',(100.042072819747,-4.22461376994535,12.0645166506804));
#55280=CARTESIAN_POINT('Ctrl Pts',(100.089389238428,-6.16967888015232,11.1953108949882));
#55281=CARTESIAN_POINT('Ctrl Pts',(100.136705657109,-7.79443115486138,9.91850336890124));
#55282=CARTESIAN_POINT('Ctrl Pts',(100.184022075789,-9.41918342957046,8.64169584281428));
#55283=CARTESIAN_POINT('Ctrl Pts',(100.23133849447,-10.7236228687816,6.95728654633254));
#55284=CARTESIAN_POINT('Ctrl Pts',(100.278654913151,-11.5532792775025,5.06474126119284));
#55285=CARTESIAN_POINT('Ctrl Pts',(100.325971331832,-12.3829356862234,3.17219597605314));
#55286=CARTESIAN_POINT('Ctrl Pts',(100.373287750513,-12.737809064454,1.07151470225547));
#55287=CARTESIAN_POINT('Ctrl Pts',(100.420604169194,-12.5758757211841,-0.988542337046582));
#55288=CARTESIAN_POINT('Ctrl Pts',(100.467920587875,-12.4139423779141,-3.04859937634864));
#55289=CARTESIAN_POINT('Ctrl Pts',(100.515237006556,-11.7352023131437,-5.06803218115509));
#55290=CARTESIAN_POINT('Ctrl Pts',(100.562553425236,-10.6200311326729,-6.80770187712794));
#55291=CARTESIAN_POINT('Ctrl Pts',(100.609869843917,-9.5048599522022,-8.5473715731008));
#55292=CARTESIAN_POINT('Ctrl Pts',(100.657186262598,-7.95325765603118,-10.00727816024));
#55293=CARTESIAN_POINT('Ctrl Pts',(100.704502681279,-6.14896317602482,-11.0145412054561));
#55294=CARTESIAN_POINT('Ctrl Pts',(100.740580135996,-4.77323876125789,-11.7825512940261));
#55295=CARTESIAN_POINT('Ctrl Pts',(100.776657590713,-3.25060823709326,-12.2874107750916));
#55296=CARTESIAN_POINT('Ctrl Pts',(100.81273504543,-1.68904687944152,-12.5000065800333));
#55297=CARTESIAN_POINT('',(98.9984493311445,-1.68935314531929,-12.5));
#55298=CARTESIAN_POINT('Ctrl Pts',(98.9984493311444,-1.68945110984984,-12.5010138634865));
#55299=CARTESIAN_POINT('Ctrl Pts',(98.9979474259811,-1.6802677427303,-12.5010150828114));
#55300=CARTESIAN_POINT('Ctrl Pts',(98.9974512546758,-1.67108405301431,-12.5010161252244));
#55301=CARTESIAN_POINT('Ctrl Pts',(98.9969608216067,-1.66190002447542,-12.5010169855558));
#55302=CARTESIAN_POINT('Ctrl Pts',(98.9953653343946,-1.63202234898023,-12.5010197844042));
#55303=CARTESIAN_POINT('Ctrl Pts',(98.993830837603,-1.60214584008525,-12.501020667113));
#55304=CARTESIAN_POINT('Ctrl Pts',(98.9923574210217,-1.57226996295488,-12.5010194467146));
#55305=CARTESIAN_POINT('Ctrl Pts',(98.9800706385758,-1.32313580271385,-12.501009269844));
#55306=CARTESIAN_POINT('Ctrl Pts',(98.9720312814802,-1.0740498127315,-12.5008541512912));
#55307=CARTESIAN_POINT('Ctrl Pts',(98.9682914170034,-0.824698135317126,
-12.5006462662282));
#55308=CARTESIAN_POINT('Ctrl Pts',(98.9671276888522,-0.747107739094962,
-12.5005815789376));
#55309=CARTESIAN_POINT('Ctrl Pts',(98.9663802627598,-0.669491254130434,
-12.5005116497004));
#55310=CARTESIAN_POINT('Ctrl Pts',(98.9660507074694,-0.591838307311,-12.5004388277769));
#55311=CARTESIAN_POINT('Ctrl Pts',(98.9652977264628,-0.414413772565412,
-12.5002724413558));
#55312=CARTESIAN_POINT('Ctrl Pts',(98.9667272816058,-0.237059727277439,
-12.5000915331407));
#55313=CARTESIAN_POINT('Ctrl Pts',(98.9703388892135,-0.0596558322633638,
-12.4999195073644));
#55314=CARTESIAN_POINT('Ctrl Pts',(98.9706081879978,-0.0464277470335215,
-12.4999066802975));
#55315=CARTESIAN_POINT('Ctrl Pts',(98.970889608187,-0.0331999056257905,
-12.4998939000497));
#55316=CARTESIAN_POINT('Ctrl Pts',(98.9711831467108,-0.019972258301805,
-12.4998811748209));
#55317=CARTESIAN_POINT('Ctrl Pts',(98.9712637987576,-0.0163378568726815,
-12.4998776784629));
#55318=CARTESIAN_POINT('Ctrl Pts',(98.971345365564,-0.0127034735610646,
-12.4998741862605));
#55319=CARTESIAN_POINT('Ctrl Pts',(98.9714278470603,-0.00906910737247381,
-12.499870698381));
#55320=CARTESIAN_POINT('Ctrl Pts',(98.9714763003207,-0.00693412074554248,
-12.4998686494471));
#55321=CARTESIAN_POINT('Ctrl Pts',(98.9715250692229,-0.00479914042401758,
-12.4998666020053));
#55322=CARTESIAN_POINT('Ctrl Pts',(98.971574153754,-0.00266416613580766,
-12.4998645560894));
#55323=CARTESIAN_POINT('Ctrl Pts',(98.9716165319915,-0.000820887908404128,
-12.4998627897016));
#55324=CARTESIAN_POINT('Ctrl Pts',(98.9716591454966,0.00102238556451054,
-12.4998610244515));
#55325=CARTESIAN_POINT('Ctrl Pts',(98.9717019942601,0.00286565441603858,
-12.4998592603605));
#55326=CARTESIAN_POINT('Ctrl Pts',(98.9717541779398,0.00511049285387701,
-12.4998571119494));
#55327=CARTESIAN_POINT('Ctrl Pts',(98.9718067105416,0.00735532411911638,
-12.499854965258));
#55328=CARTESIAN_POINT('Ctrl Pts',(98.9718595920468,0.00960014839710077,
-12.499852820325));
#55329=CARTESIAN_POINT('Ctrl Pts',(98.9719593605523,0.0138353297160231,
-12.4998487736029));
#55330=CARTESIAN_POINT('Ctrl Pts',(98.9720603709144,0.018070484562572,-12.4998447331417));
#55331=CARTESIAN_POINT('Ctrl Pts',(98.9721626230162,0.0223056146626419,
-12.4998406992006));
#55332=CARTESIAN_POINT('Ctrl Pts',(98.9727450549982,0.0464290817843739,
-12.4998177217141));
#55333=CARTESIAN_POINT('Ctrl Pts',(98.9733677688012,0.0705514868195058,
-12.4997949562095));
#55334=CARTESIAN_POINT('Ctrl Pts',(98.9740307398311,0.094673130418238,-12.4997724491959));
#55335=CARTESIAN_POINT('Ctrl Pts',(98.9748783930467,0.125514280088803,-12.4997436724596));
#55336=CARTESIAN_POINT('Ctrl Pts',(98.9757918339131,0.156353375762838,-12.4997153192498));
#55337=CARTESIAN_POINT('Ctrl Pts',(98.9767710005896,0.187191043402697,-12.4996874810608));
#55338=CARTESIAN_POINT('Ctrl Pts',(98.9815927965995,0.339047664282832,-12.4995503950348));
#55339=CARTESIAN_POINT('Ctrl Pts',(98.9880063803661,0.490805467490059,-12.4994261570224));
#55340=CARTESIAN_POINT('Ctrl Pts',(98.9960002547573,0.642537640964607,-12.499323396877));
#55341=CARTESIAN_POINT('Ctrl Pts',(99.008622407575,0.882119424117457,-12.4991611408552));
#55342=CARTESIAN_POINT('Ctrl Pts',(99.0251629778626,1.12122192559231,-12.4990545261512));
#55343=CARTESIAN_POINT('Ctrl Pts',(99.0455338141878,1.36011436106045,-12.499016424172));
#55344=CARTESIAN_POINT('Ctrl Pts',(99.0548929207919,1.46987027558398,-12.4989989187304));
#55345=CARTESIAN_POINT('Ctrl Pts',(99.0650605273681,1.57958119595339,-12.4989956130992));
#55346=CARTESIAN_POINT('Ctrl Pts',(99.0760280851,1.68926961768503,-12.4990067873254));
#55347=CARTESIAN_POINT('Ctrl Pts',(97.2617423708144,1.68963646449132,-12.4998270697761));
#55348=CARTESIAN_POINT('Ctrl Pts',(97.2737350926282,2.20887124184649,-12.4301620153288));
#55349=CARTESIAN_POINT('Ctrl Pts',(97.285727814442,2.72368641886456,-12.3282504960299));
#55350=CARTESIAN_POINT('Ctrl Pts',(97.2977205362559,3.22997473648381,-12.1941459828224));
#55351=CARTESIAN_POINT('Ctrl Pts',(97.3450369549367,5.22749876660567,-11.6650463011637));
#55352=CARTESIAN_POINT('Ctrl Pts',(97.3923533736176,7.09229028452064,-10.6348175686913));
#55353=CARTESIAN_POINT('Ctrl Pts',(97.4396697922984,8.6035177604385,-9.22547184209238));
#55354=CARTESIAN_POINT('Ctrl Pts',(97.4869862109793,10.1147452363564,-7.81612611549341));
#55355=CARTESIAN_POINT('Ctrl Pts',(97.5343026296602,11.2724086702771,-6.02766339476788));
#55356=CARTESIAN_POINT('Ctrl Pts',(97.5816190483411,11.9394213573864,-4.07186482841795));
#55357=CARTESIAN_POINT('Ctrl Pts',(97.628935467022,12.6064340444957,-2.11606626206803));
#55358=CARTESIAN_POINT('Ctrl Pts',(97.6762518857028,12.7827959847935,0.00706814990629356));
#55359=CARTESIAN_POINT('Ctrl Pts',(97.7235683043837,12.447621428183,2.04611617989715));
#55360=CARTESIAN_POINT('Ctrl Pts',(97.7708847230646,12.1124468715726,4.085164209888));
#55361=CARTESIAN_POINT('Ctrl Pts',(97.8182011417455,11.2657358180539,6.04012585789538));
#55362=CARTESIAN_POINT('Ctrl Pts',(97.8655175604264,10.0077553660322,7.67949835174444));
#55363=CARTESIAN_POINT('Ctrl Pts',(97.9128339791073,8.74977491401052,9.3188708455935));
#55364=CARTESIAN_POINT('Ctrl Pts',(97.9601503977881,7.08052506348581,10.6426541852842));
#55365=CARTESIAN_POINT('Ctrl Pts',(98.007466816469,5.19767616134277,11.4940867719376));
#55366=CARTESIAN_POINT('Ctrl Pts',(98.0547832351499,3.31482725919971,12.345519358591));
#55367=CARTESIAN_POINT('Ctrl Pts',(98.1020996538307,1.21837930543832,12.724601192207));
#55368=CARTESIAN_POINT('Ctrl Pts',(98.1494160725116,-0.843408651483552,
12.586442191364));
#55369=CARTESIAN_POINT('Ctrl Pts',(98.1967324911925,-2.90519660840542,12.4482831905211));
#55370=CARTESIAN_POINT('Ctrl Pts',(98.2440489098734,-4.93232456848778,11.7928833552192));
#55371=CARTESIAN_POINT('Ctrl Pts',(98.2913653285542,-6.68474246857545,10.6978542021024));
#55372=CARTESIAN_POINT('Ctrl Pts',(98.3386817472351,-8.43716036866312,9.60282504898553));
#55373=CARTESIAN_POINT('Ctrl Pts',(98.385998165916,-9.91486820875611,8.0681665780538));
#55374=CARTESIAN_POINT('Ctrl Pts',(98.4333145845969,-10.9428775221743,6.27561133310073));
#55375=CARTESIAN_POINT('Ctrl Pts',(98.4806310032778,-11.9708868355925,4.48305608814765));
#55376=CARTESIAN_POINT('Ctrl Pts',(98.5279474219587,-12.5491976223359,2.43260406917324));
#55377=CARTESIAN_POINT('Ctrl Pts',(98.5752638406395,-12.6093270088307,0.367067371252128));
#55378=CARTESIAN_POINT('Ctrl Pts',(98.6225802593204,-12.6694563953254,-1.69846932666899));
#55379=CARTESIAN_POINT('Ctrl Pts',(98.6698966780013,-12.2114043815716,-3.77909070353679));
#55380=CARTESIAN_POINT('Ctrl Pts',(98.7172130966822,-11.28941294518,-5.62841198733738));
#55381=CARTESIAN_POINT('Ctrl Pts',(98.7645295153631,-10.3674215087885,-7.47773327113796));
#55382=CARTESIAN_POINT('Ctrl Pts',(98.811845934044,-8.98149064975927,-9.09575446187132));
#55383=CARTESIAN_POINT('Ctrl Pts',(98.8591623527248,-7.29574068517416,-10.2908713885963));
#55384=CARTESIAN_POINT('Ctrl Pts',(98.9055913455314,-5.64160719068382,-11.4635737346495));
#55385=CARTESIAN_POINT('Ctrl Pts',(98.9520203383379,-3.69879542401664,-12.2290863120461));
#55386=CARTESIAN_POINT('Ctrl Pts',(98.9984493311445,-1.68945110984913,-12.5010138634866));
#55387=CARTESIAN_POINT('Ctrl Pts',(107.547344722949,1.01347785817195,-11.5532729648613));
#55388=CARTESIAN_POINT('Ctrl Pts',(107.609159016559,3.48672851139089,-11.3363141184487));
#55389=CARTESIAN_POINT('Ctrl Pts',(107.701880456974,7.0775262685878,-9.77461236926229));
#55390=CARTESIAN_POINT('Ctrl Pts',(107.825509044195,10.2343745743181,-5.85997992529276));
#55391=CARTESIAN_POINT('Ctrl Pts',(107.949137631415,12.0158490350764,-1.15276339618737));
#55392=CARTESIAN_POINT('Ctrl Pts',(108.072766218635,11.3809885644172,4.02471057714319));
#55393=CARTESIAN_POINT('Ctrl Pts',(108.227301952661,7.79854554867288,9.20330948728365));
#55394=CARTESIAN_POINT('Ctrl Pts',(108.320023393076,4.34404808711794,11.0362375708885));
#55395=CARTESIAN_POINT('Ctrl Pts',(108.381837686686,1.89465380507476,11.4418329182223));
#55396=CARTESIAN_POINT('Ctrl Pts',(107.742874014115,1.04307277299664,-11.8906440545054));
#55397=CARTESIAN_POINT('Ctrl Pts',(107.804688307725,3.58854566751268,-11.667349718345));
#55398=CARTESIAN_POINT('Ctrl Pts',(107.89740974814,7.28419954260115,-10.0600441803081));
#55399=CARTESIAN_POINT('Ctrl Pts',(108.02103833536,10.5332320593325,-6.03109921059844));
#55400=CARTESIAN_POINT('Ctrl Pts',(108.144666922581,12.3667279673315,-1.18642563581908));
#55401=CARTESIAN_POINT('Ctrl Pts',(108.268295509801,11.7133287181453,4.14223753223569));
#55402=CARTESIAN_POINT('Ctrl Pts',(108.422831243826,8.0262735541824,9.47205848676629));
#55403=CARTESIAN_POINT('Ctrl Pts',(108.515552684241,4.47090012645561,11.3585105325147));
#55404=CARTESIAN_POINT('Ctrl Pts',(108.577366977851,1.94998024119902,11.7759498088114));
#55405=CARTESIAN_POINT('Ctrl Pts',(107.93840330528,1.07266768782132,-12.2280151441495));
#55406=CARTESIAN_POINT('Ctrl Pts',(108.00021759889,3.69036282363445,-11.9983853182413));
#55407=CARTESIAN_POINT('Ctrl Pts',(108.092939039306,7.49087281661451,-10.3454759913538));
#55408=CARTESIAN_POINT('Ctrl Pts',(108.216567626526,10.8320895443469,-6.20221849590413));
#55409=CARTESIAN_POINT('Ctrl Pts',(108.340196213746,12.7176068995866,-1.2200878754508));
#55410=CARTESIAN_POINT('Ctrl Pts',(108.463824800966,12.0456688718733,4.25976448732819));
#55411=CARTESIAN_POINT('Ctrl Pts',(108.618360534992,8.25400155969191,9.74080748624894));
#55412=CARTESIAN_POINT('Ctrl Pts',(108.711081975407,4.59775216579328,11.6807834941409));
#55413=CARTESIAN_POINT('Ctrl Pts',(108.772896269017,2.00530667732328,12.1100666994004));
#55414=CARTESIAN_POINT('Ctrl Pts',(108.133932596446,1.10226260264601,-12.5653862337935));
#55415=CARTESIAN_POINT('Ctrl Pts',(108.195746890056,3.79217997975623,-12.3294209181376));
#55416=CARTESIAN_POINT('Ctrl Pts',(108.288468330471,7.69754609062786,-10.6309078023996));
#55417=CARTESIAN_POINT('Ctrl Pts',(108.412096917691,11.1309470293613,-6.37333778120981));
#55418=CARTESIAN_POINT('Ctrl Pts',(108.535725504912,13.0684858318418,-1.2537501150825));
#55419=CARTESIAN_POINT('Ctrl Pts',(108.659354092132,12.3780090256014,4.37729144242069));
#55420=CARTESIAN_POINT('Ctrl Pts',(108.813889826157,8.48172956520142,10.0095564857316));
#55421=CARTESIAN_POINT('Ctrl Pts',(108.906611266572,4.72460420513094,12.0030564557671));
#55422=CARTESIAN_POINT('Ctrl Pts',(108.968425560183,2.06063311344754,12.4441835899895));
#55423=CARTESIAN_POINT('',(108.966713351645,2.13438641081836,12.4317460036358));
#55424=CARTESIAN_POINT('Ctrl Pts',(108.966713351645,2.13438197832376,12.4317378478958));
#55425=CARTESIAN_POINT('Ctrl Pts',(108.904270759855,2.11878011600994,12.3247891977871));
#55426=CARTESIAN_POINT('Ctrl Pts',(108.841707114744,2.10024321437466,12.2180180253493));
#55427=CARTESIAN_POINT('Ctrl Pts',(108.779287547041,2.07859884281513,12.111899302578));
#55428=CARTESIAN_POINT('Ctrl Pts',(108.744012990319,2.06636717187634,12.051929471908));
#55429=CARTESIAN_POINT('Ctrl Pts',(108.708784446274,2.05314400460933,11.9921676130932));
#55430=CARTESIAN_POINT('Ctrl Pts',(108.673649764967,2.03890467453726,11.9326960190957));
#55431=CARTESIAN_POINT('Ctrl Pts',(108.614852890925,2.01507556707034,11.8331720248194));
#55432=CARTESIAN_POINT('Ctrl Pts',(108.556034583919,1.98828429254243,11.7339812222009));
#55433=CARTESIAN_POINT('Ctrl Pts',(108.497516928003,1.95832745664509,11.6356749683345));
#55434=CARTESIAN_POINT('Ctrl Pts',(108.458794424042,1.93850431645706,11.5706234168811));
#55435=CARTESIAN_POINT('Ctrl Pts',(108.420203568548,1.91729608573862,11.5059586389564));
#55436=CARTESIAN_POINT('Ctrl Pts',(108.381837686686,1.89465380507476,11.4418329182223));
#55437=CARTESIAN_POINT('',(108.14853343171,1.73584852417216,-12.4932937197078));
#55438=CARTESIAN_POINT('Ctrl Pts',(108.14853343171,1.73578194556693,-12.4930929274479));
#55439=CARTESIAN_POINT('Ctrl Pts',(108.205480780232,4.19849975430616,-12.1469930389749));
#55440=CARTESIAN_POINT('Ctrl Pts',(108.262428128754,6.55419777563119,-11.0556206944382));
#55441=CARTESIAN_POINT('Ctrl Pts',(108.319375477276,8.40808350233105,-9.40044147486277));
#55442=CARTESIAN_POINT('Ctrl Pts',(108.350282624081,9.41424655999455,-8.50212279180473));
#55443=CARTESIAN_POINT('Ctrl Pts',(108.381189770886,10.2725967946779,-7.43773028650731));
#55444=CARTESIAN_POINT('Ctrl Pts',(108.412096917691,10.9439642623296,-6.2655855755927));
#55445=CARTESIAN_POINT('Ctrl Pts',(108.443004064496,11.6153317299814,-5.09344086467804));
#55446=CARTESIAN_POINT('Ctrl Pts',(108.473911211301,12.0997164306015,-3.81354394814619));
#55447=CARTESIAN_POINT('Ctrl Pts',(108.504818358107,12.3650998304949,-2.49102587399968));
#55448=CARTESIAN_POINT('Ctrl Pts',(108.566632651717,12.8958666302817,0.154010274293264));
#55449=CARTESIAN_POINT('Ctrl Pts',(108.628446945327,12.5506282271615,2.96953105304482));
#55450=CARTESIAN_POINT('Ctrl Pts',(108.690261238937,11.3965409033481,5.40997532417824));
#55451=CARTESIAN_POINT('Ctrl Pts',(108.721168385742,10.8194972414414,6.63019745974499));
#55452=CARTESIAN_POINT('Ctrl Pts',(108.752075532547,10.0402413493614,7.75665046840719));
#55453=CARTESIAN_POINT('Ctrl Pts',(108.782982679352,9.10327904796693,8.72911913751927));
#55454=CARTESIAN_POINT('Ctrl Pts',(108.844226236783,7.246656536744,10.6560987180694));
#55455=CARTESIAN_POINT('Ctrl Pts',(108.905469794214,4.77080353486937,11.9784624269707));
#55456=CARTESIAN_POINT('Ctrl Pts',(108.966713351645,2.13438197832402,12.4317378478958));
#55457=CARTESIAN_POINT('Ctrl Pts',(107.547344722949,1.01347785817195,-11.5532729648613));
#55458=CARTESIAN_POINT('Ctrl Pts',(107.555157200122,1.02853006148911,-11.5649311188494));
#55459=CARTESIAN_POINT('Ctrl Pts',(107.563081485634,1.04337171979055,-11.5767876635257));
#55460=CARTESIAN_POINT('Ctrl Pts',(107.571107356017,1.05800344929602,-11.5888274417128));
#55461=CARTESIAN_POINT('Ctrl Pts',(107.601592993975,1.11358092402132,-11.6345595930381));
#55462=CARTESIAN_POINT('Ctrl Pts',(107.633652536267,1.16633032082653,-11.6830998317929));
#55463=CARTESIAN_POINT('Ctrl Pts',(107.666874561659,1.2163822695299,-11.7338367536604));
#55464=CARTESIAN_POINT('Ctrl Pts',(107.703659888335,1.27180264989783,-11.7900155754933));
#55465=CARTESIAN_POINT('Ctrl Pts',(107.741870440797,1.32391544230277,-11.8488877529446));
#55466=CARTESIAN_POINT('Ctrl Pts',(107.780947707395,1.37283791092559,-11.9095908316944));
#55467=CARTESIAN_POINT('Ctrl Pts',(107.811334718166,1.41088068388255,-11.9567943663416));
#55468=CARTESIAN_POINT('Ctrl Pts',(107.842245816055,1.44699286001964,-12.0051043086855));
#55469=CARTESIAN_POINT('Ctrl Pts',(107.873418383575,1.48121215166239,-12.0541027667175));
#55470=CARTESIAN_POINT('Ctrl Pts',(107.923912309557,1.53664122013029,-12.1334714138957));
#55471=CARTESIAN_POINT('Ctrl Pts',(107.97573271635,1.58784070065421,-12.215649995053));
#55472=CARTESIAN_POINT('Ctrl Pts',(108.028235752821,1.63507762537721,-12.2995995033468));
#55473=CARTESIAN_POINT('Ctrl Pts',(108.068036194817,1.6708860396869,-12.3632382518832));
#55474=CARTESIAN_POINT('Ctrl Pts',(108.108228913152,1.70441636021813,-12.4278934158814));
#55475=CARTESIAN_POINT('Ctrl Pts',(108.14853343171,1.73578194556773,-12.4930929274478));
#55476=CARTESIAN_POINT('Ctrl Pts',(108.477958351107,-1.94818655881014,11.4328396604549));
#55477=CARTESIAN_POINT('Ctrl Pts',(108.53784915696,-4.31949723671962,11.0287619573935));
#55478=CARTESIAN_POINT('Ctrl Pts',(108.627685365739,-7.67204750982751,9.27780206687928));
#55479=CARTESIAN_POINT('Ctrl Pts',(108.747466977445,-10.5120654759104,5.32006485465251));
#55480=CARTESIAN_POINT('Ctrl Pts',(108.86724858915,-12.0211681894647,0.692105791054637));
#55481=CARTESIAN_POINT('Ctrl Pts',(109.016975603782,-11.068234710412,-5.54964839940795));
#55482=CARTESIAN_POINT('Ctrl Pts',(109.166702618414,-6.63827437718498,-10.0475317645548));
#55483=CARTESIAN_POINT('Ctrl Pts',(109.256538827193,-3.17834332867996,-11.2182879948304));
#55484=CARTESIAN_POINT('Ctrl Pts',(109.286484230119,-1.99349831895978,-11.4250259527891));
#55485=CARTESIAN_POINT('Ctrl Pts',(108.673487642273,-2.00507622325195,11.7666939358369));
#55486=CARTESIAN_POINT('Ctrl Pts',(108.733378448126,-4.44563235824741,11.3508166210639));
#55487=CARTESIAN_POINT('Ctrl Pts',(108.823214656905,-7.89608160268274,9.54872634974918));
#55488=CARTESIAN_POINT('Ctrl Pts',(108.94299626861,-10.8190319082629,5.47541789464821));
#55489=CARTESIAN_POINT('Ctrl Pts',(109.062777880316,-12.372202448173,0.712316209832714));
#55490=CARTESIAN_POINT('Ctrl Pts',(109.212504894948,-11.3914420314928,-5.71170558730129));
#55491=CARTESIAN_POINT('Ctrl Pts',(109.362231909579,-6.83212090593912,-10.3409331885453));
#55492=CARTESIAN_POINT('Ctrl Pts',(109.452068118358,-3.27115522322458,-11.545877073377));
#55493=CARTESIAN_POINT('Ctrl Pts',(109.482013521285,-2.05171114766354,-11.7586520574114));
#55494=CARTESIAN_POINT('Ctrl Pts',(108.869016933439,-2.06196588769375,12.1005482112188));
#55495=CARTESIAN_POINT('Ctrl Pts',(108.928907739291,-4.5717674797752,11.6728712847344));
#55496=CARTESIAN_POINT('Ctrl Pts',(109.01874394807,-8.12011569553795,9.81965063261907));
#55497=CARTESIAN_POINT('Ctrl Pts',(109.138525559776,-11.1259983406154,5.63077093464392));
#55498=CARTESIAN_POINT('Ctrl Pts',(109.258307171481,-12.7232367068813,0.732526628610785));
#55499=CARTESIAN_POINT('Ctrl Pts',(109.408034186113,-11.7146493525736,-5.87376277519463));
#55500=CARTESIAN_POINT('Ctrl Pts',(109.557761200745,-7.02596743469325,-10.6343346125358));
#55501=CARTESIAN_POINT('Ctrl Pts',(109.647597409524,-3.3639671177692,-11.8734661519237));
#55502=CARTESIAN_POINT('Ctrl Pts',(109.67754281245,-2.1099239763673,-12.0922781620336));
#55503=CARTESIAN_POINT('Ctrl Pts',(109.064546224604,-2.11885555213556,12.4344024866008));
#55504=CARTESIAN_POINT('Ctrl Pts',(109.124437030457,-4.69790260130299,11.9949259484048));
#55505=CARTESIAN_POINT('Ctrl Pts',(109.214273239236,-8.34414978839318,10.090574915489));
#55506=CARTESIAN_POINT('Ctrl Pts',(109.334054850941,-11.4329647729678,5.78612397463963));
#55507=CARTESIAN_POINT('Ctrl Pts',(109.453836462647,-13.0742709655896,0.752737047388862));
#55508=CARTESIAN_POINT('Ctrl Pts',(109.603563477279,-12.0378566736544,-6.03581996308797));
#55509=CARTESIAN_POINT('Ctrl Pts',(109.75329049191,-7.21981396344739,-10.9277360365263));
#55510=CARTESIAN_POINT('Ctrl Pts',(109.84312670069,-3.45677901231382,-12.2010552304703));
#55511=CARTESIAN_POINT('Ctrl Pts',(109.873072103616,-2.16813680507106,-12.4259042666559));
#55512=CARTESIAN_POINT('',(109.873072103616,-2.16813680507102,-12.4259042666559));
#55513=CARTESIAN_POINT('',(109.281532350295,-2.18912582690727,-11.3891607102353));
#55514=CARTESIAN_POINT('Ctrl Pts',(109.873072103616,-2.16813680507115,-12.4259042666558));
#55515=CARTESIAN_POINT('Ctrl Pts',(109.802888483755,-2.18021332655258,-12.3017367690068));
#55516=CARTESIAN_POINT('Ctrl Pts',(109.732266767812,-2.1888609950872,-12.177170292616));
#55517=CARTESIAN_POINT('Ctrl Pts',(109.661457734895,-2.19407037232472,-12.0527002541065));
#55518=CARTESIAN_POINT('Ctrl Pts',(109.633303673289,-2.19614164941518,-12.0032102810333));
#55519=CARTESIAN_POINT('Ctrl Pts',(109.605119998715,-2.19766992928173,-11.95373538301));
#55520=CARTESIAN_POINT('Ctrl Pts',(109.576922474526,-2.19865677093697,-11.9043059834552));
#55521=CARTESIAN_POINT('Ctrl Pts',(109.510004507875,-2.20099872963269,-11.7870008296852));
#55522=CARTESIAN_POINT('Ctrl Pts',(109.442772533832,-2.20029775063903,-11.6695389907235));
#55523=CARTESIAN_POINT('Ctrl Pts',(109.375440744552,-2.19647822257344,-11.552340529106));
#55524=CARTESIAN_POINT('Ctrl Pts',(109.344152335973,-2.19470332610961,-11.4978795769887));
#55525=CARTESIAN_POINT('Ctrl Pts',(109.312842373612,-2.19225573972214,-11.4434752830729));
#55526=CARTESIAN_POINT('Ctrl Pts',(109.281532350295,-2.18913148123183,-11.3891685808071));
#55527=CARTESIAN_POINT('',(109.065424143392,-2.15665106701421,12.4279028892547));
#55528=CARTESIAN_POINT('Ctrl Pts',(109.065424143392,-2.15665025088522,12.4279009233094));
#55529=CARTESIAN_POINT('Ctrl Pts',(109.125022309649,-4.72164364222117,11.982505130978));
#55530=CARTESIAN_POINT('Ctrl Pts',(109.184620475906,-7.13772412654634,10.716279968349));
#55531=CARTESIAN_POINT('Ctrl Pts',(109.244218642162,-8.96861620690796,8.86735249441881));
#55532=CARTESIAN_POINT('Ctrl Pts',(109.274164045089,-9.88855728068048,7.93834944506434));
#55533=CARTESIAN_POINT('Ctrl Pts',(109.304109448015,-10.6607610268242,6.86223670985195));
#55534=CARTESIAN_POINT('Ctrl Pts',(109.334054850941,-11.2520261739738,5.69500697633937));
#55535=CARTESIAN_POINT('Ctrl Pts',(109.364000253868,-11.8432913211233,4.52777724282685));
#55536=CARTESIAN_POINT('Ctrl Pts',(109.393945656794,-12.2536178692787,3.26943051101414));
#55537=CARTESIAN_POINT('Ctrl Pts',(109.42389105972,-12.4580746152533,1.97796222244055));
#55538=CARTESIAN_POINT('Ctrl Pts',(109.483781865573,-12.8669881072025,-0.60497435470658));
#55539=CARTESIAN_POINT('Ctrl Pts',(109.543672671426,-12.4524223904284,-3.32039715889727));
#55540=CARTESIAN_POINT('Ctrl Pts',(109.603563477279,-11.28153099,-5.65649177568027));
#55541=CARTESIAN_POINT('Ctrl Pts',(109.663454283131,-10.1106395895716,-7.99258639246326));
#55542=CARTESIAN_POINT('Ctrl Pts',(109.723345088984,-8.18342250548884,-9.94935282183856));
#55543=CARTESIAN_POINT('Ctrl Pts',(109.783235894837,-5.86855683251303,-11.1675279400499));
#55544=CARTESIAN_POINT('Ctrl Pts',(109.813181297763,-4.7111239960251,-11.7766154991556));
#55545=CARTESIAN_POINT('Ctrl Pts',(109.84312670069,-3.4567790123139,-12.2010552304703));
#55546=CARTESIAN_POINT('Ctrl Pts',(109.873072103616,-2.16813680507115,-12.4259042666558));
#55547=CARTESIAN_POINT('',(108.477958351107,-1.9481865588103,11.4328396604549));
#55548=CARTESIAN_POINT('Ctrl Pts',(108.477958351107,-1.9481865588103,11.4328396604549));
#55549=CARTESIAN_POINT('Ctrl Pts',(108.478836583785,-1.94864729003221,11.434295047288));
#55550=CARTESIAN_POINT('Ctrl Pts',(108.479714849452,-1.94910728118743,11.4357506492995));
#55551=CARTESIAN_POINT('Ctrl Pts',(108.480593146676,-1.949566532967,11.437206463898));
#55552=CARTESIAN_POINT('Ctrl Pts',(108.538946250772,-1.98007871742698,11.5339291888642));
#55553=CARTESIAN_POINT('Ctrl Pts',(108.597609547501,-2.00742552408462,11.6318734233243));
#55554=CARTESIAN_POINT('Ctrl Pts',(108.656284391412,-2.03178856868386,11.7304879191871));
#55555=CARTESIAN_POINT('Ctrl Pts',(108.695850475067,-2.04821724912794,11.796986424047));
#55556=CARTESIAN_POINT('Ctrl Pts',(108.735421809435,-2.06328990179688,11.8637890556732));
#55557=CARTESIAN_POINT('Ctrl Pts',(108.774906821129,-2.07707374906138,11.9307197670003));
#55558=CARTESIAN_POINT('Ctrl Pts',(108.837124803449,-2.09879346316566,12.0361849456926));
#55559=CARTESIAN_POINT('Ctrl Pts',(108.899470076242,-2.11742830718139,12.1425486267099));
#55560=CARTESIAN_POINT('Ctrl Pts',(108.961695535961,-2.13312920500828,12.249330872859));
#55561=CARTESIAN_POINT('Ctrl Pts',(108.996323035935,-2.14186651030987,12.3087535310842));
#55562=CARTESIAN_POINT('Ctrl Pts',(109.030913432804,-2.14969603440291,12.3683053914907));
#55563=CARTESIAN_POINT('Ctrl Pts',(109.065424143392,-2.15665025088575,12.4279009233093));
#55564=CARTESIAN_POINT('Ctrl Pts',(108.477958351107,-1.94818655881014,11.4328396604549));
#55565=CARTESIAN_POINT('Ctrl Pts',(108.53784915696,-4.31949723671962,11.0287619573935));
#55566=CARTESIAN_POINT('Ctrl Pts',(108.627685365739,-7.67204750982751,9.27780206687928));
#55567=CARTESIAN_POINT('Ctrl Pts',(108.747466977445,-10.5120654759104,5.32006485465251));
#55568=CARTESIAN_POINT('Ctrl Pts',(108.86724858915,-12.0211681894647,0.692105791054637));
#55569=CARTESIAN_POINT('Ctrl Pts',(109.016975603782,-11.068234710412,-5.54964839940795));
#55570=CARTESIAN_POINT('Ctrl Pts',(109.165051991806,-6.687111324995,-9.99794601691013));
#55571=CARTESIAN_POINT('Ctrl Pts',(109.253237573977,-3.30521629928841,-11.1747498326638));
#55572=CARTESIAN_POINT('Ctrl Pts',(109.281532350295,-2.18913148123183,-11.3891685808071));
#55573=CARTESIAN_POINT('Ctrl Pts',(109.38579409552,1.97561503404851,-11.4281319036333));
#55574=CARTESIAN_POINT('Ctrl Pts',(109.416044709093,3.17286165411581,-11.2211603319002));
#55575=CARTESIAN_POINT('Ctrl Pts',(109.506796549814,6.66901151712989,-10.0383350847298));
#55576=CARTESIAN_POINT('Ctrl Pts',(109.658049617681,11.1270467960305,-5.46893215383385));
#55577=CARTESIAN_POINT('Ctrl Pts',(109.809302685548,12.0200961191123,0.853135904503782));
#55578=CARTESIAN_POINT('Ctrl Pts',(109.930305139842,10.4208972763816,5.50447055552805));
#55579=CARTESIAN_POINT('Ctrl Pts',(110.051307594136,7.47576055358735,9.44837079282557));
#55580=CARTESIAN_POINT('Ctrl Pts',(110.142059434856,4.04474488933938,11.1377843017737));
#55581=CARTESIAN_POINT('Ctrl Pts',(110.202560662003,1.63912736726564,11.4812244574993));
#55582=CARTESIAN_POINT('Ctrl Pts',(109.581323386685,2.0333056468109,-11.7618487061923));
#55583=CARTESIAN_POINT('Ctrl Pts',(109.611574000259,3.26551347639981,-11.5488332865476));
#55584=CARTESIAN_POINT('Ctrl Pts',(109.702325840979,6.86375561165841,-10.3314679533159));
#55585=CARTESIAN_POINT('Ctrl Pts',(109.853578908847,11.4519715090114,-5.62863231893341));
#55586=CARTESIAN_POINT('Ctrl Pts',(110.004831976714,12.3710990719262,0.878048618900141));
#55587=CARTESIAN_POINT('Ctrl Pts',(110.125834431008,10.7252014748451,5.66520848969443));
#55588=CARTESIAN_POINT('Ctrl Pts',(110.246836885302,7.69406280365562,9.72427591161154));
#55589=CARTESIAN_POINT('Ctrl Pts',(110.337588726022,4.16285687325936,11.4630225643455));
#55590=CARTESIAN_POINT('Ctrl Pts',(110.398089953169,1.68699208816697,11.8164916339484));
#55591=CARTESIAN_POINT('Ctrl Pts',(109.776852677851,2.09099625957329,-12.0955655087513));
#55592=CARTESIAN_POINT('Ctrl Pts',(109.807103291424,3.3581652986838,-11.876506241195));
#55593=CARTESIAN_POINT('Ctrl Pts',(109.897855132145,7.05849970618694,-10.624600821902));
#55594=CARTESIAN_POINT('Ctrl Pts',(110.049108200012,11.7768962219922,-5.78833248403296));
#55595=CARTESIAN_POINT('Ctrl Pts',(110.200361267879,12.7221020247401,0.902961333296493));
#55596=CARTESIAN_POINT('Ctrl Pts',(110.321363722173,11.0295056733086,5.82594642386081));
#55597=CARTESIAN_POINT('Ctrl Pts',(110.442366176467,7.91236505372388,10.0001810303975));
#55598=CARTESIAN_POINT('Ctrl Pts',(110.533118017188,4.28096885717935,11.7882608269174));
#55599=CARTESIAN_POINT('Ctrl Pts',(110.593619244335,1.73485680906831,12.1517588103975));
#55600=CARTESIAN_POINT('Ctrl Pts',(109.972381969016,2.14868687233568,-12.4292823113103));
#55601=CARTESIAN_POINT('Ctrl Pts',(110.00263258259,3.45081712096779,-12.2041791958424));
#55602=CARTESIAN_POINT('Ctrl Pts',(110.09338442331,7.25324380071547,-10.917733690488));
#55603=CARTESIAN_POINT('Ctrl Pts',(110.244637491178,12.1018209349731,-5.94803264913252));
#55604=CARTESIAN_POINT('Ctrl Pts',(110.395890559045,13.073104977554,0.927874047692852));
#55605=CARTESIAN_POINT('Ctrl Pts',(110.516893013339,11.333809871772,5.98668435802718));
#55606=CARTESIAN_POINT('Ctrl Pts',(110.637895467633,8.13066730379214,10.2760861491835));
#55607=CARTESIAN_POINT('Ctrl Pts',(110.728647308353,4.39908084109933,12.1134990894893));
#55608=CARTESIAN_POINT('Ctrl Pts',(110.7891485355,1.78272152996964,12.4870259868466));
#55609=CARTESIAN_POINT('',(109.391405608182,2.19731819681764,-11.3875829881294));
#55610=CARTESIAN_POINT('',(109.972381969016,2.14868687233581,-12.4292823113103));
#55611=CARTESIAN_POINT('Ctrl Pts',(109.391405608182,2.1973257056837,-11.3875934426363));
#55612=CARTESIAN_POINT('Ctrl Pts',(109.392396565347,2.19737466243356,-11.3893444745));
#55613=CARTESIAN_POINT('Ctrl Pts',(109.39338746931,2.19742294454714,-11.3910955560154));
#55614=CARTESIAN_POINT('Ctrl Pts',(109.394378319473,2.19747055234629,-11.3928466858768));
#55615=CARTESIAN_POINT('Ctrl Pts',(109.461338464392,2.20068781490421,-11.51118537485));
#55616=CARTESIAN_POINT('Ctrl Pts',(109.528177183617,2.20083641292418,-11.6299636424174));
#55617=CARTESIAN_POINT('Ctrl Pts',(109.594689085937,2.19796783634277,-11.7487490106668));
#55618=CARTESIAN_POINT('Ctrl Pts',(109.624936761945,2.19666329126121,-11.8027691365074));
#55619=CARTESIAN_POINT('Ctrl Pts',(109.655116846808,2.19473541263824,-11.8567905206786));
#55620=CARTESIAN_POINT('Ctrl Pts',(109.685210022632,2.19219250554556,-11.9107715248805));
#55621=CARTESIAN_POINT('Ctrl Pts',(109.755294163322,2.18627031709048,-12.036488142997));
#55622=CARTESIAN_POINT('Ctrl Pts',(109.825179300418,2.17698401578315,-12.1624758836485));
#55623=CARTESIAN_POINT('Ctrl Pts',(109.894618363154,2.16432091039785,-12.2882242713375));
#55624=CARTESIAN_POINT('Ctrl Pts',(109.920606362969,2.15958166468455,-12.3352863851853));
#55625=CARTESIAN_POINT('Ctrl Pts',(109.946531882172,2.15436993164035,-12.3823148221297));
#55626=CARTESIAN_POINT('Ctrl Pts',(109.972381969016,2.14868687233568,-12.4292823113103));
#55627=CARTESIAN_POINT('',(110.191221970063,2.08852238929011,11.4078504030635));
#55628=CARTESIAN_POINT('Ctrl Pts',(109.391405608182,2.19732570568378,-11.3875934426363));
#55629=CARTESIAN_POINT('Ctrl Pts',(109.419785717535,3.31663241499189,-11.1717392207365));
#55630=CARTESIAN_POINT('Ctrl Pts',(109.508667054035,6.72414278767814,-9.98182656169961));
#55631=CARTESIAN_POINT('Ctrl Pts',(109.658049617681,11.1270467960305,-5.46893215383385));
#55632=CARTESIAN_POINT('Ctrl Pts',(109.809302685548,12.0200961191123,0.853135904503782));
#55633=CARTESIAN_POINT('Ctrl Pts',(109.930305139842,10.4208972763816,5.50447055552805));
#55634=CARTESIAN_POINT('Ctrl Pts',(110.047528030156,7.56775317257574,9.32518136360488));
#55635=CARTESIAN_POINT('Ctrl Pts',(110.134500306896,4.32840974362946,10.9948652468278));
#55636=CARTESIAN_POINT('Ctrl Pts',(110.191221970063,2.0884820668001,11.4077475491063));
#55637=CARTESIAN_POINT('',(110.7891485355,1.78272152996986,12.4870259868466));
#55638=CARTESIAN_POINT('Ctrl Pts',(110.7891485355,1.78272152996991,12.4870259868466));
#55639=CARTESIAN_POINT('Ctrl Pts',(110.73086285581,1.82486995155475,12.3813009097418));
#55640=CARTESIAN_POINT('Ctrl Pts',(110.671639795078,1.86334704785855,12.2739780744279));
#55641=CARTESIAN_POINT('Ctrl Pts',(110.611907449059,1.89832348357942,12.1658919835167));
#55642=CARTESIAN_POINT('Ctrl Pts',(110.571370896696,1.92205977074311,12.092540813239));
#55643=CARTESIAN_POINT('Ctrl Pts',(110.530599794242,1.94418497331027,12.0188377356399));
#55644=CARTESIAN_POINT('Ctrl Pts',(110.489727940626,1.96476502139403,11.94503854261));
#55645=CARTESIAN_POINT('Ctrl Pts',(110.424075796662,1.9978225942717,11.8264954667157));
#55646=CARTESIAN_POINT('Ctrl Pts',(110.357675707854,2.02713460334668,11.7068242062579));
#55647=CARTESIAN_POINT('Ctrl Pts',(110.290889857939,2.05284419609184,11.5867407952597));
#55648=CARTESIAN_POINT('Ctrl Pts',(110.257747473351,2.06560254552451,11.5271495705457));
#55649=CARTESIAN_POINT('Ctrl Pts',(110.224510090202,2.07747454356665,11.4674565629599));
#55650=CARTESIAN_POINT('Ctrl Pts',(110.191221970063,2.08848206680026,11.4077475491063));
#55651=CARTESIAN_POINT('Ctrl Pts',(109.972381969016,2.14868687233568,-12.4292823113103));
#55652=CARTESIAN_POINT('Ctrl Pts',(110.00263258259,3.45081712096779,-12.2041791958424));
#55653=CARTESIAN_POINT('Ctrl Pts',(110.032883196163,4.71829268088368,-11.7753640273909));
#55654=CARTESIAN_POINT('Ctrl Pts',(110.063133809737,5.88651486311146,-11.1581738456663));
#55655=CARTESIAN_POINT('Ctrl Pts',(110.123635036884,8.22295922756701,-9.92379348221692));
#55656=CARTESIAN_POINT('Ctrl Pts',(110.184136264031,10.1623900812701,-7.93591306567471));
#55657=CARTESIAN_POINT('Ctrl Pts',(110.244637491178,11.3263623166378,-5.56679151803852));
#55658=CARTESIAN_POINT('Ctrl Pts',(110.305138718325,12.4903345520055,-3.19766997040239));
#55659=CARTESIAN_POINT('Ctrl Pts',(110.365639945472,12.8788481690378,-0.447307291672291));
#55660=CARTESIAN_POINT('Ctrl Pts',(110.426141172618,12.428587672788,2.15575037134916));
#55661=CARTESIAN_POINT('Ctrl Pts',(110.456391786192,12.203457424663,3.45727920285992));
#55662=CARTESIAN_POINT('Ctrl Pts',(110.486642399765,11.7686336482176,4.72198178044351));
#55663=CARTESIAN_POINT('Ctrl Pts',(110.516893013339,11.1508289389973,5.89050829312984));
#55664=CARTESIAN_POINT('Ctrl Pts',(110.547143626912,10.5330242297771,7.05903480581618));
#55665=CARTESIAN_POINT('Ctrl Pts',(110.577394240486,9.73223858778215,8.13138525360525));
#55666=CARTESIAN_POINT('Ctrl Pts',(110.607644854059,8.78376077504186,9.05044254549862));
#55667=CARTESIAN_POINT('Ctrl Pts',(110.668146081206,6.88680514956126,10.8885571292854));
#55668=CARTESIAN_POINT('Ctrl Pts',(110.728647308353,4.39908084109936,12.1134990894893));
#55669=CARTESIAN_POINT('Ctrl Pts',(110.7891485355,1.78272152996964,12.4870259868466));
#55670=CARTESIAN_POINT('Ctrl Pts',(111.097169771268,-0.290214146636271,
12.6103009400526));
#55671=CARTESIAN_POINT('Ctrl Pts',(111.144815151789,-2.37096670930334,12.5624143882402));
#55672=CARTESIAN_POINT('Ctrl Pts',(111.240105912831,-6.50629452391662,11.4165924521908));
#55673=CARTESIAN_POINT('Ctrl Pts',(111.383042054393,-11.1491329074663,6.95494094815187));
#55674=CARTESIAN_POINT('Ctrl Pts',(111.525978195955,-13.1145440767032,0.824063538448764));
#55675=CARTESIAN_POINT('Ctrl Pts',(111.668914337517,-11.9318640492024,-5.5049451877202));
#55676=CARTESIAN_POINT('Ctrl Pts',(111.811850479079,-7.88447155714136,-10.5122325482705));
#55677=CARTESIAN_POINT('Ctrl Pts',(111.954786620641,-1.94430045531652,-12.9958610226402));
#55678=CARTESIAN_POINT('Ctrl Pts',(112.097722762203,4.4626861392344,-12.3594863000869));
#55679=CARTESIAN_POINT('Ctrl Pts',(112.240658903765,9.79827742810367,-8.75592671286024));
#55680=CARTESIAN_POINT('Ctrl Pts',(112.383595045327,12.7815601968128,-3.05028594329674));
#55681=CARTESIAN_POINT('Ctrl Pts',(112.526531186889,12.696311862802,3.38764795390582));
#55682=CARTESIAN_POINT('Ctrl Pts',(112.669467328451,9.56300415581823,9.01229516996203));
#55683=CARTESIAN_POINT('Ctrl Pts',(112.812403470013,4.13386177705519,12.4733191545619));
#55684=CARTESIAN_POINT('Ctrl Pts',(112.955339611575,-2.28771515821232,12.9398170902243));
#55685=CARTESIAN_POINT('Ctrl Pts',(113.098275753138,-8.16007012053368,10.2997942704675));
#55686=CARTESIAN_POINT('Ctrl Pts',(113.2412118947,-12.0733999250621,5.18705315684538));
#55687=CARTESIAN_POINT('Ctrl Pts',(113.384148036262,-13.0882138535401,-1.1709673804415));
#55688=CARTESIAN_POINT('Ctrl Pts',(113.527084177824,-10.9608808597989,-7.24786845005694));
#55689=CARTESIAN_POINT('Ctrl Pts',(113.670020319386,-6.20211945919366,-11.5847408517043));
#55690=CARTESIAN_POINT('Ctrl Pts',(113.812956460948,0.0456129136003346,
-13.1404119346645));
#55691=CARTESIAN_POINT('Ctrl Pts',(113.95589260251,6.28239478521566,-11.5414046858392));
#55692=CARTESIAN_POINT('Ctrl Pts',(114.098828744072,11.0109336279624,-7.1716000307795));
#55693=CARTESIAN_POINT('Ctrl Pts',(114.241764885634,13.0960276590931,-1.08007680700643));
#55694=CARTESIAN_POINT('Ctrl Pts',(114.384701027196,12.0370988918816,5.27074535791014));
#55695=CARTESIAN_POINT('Ctrl Pts',(114.527637168758,8.08836916076015,10.3561957628697));
#55696=CARTESIAN_POINT('Ctrl Pts',(114.67057331032,2.19782793558771,12.9553872468603));
#55697=CARTESIAN_POINT('Ctrl Pts',(114.813509451882,-4.22035581903552,12.4443201159399));
#55698=CARTESIAN_POINT('Ctrl Pts',(114.956445593445,-9.62533959369969,8.945688570367));
#55699=CARTESIAN_POINT('Ctrl Pts',(115.099381735007,-12.7195244136438,3.29942497607923));
#55700=CARTESIAN_POINT('Ctrl Pts',(115.242317876569,-12.7600752611215,-3.1389465642066));
#55701=CARTESIAN_POINT('Ctrl Pts',(115.385254018131,-9.73725696256094,-8.82373691986794));
#55702=CARTESIAN_POINT('Ctrl Pts',(115.528190159693,-4.37677111438902,-12.3901727827269));
#55703=CARTESIAN_POINT('Ctrl Pts',(115.671126301255,2.03446587665453,-12.982043464728));
#55704=CARTESIAN_POINT('Ctrl Pts',(115.814062442817,7.95727976006216,-10.4572564057129));
#55705=CARTESIAN_POINT('Ctrl Pts',(115.956998584379,11.9697526294507,-5.42194758061048));
#55706=CARTESIAN_POINT('Ctrl Pts',(116.099934725941,13.1085942544627,0.915031186620946));
#55707=CARTESIAN_POINT('Ctrl Pts',(116.242870867503,11.1003927484593,7.03233773286076));
#55708=CARTESIAN_POINT('Ctrl Pts',(116.385807009065,6.42727687176741,11.4613516302832));
#55709=CARTESIAN_POINT('Ctrl Pts',(116.528743150627,0.211119866039206,13.1388026997321));
#55710=CARTESIAN_POINT('Ctrl Pts',(116.671679292189,-6.05568826983115,11.6619279908134));
#55711=CARTESIAN_POINT('Ctrl Pts',(116.814615433752,-10.8687510776711,7.38539445257166));
#55712=CARTESIAN_POINT('Ctrl Pts',(116.957551575314,-13.0723504975697,1.33566445033233));
#55713=CARTESIAN_POINT('Ctrl Pts',(117.100487716876,-12.1379349596952,-5.03437216491156));
#55714=CARTESIAN_POINT('Ctrl Pts',(117.243423858438,-8.28879524507787,-10.1963878425912));
#55715=CARTESIAN_POINT('Ctrl Pts',(117.338714619479,-4.39706681368208,-12.0042301641757));
#55716=CARTESIAN_POINT('Ctrl Pts',(117.38636,-2.35227454062139,-12.3923653325402));
#55717=CARTESIAN_POINT('Ctrl Pts',(111.292699062434,-0.282422116923941,
12.2717239246129));
#55718=CARTESIAN_POINT('Ctrl Pts',(111.340344442955,-2.30730805151564,12.2251230903951));
#55719=CARTESIAN_POINT('Ctrl Pts',(111.435635203996,-6.33160545091578,11.1100656042329));
#55720=CARTESIAN_POINT('Ctrl Pts',(111.578571345558,-10.8497871454186,6.76820605895459));
#55721=CARTESIAN_POINT('Ctrl Pts',(111.72150748712,-12.7624285155083,0.801938057486237));
#55722=CARTESIAN_POINT('Ctrl Pts',(111.864443628682,-11.6115025496937,-5.3571415848817));
#55723=CARTESIAN_POINT('Ctrl Pts',(112.007379770244,-7.6727794761334,-10.229987077784));
#55724=CARTESIAN_POINT('Ctrl Pts',(112.150315911806,-1.89209746282579,-12.6469320114269));
#55725=CARTESIAN_POINT('Ctrl Pts',(112.293252053368,4.34286640130357,-12.0276434674896));
#55726=CARTESIAN_POINT('Ctrl Pts',(112.436188194931,9.53520111106505,-8.52083672191218));
#55727=CARTESIAN_POINT('Ctrl Pts',(112.579124336493,12.4383850002277,-2.96838807933386));
#55728=CARTESIAN_POINT('Ctrl Pts',(112.722060478055,12.355425519325,3.29669217584419));
#55729=CARTESIAN_POINT('Ctrl Pts',(112.864996619617,9.30624474768778,8.770321880394));
#55730=CARTESIAN_POINT('Ctrl Pts',(113.007932761179,4.0228707238385,12.1384199961632));
#55731=CARTESIAN_POINT('Ctrl Pts',(113.150868902741,-2.22629174142586,12.5923928160875));
#55732=CARTESIAN_POINT('Ctrl Pts',(113.293805044303,-7.9409784271377,10.0232526066075));
#55733=CARTESIAN_POINT('Ctrl Pts',(113.436741185865,-11.7492382946403,5.04778471391757));
#55734=CARTESIAN_POINT('Ctrl Pts',(113.579677327427,-12.7368052388659,-1.13952779444496));
#55735=CARTESIAN_POINT('Ctrl Pts',(113.722613468989,-10.6665895224436,-7.05326867961644));
#55736=CARTESIAN_POINT('Ctrl Pts',(113.865549610551,-6.03559725596654,-11.2736993467585));
#55737=CARTESIAN_POINT('Ctrl Pts',(114.008485752114,0.0443882414671669,
-12.7876018411039));
#55738=CARTESIAN_POINT('Ctrl Pts',(114.151421893675,6.11371725037299,-11.2315267240768));
#55739=CARTESIAN_POINT('Ctrl Pts',(114.294358035238,10.7152984117464,-6.97904800954766));
#55740=CARTESIAN_POINT('Ctrl Pts',(114.4372941768,12.7444092496665,-1.05107756396691));
#55741=CARTESIAN_POINT('Ctrl Pts',(114.580230318362,11.7139119166666,5.12922984286356));
#55742=CARTESIAN_POINT('Ctrl Pts',(114.723166459924,7.87120258374953,10.0781397617187));
#55743=CARTESIAN_POINT('Ctrl Pts',(114.866102601486,2.13881792255004,12.6075449258277));
#55744=CARTESIAN_POINT('Ctrl Pts',(115.009038743048,-4.10704246639664,12.1101995597327));
#55745=CARTESIAN_POINT('Ctrl Pts',(115.15197488461,-9.36690652634302,8.70550361747755));
#55746=CARTESIAN_POINT('Ctrl Pts',(115.294911026172,-12.3780148307832,3.21083791805588));
#55747=CARTESIAN_POINT('Ctrl Pts',(115.437847167734,-12.4174769187636,-3.05466822982062));
#55748=CARTESIAN_POINT('Ctrl Pts',(115.580783309296,-9.47581899873865,-8.58682627629518));
#55749=CARTESIAN_POINT('Ctrl Pts',(115.723719450858,-4.25925812970948,-12.0575060413461));
#55750=CARTESIAN_POINT('Ctrl Pts',(115.86665559242,1.97984201099058,-12.6334854444642));
#55751=CARTESIAN_POINT('Ctrl Pts',(116.009591733983,7.74363283403016,-10.1764870029551));
#55752=CARTESIAN_POINT('Ctrl Pts',(116.152527875545,11.6483738503004,-5.2763724005699));
#55753=CARTESIAN_POINT('Ctrl Pts',(116.295464017107,12.7566384414821,0.890463293303174));
#55754=CARTESIAN_POINT('Ctrl Pts',(116.438400158669,10.802355622712,6.84352479869885));
#55755=CARTESIAN_POINT('Ctrl Pts',(116.581336300231,6.25470936279257,11.1536230323429));
#55756=CARTESIAN_POINT('Ctrl Pts',(116.724272441793,0.205451457768569,12.7860358129088));
#55757=CARTESIAN_POINT('Ctrl Pts',(116.867208583355,-5.89309763297169,11.3488140697284));
#55758=CARTESIAN_POINT('Ctrl Pts',(117.010144724917,-10.5769333550863,7.18710221327586));
#55759=CARTESIAN_POINT('Ctrl Pts',(117.153080866479,-12.7213678019711,1.29980287293045));
#55760=CARTESIAN_POINT('Ctrl Pts',(117.296017008041,-11.8120406125427,-4.89920309081004));
#55761=CARTESIAN_POINT('Ctrl Pts',(117.438953149603,-8.06624737972471,-9.92262256288682));
#55762=CARTESIAN_POINT('Ctrl Pts',(117.534243910645,-4.27900890487063,-11.681925689369));
#55763=CARTESIAN_POINT('Ctrl Pts',(117.581889291165,-2.28911775338493,-12.05963972286));
#55764=CARTESIAN_POINT('Ctrl Pts',(111.4882283536,-0.27463008721161,11.9331469091732));
#55765=CARTESIAN_POINT('Ctrl Pts',(111.53587373412,-2.24364939372795,11.8878317925501));
#55766=CARTESIAN_POINT('Ctrl Pts',(111.631164495162,-6.15691637791494,10.8035387562751));
#55767=CARTESIAN_POINT('Ctrl Pts',(111.774100636724,-10.5504413833709,6.58147116975733));
#55768=CARTESIAN_POINT('Ctrl Pts',(111.917036778286,-12.4103129543134,0.779812576523712));
#55769=CARTESIAN_POINT('Ctrl Pts',(112.059972919848,-11.2911410501849,-5.20933798204321));
#55770=CARTESIAN_POINT('Ctrl Pts',(112.20290906141,-7.46108739512543,-9.94774160729745));
#55771=CARTESIAN_POINT('Ctrl Pts',(112.345845202972,-1.83989447033507,-12.2980030002136));
#55772=CARTESIAN_POINT('Ctrl Pts',(112.488781344534,4.22304666337274,-11.6958006348923));
#55773=CARTESIAN_POINT('Ctrl Pts',(112.631717486096,9.27212479402644,-8.28574673096412));
#55774=CARTESIAN_POINT('Ctrl Pts',(112.774653627658,12.0952098036425,-2.88649021537098));
#55775=CARTESIAN_POINT('Ctrl Pts',(112.91758976922,12.0145391758479,3.20573639778256));
#55776=CARTESIAN_POINT('Ctrl Pts',(113.060525910782,9.04948533955733,8.52834859082596));
#55777=CARTESIAN_POINT('Ctrl Pts',(113.203462052344,3.9118796706218,11.8035208377644));
#55778=CARTESIAN_POINT('Ctrl Pts',(113.346398193907,-2.1648683246394,12.2449685419508));
#55779=CARTESIAN_POINT('Ctrl Pts',(113.489334335469,-7.72188673374172,9.74671094274739));
#55780=CARTESIAN_POINT('Ctrl Pts',(113.632270477031,-11.4250766642184,4.90851627098979));
#55781=CARTESIAN_POINT('Ctrl Pts',(113.775206618593,-12.3853966241917,-1.10808820844843));
#55782=CARTESIAN_POINT('Ctrl Pts',(113.918142760155,-10.3722981850883,-6.85866890917593));
#55783=CARTESIAN_POINT('Ctrl Pts',(114.061078901717,-5.86907505273941,-10.9626578418128));
#55784=CARTESIAN_POINT('Ctrl Pts',(114.204015043279,0.0431635693339993,
-12.4347917475433));
#55785=CARTESIAN_POINT('Ctrl Pts',(114.346951184841,5.94503971553032,-10.9216487623144));
#55786=CARTESIAN_POINT('Ctrl Pts',(114.489887326403,10.4196631955305,-6.78649598831582));
#55787=CARTESIAN_POINT('Ctrl Pts',(114.632823467965,12.3927908402399,-1.02207832092739));
#55788=CARTESIAN_POINT('Ctrl Pts',(114.775759609527,11.3907249414516,4.98771432781699));
#55789=CARTESIAN_POINT('Ctrl Pts',(114.918695751089,7.65403600673891,9.80008376056765));
#55790=CARTESIAN_POINT('Ctrl Pts',(115.061631892651,2.07980790951236,12.259702604795));
#55791=CARTESIAN_POINT('Ctrl Pts',(115.204568034214,-3.99372911375776,11.7760790035254));
#55792=CARTESIAN_POINT('Ctrl Pts',(115.347504175776,-9.10847345898634,8.4653186645881));
#55793=CARTESIAN_POINT('Ctrl Pts',(115.490440317338,-12.0365052479226,3.12225086003253));
#55794=CARTESIAN_POINT('Ctrl Pts',(115.6333764589,-12.0748785764056,-2.97038989543463));
#55795=CARTESIAN_POINT('Ctrl Pts',(115.776312600462,-9.21438103491635,-8.34991563272242));
#55796=CARTESIAN_POINT('Ctrl Pts',(115.919248742024,-4.14174514502994,-11.7248392999654));
#55797=CARTESIAN_POINT('Ctrl Pts',(116.062184883586,1.92521814532663,-12.2849274242003));
#55798=CARTESIAN_POINT('Ctrl Pts',(116.205121025148,7.52998590799816,-9.89571760019732));
#55799=CARTESIAN_POINT('Ctrl Pts',(116.34805716671,11.3269950711502,-5.13079722052934));
#55800=CARTESIAN_POINT('Ctrl Pts',(116.490993308272,12.4046826285015,0.865895399985405));
#55801=CARTESIAN_POINT('Ctrl Pts',(116.633929449834,10.5043184969647,6.65471186453694));
#55802=CARTESIAN_POINT('Ctrl Pts',(116.776865591396,6.08214185381772,10.8458944344027));
#55803=CARTESIAN_POINT('Ctrl Pts',(116.919801732959,0.199783049497946,12.4332689260855));
#55804=CARTESIAN_POINT('Ctrl Pts',(117.062737874521,-5.73050699611223,11.0357001486433));
#55805=CARTESIAN_POINT('Ctrl Pts',(117.205674016083,-10.2851156325015,6.98880997398006));
#55806=CARTESIAN_POINT('Ctrl Pts',(117.348610157645,-12.3703851063725,1.26394129552858));
#55807=CARTESIAN_POINT('Ctrl Pts',(117.491546299207,-11.4861462653902,-4.76403401670852));
#55808=CARTESIAN_POINT('Ctrl Pts',(117.634482440769,-7.84369951437156,-9.64885728318242));
#55809=CARTESIAN_POINT('Ctrl Pts',(117.72977320181,-4.16095099605918,-11.3596212145623));
#55810=CARTESIAN_POINT('Ctrl Pts',(117.777418582331,-2.22596096614847,-11.7269141131798));
#55811=CARTESIAN_POINT('Ctrl Pts',(111.683757644765,-0.266838057499279,
11.5945698937334));
#55812=CARTESIAN_POINT('Ctrl Pts',(111.731403025286,-2.17999073594025,11.550540494705));
#55813=CARTESIAN_POINT('Ctrl Pts',(111.826693786327,-5.98222730491411,10.4970119083172));
#55814=CARTESIAN_POINT('Ctrl Pts',(111.969629927889,-10.2510956213232,6.39473628056006));
#55815=CARTESIAN_POINT('Ctrl Pts',(112.112566069451,-12.0581973931186,0.757687095561184));
#55816=CARTESIAN_POINT('Ctrl Pts',(112.255502211013,-10.9707795506762,-5.06153437920471));
#55817=CARTESIAN_POINT('Ctrl Pts',(112.398438352575,-7.24939531411746,-9.66549613681094));
#55818=CARTESIAN_POINT('Ctrl Pts',(112.541374494138,-1.78769147784434,-11.9490739890003));
#55819=CARTESIAN_POINT('Ctrl Pts',(112.6843106357,4.1032269254419,-11.363957802295));
#55820=CARTESIAN_POINT('Ctrl Pts',(112.827246777262,9.00904847698782,-8.05065674001605));
#55821=CARTESIAN_POINT('Ctrl Pts',(112.970182918824,11.7520346070574,-2.80459235140811));
#55822=CARTESIAN_POINT('Ctrl Pts',(113.113119060386,11.6736528323709,3.11478061972093));
#55823=CARTESIAN_POINT('Ctrl Pts',(113.256055201948,8.79272593142687,8.28637530125792));
#55824=CARTESIAN_POINT('Ctrl Pts',(113.39899134351,3.80088861740511,11.4686216793657));
#55825=CARTESIAN_POINT('Ctrl Pts',(113.541927485072,-2.10344490785294,11.897544267814));
#55826=CARTESIAN_POINT('Ctrl Pts',(113.684863626634,-7.50279504034574,9.47016927888733));
#55827=CARTESIAN_POINT('Ctrl Pts',(113.827799768196,-11.1009150337966,4.76924782806198));
#55828=CARTESIAN_POINT('Ctrl Pts',(113.970735909758,-12.0339880095176,-1.07664862245189));
#55829=CARTESIAN_POINT('Ctrl Pts',(114.11367205132,-10.078006847733,-6.66406913873543));
#55830=CARTESIAN_POINT('Ctrl Pts',(114.256608192883,-5.7025528495123,-10.6516163368671));
#55831=CARTESIAN_POINT('Ctrl Pts',(114.399544334445,0.0419388972008348,
-12.0819816539827));
#55832=CARTESIAN_POINT('Ctrl Pts',(114.542480476007,5.77636218068765,-10.6117708005521));
#55833=CARTESIAN_POINT('Ctrl Pts',(114.685416617569,10.1240279793146,-6.59394396708397));
#55834=CARTESIAN_POINT('Ctrl Pts',(114.828352759131,12.0411724308134,-0.993079077887869));
#55835=CARTESIAN_POINT('Ctrl Pts',(114.971288900693,11.0675379662367,4.84619881277042));
#55836=CARTESIAN_POINT('Ctrl Pts',(115.114225042255,7.43686942972829,9.52202775941664));
#55837=CARTESIAN_POINT('Ctrl Pts',(115.257161183817,2.02079789647468,11.9118602837624));
#55838=CARTESIAN_POINT('Ctrl Pts',(115.400097325379,-3.88041576111888,11.4419584473181));
#55839=CARTESIAN_POINT('Ctrl Pts',(115.543033466941,-8.85004039162967,8.22513371169866));
#55840=CARTESIAN_POINT('Ctrl Pts',(115.685969608503,-11.694995665062,3.03366380200918));
#55841=CARTESIAN_POINT('Ctrl Pts',(115.828905750065,-11.7322802340477,-2.88611156104865));
#55842=CARTESIAN_POINT('Ctrl Pts',(115.971841891627,-8.95294307109407,-8.11300498914965));
#55843=CARTESIAN_POINT('Ctrl Pts',(116.11477803319,-4.0242321603504,-11.3921725585846));
#55844=CARTESIAN_POINT('Ctrl Pts',(116.257714174752,1.87059427966267,-11.9363694039364));
#55845=CARTESIAN_POINT('Ctrl Pts',(116.400650316314,7.31633898196617,-9.61494819743955));
#55846=CARTESIAN_POINT('Ctrl Pts',(116.543586457876,11.005616292,-4.98522204048877));
#55847=CARTESIAN_POINT('Ctrl Pts',(116.686522599438,12.0527268155209,0.841327506667632));
#55848=CARTESIAN_POINT('Ctrl Pts',(116.829458741,10.2062813712173,6.46589893037503));
#55849=CARTESIAN_POINT('Ctrl Pts',(116.972394882562,5.9095743448429,10.5381658364625));
#55850=CARTESIAN_POINT('Ctrl Pts',(117.115331024124,0.194114641227306,12.0805020392623));
#55851=CARTESIAN_POINT('Ctrl Pts',(117.258267165686,-5.56791635925277,10.7225862275582));
#55852=CARTESIAN_POINT('Ctrl Pts',(117.401203307248,-9.99329790991669,6.79051773468426));
#55853=CARTESIAN_POINT('Ctrl Pts',(117.54413944881,-12.0194024107739,1.2280797181267));
#55854=CARTESIAN_POINT('Ctrl Pts',(117.687075590372,-11.1602519182376,-4.628864942607));
#55855=CARTESIAN_POINT('Ctrl Pts',(117.830011731934,-7.6211516490184,-9.375092003478));
#55856=CARTESIAN_POINT('Ctrl Pts',(117.925302492976,-4.04289308724772,-11.0373167397556));
#55857=CARTESIAN_POINT('Ctrl Pts',(117.972947873497,-2.16280417891201,-11.3941885034995));
#55858=CARTESIAN_POINT('',(115.665029240284,1.6893531453192,-12.5));
#55859=CARTESIAN_POINT('',(115.587450486329,-1.68935314531919,-12.5));
#55860=CARTESIAN_POINT('Ctrl Pts',(115.665029240284,1.68957794637807,-12.5009920189267));
#55861=CARTESIAN_POINT('Ctrl Pts',(115.665531145448,1.68039383998756,-12.5009881210131));
#55862=CARTESIAN_POINT('Ctrl Pts',(115.666027316753,1.67120940348572,-12.5009840718973));
#55863=CARTESIAN_POINT('Ctrl Pts',(115.666517749822,1.66202462200871,-12.5009798762235));
#55864=CARTESIAN_POINT('Ctrl Pts',(115.679790027354,1.41346273549435,-12.5008663313784));
#55865=CARTESIAN_POINT('Ctrl Pts',(115.688841785677,1.16498141737867,-12.5006475672998));
#55866=CARTESIAN_POINT('Ctrl Pts',(115.693621337552,0.91627655910125,-12.5004053081459));
#55867=CARTESIAN_POINT('Ctrl Pts',(115.695698464643,0.808192870062367,-12.5003000256707));
#55868=CARTESIAN_POINT('Ctrl Pts',(115.69696872091,0.700066299056772,-12.5001901057846));
#55869=CARTESIAN_POINT('Ctrl Pts',(115.697427863959,0.591869115320174,-12.5000810369122));
#55870=CARTESIAN_POINT('Ctrl Pts',(115.698180844966,0.414428937293237,-12.4999021671905));
#55871=CARTESIAN_POINT('Ctrl Pts',(115.696751289823,0.237059544937474,-12.4997260835975));
#55872=CARTESIAN_POINT('Ctrl Pts',(115.693139682215,0.059641091855054,-12.499571625275));
#55873=CARTESIAN_POINT('Ctrl Pts',(115.692870383431,0.0464119211050218,
-12.4995601081217));
#55874=CARTESIAN_POINT('Ctrl Pts',(115.692588963242,0.0331829986088157,
-12.4995487085824));
#55875=CARTESIAN_POINT('Ctrl Pts',(115.692295424718,0.0199542748338118,
-12.4995374329471));
#55876=CARTESIAN_POINT('Ctrl Pts',(115.692214772672,0.0163195776711995,
-12.4995343348766));
#55877=CARTESIAN_POINT('Ctrl Pts',(115.692133205866,0.0126848989764344,
-12.4995312461615));
#55878=CARTESIAN_POINT('Ctrl Pts',(115.692050724368,0.00905023766942509,
-12.4995281669295));
#55879=CARTESIAN_POINT('Ctrl Pts',(115.692002271107,0.0069150776746254,
-12.4995263580531));
#55880=CARTESIAN_POINT('Ctrl Pts',(115.691953502204,0.00477992410763924,
-12.4995245524496));
#55881=CARTESIAN_POINT('Ctrl Pts',(115.691904417675,0.00264477680910505,
-12.4995227501446));
#55882=CARTESIAN_POINT('Ctrl Pts',(115.691862039437,0.000801349139794612,
-12.4995211940839));
#55883=CARTESIAN_POINT('Ctrl Pts',(115.691819425932,-0.0010420736832491,
-12.4995196404822));
#55884=CARTESIAN_POINT('Ctrl Pts',(115.691776577169,-0.0028854917766748,
-12.4995180893558));
#55885=CARTESIAN_POINT('Ctrl Pts',(115.691724393489,-0.00513051196352565,
-12.4995162003052));
#55886=CARTESIAN_POINT('Ctrl Pts',(115.691671860888,-0.00737552484080946,
-12.4995143149263));
#55887=CARTESIAN_POINT('Ctrl Pts',(115.691618979382,-0.00962053064940818,
-12.4995124332486));
#55888=CARTESIAN_POINT('Ctrl Pts',(115.691519210876,-0.0138560543912522,
-12.4995088831952));
#55889=CARTESIAN_POINT('Ctrl Pts',(115.691418200514,-0.0180915511691172,
-12.4995053463176));
#55890=CARTESIAN_POINT('Ctrl Pts',(115.691315948412,-0.0223270226677909,
-12.4995018228123));
#55891=CARTESIAN_POINT('Ctrl Pts',(115.690733516431,-0.0464524345272299,
-12.4994817527879));
#55892=CARTESIAN_POINT('Ctrl Pts',(115.690110802628,-0.070576768109223,
-12.4994621170303));
#55893=CARTESIAN_POINT('Ctrl Pts',(115.689447831599,-0.0947003228280837,
-12.4994429504498));
#55894=CARTESIAN_POINT('Ctrl Pts',(115.688600178345,-0.125543917413364,
-12.4994184446818));
#55895=CARTESIAN_POINT('Ctrl Pts',(115.687686737434,-0.156385429448937,
-12.4993947067422));
#55896=CARTESIAN_POINT('Ctrl Pts',(115.686707570708,-0.187225482320612,
-12.4993718038707));
#55897=CARTESIAN_POINT('Ctrl Pts',(115.681885774495,-0.339093847577508,
-12.4992590212612));
#55898=CARTESIAN_POINT('Ctrl Pts',(115.675472190412,-0.490862634991197,
-12.499166833351));
#55899=CARTESIAN_POINT('Ctrl Pts',(115.667478315592,-0.642604728235641,
-12.4991009813609));
#55900=CARTESIAN_POINT('Ctrl Pts',(115.654842096987,-0.882469162560806,
-12.4989968866432));
#55901=CARTESIAN_POINT('Ctrl Pts',(115.638278723029,-1.12185056467011,-12.4989605577552));
#55902=CARTESIAN_POINT('Ctrl Pts',(115.617876640176,-1.36101788355078,-12.4989937660998));
#55903=CARTESIAN_POINT('Ctrl Pts',(115.608536321962,-1.47051155050242,-12.4990089692783));
#55904=CARTESIAN_POINT('Ctrl Pts',(115.598391441759,-1.5799596952695,-12.4990384938089));
#55905=CARTESIAN_POINT('Ctrl Pts',(115.587450486329,-1.68938454186076,-12.4990815932618));
#55906=CARTESIAN_POINT('',(117.38636,-2.35227454062139,-12.3923653325402));
#55907=CARTESIAN_POINT('Ctrl Pts',(117.38636,-2.35227454062139,-12.3923653325402));
#55908=CARTESIAN_POINT('Ctrl Pts',(117.338714619479,-4.39706681368208,-12.0042301641757));
#55909=CARTESIAN_POINT('Ctrl Pts',(117.291069238959,-6.34293102937998,-11.1003090033835));
#55910=CARTESIAN_POINT('Ctrl Pts',(117.243423858438,-7.95738642299848,-9.78801247670741));
#55911=CARTESIAN_POINT('Ctrl Pts',(117.195778477917,-9.57184181661693,-8.47571595003138));
#55912=CARTESIAN_POINT('Ctrl Pts',(117.148133097396,-10.854888388156,-6.75504405747155));
#55913=CARTESIAN_POINT('Ctrl Pts',(117.100487716876,-11.6521475969046,-4.83303534198435));
#55914=CARTESIAN_POINT('Ctrl Pts',(117.052842336355,-12.4494068056533,-2.91102662649703));
#55915=CARTESIAN_POINT('Ctrl Pts',(117.005196955834,-12.7608786516115,-0.78768108808232));
#55916=CARTESIAN_POINT('Ctrl Pts',(116.957551575314,-12.5493480046075,1.28228001483163));
#55917=CARTESIAN_POINT('Ctrl Pts',(116.909906194793,-12.3378173576035,3.35224111774546));
#55918=CARTESIAN_POINT('Ctrl Pts',(116.862260814272,-11.6032842176373,5.36881778515853));
#55919=CARTESIAN_POINT('Ctrl Pts',(116.814615433752,-10.4338405130142,7.08986170857202));
#55920=CARTESIAN_POINT('Ctrl Pts',(116.766970053231,-9.26439680839113,8.81090563198556));
#55921=CARTESIAN_POINT('Ctrl Pts',(116.71932467271,-7.66004253911114,10.2364168113995));
#55922=CARTESIAN_POINT('Ctrl Pts',(116.671679292189,-5.81339738182608,11.1953181859262));
#55923=CARTESIAN_POINT('Ctrl Pts',(116.624033911669,-3.96675222454101,12.154219560453));
#55924=CARTESIAN_POINT('Ctrl Pts',(116.576388531148,-1.87781617925087,12.6465111300925));
#55925=CARTESIAN_POINT('Ctrl Pts',(116.528743150627,0.202678011015574,12.6130817366708));
#55926=CARTESIAN_POINT('Ctrl Pts',(116.481097770107,2.28317220128196,12.5796523432491));
#55927=CARTESIAN_POINT('Ctrl Pts',(116.433452389586,4.35522453652466,12.0205019867661));
#55928=CARTESIAN_POINT('Ctrl Pts',(116.385807009065,6.17010335026131,11.0027578256209));
#55929=CARTESIAN_POINT('Ctrl Pts',(116.338161628545,7.98498216399802,9.98501366447572));
#55930=CARTESIAN_POINT('Ctrl Pts',(116.290516248024,9.54268745622868,8.50867569866824));
#55931=CARTESIAN_POINT('Ctrl Pts',(116.242870867503,10.6562403533446,6.75095562472453));
#55932=CARTESIAN_POINT('Ctrl Pts',(116.195225486983,11.7697932504605,4.99323555078082));
#55933=CARTESIAN_POINT('Ctrl Pts',(116.147580106462,12.4391937524616,2.95413336870088));
#55934=CARTESIAN_POINT('Ctrl Pts',(116.099934725941,12.5840870659602,0.878419149789012));
#55935=CARTESIAN_POINT('Ctrl Pts',(116.05228934542,12.7289803794587,-1.19729506912286));
#55936=CARTESIAN_POINT('Ctrl Pts',(116.0046439649,12.3493665044547,-3.30962132486667));
#55937=CARTESIAN_POINT('Ctrl Pts',(115.956998584379,11.4908140887213,-5.20500259025563));
#55938=CARTESIAN_POINT('Ctrl Pts',(115.909353203858,10.6322616729878,-7.1003838556446));
#55939=CARTESIAN_POINT('Ctrl Pts',(115.861707823338,9.294770716525,-8.77882013067873));
#55940=CARTESIAN_POINT('Ctrl Pts',(115.814062442817,7.63888959105897,-10.038836111365));
#55941=CARTESIAN_POINT('Ctrl Pts',(115.766417062296,5.98300846559295,-11.2988520920513));
#55942=CARTESIAN_POINT('Ctrl Pts',(115.718771681776,4.00873717112374,-12.1404477783896));
#55943=CARTESIAN_POINT('Ctrl Pts',(115.671126301255,1.95306202538188,-12.462600507892));
#55944=CARTESIAN_POINT('Ctrl Pts',(115.669093947598,1.86537547835027,-12.476342202695));
#55945=CARTESIAN_POINT('Ctrl Pts',(115.667061593941,1.77754081533774,-12.4891387603591));
#55946=CARTESIAN_POINT('Ctrl Pts',(115.665029240284,1.68957794637772,-12.5009920189268));
#55947=CARTESIAN_POINT('Ctrl Pts',(117.38636,-9.24570028839869,7.00280438584343));
#55948=CARTESIAN_POINT('Ctrl Pts',(117.38636,-9.37284071329502,6.84941999305855));
#55949=CARTESIAN_POINT('Ctrl Pts',(117.38636,-9.49588388830964,6.69285254633599));
#55950=CARTESIAN_POINT('Ctrl Pts',(117.38636,-9.61468485491513,6.53324017247767));
#55951=CARTESIAN_POINT('Ctrl Pts',(117.38636,-9.78004470797177,6.31107465109028));
#55952=CARTESIAN_POINT('Ctrl Pts',(117.38636,-9.9371875313824,6.08301130262427));
#55953=CARTESIAN_POINT('Ctrl Pts',(117.38636,-10.0859821306484,5.84958579014008));
#55954=CARTESIAN_POINT('Ctrl Pts',(117.38636,-10.2358733994428,5.61443984796328));
#55955=CARTESIAN_POINT('Ctrl Pts',(117.38636,-10.3772932439531,5.37385189057232));
#55956=CARTESIAN_POINT('Ctrl Pts',(117.38636,-10.5100664873751,5.12833571523603));
#55957=CARTESIAN_POINT('Ctrl Pts',(117.38636,-10.5658598569975,5.02516602256461));
#55958=CARTESIAN_POINT('Ctrl Pts',(117.38636,-10.620125878563,4.92112573792297));
#55959=CARTESIAN_POINT('Ctrl Pts',(117.38636,-10.6728492069859,4.81625156664499));
#55960=CARTESIAN_POINT('Ctrl Pts',(117.38636,-10.6937228617391,4.77473090948504));
#55961=CARTESIAN_POINT('Ctrl Pts',(117.38636,-10.7143546925228,4.73307953733116));
#55962=CARTESIAN_POINT('Ctrl Pts',(117.38636,-10.7347436840285,4.69129969754066));
#55963=CARTESIAN_POINT('Ctrl Pts',(117.38636,-10.7509151596584,4.65816212617968));
#55964=CARTESIAN_POINT('Ctrl Pts',(117.38636,-10.7669324216288,4.62494663051733));
#55965=CARTESIAN_POINT('Ctrl Pts',(117.38636,-10.7827907480625,4.59166356955379));
#55966=CARTESIAN_POINT('Ctrl Pts',(117.38636,-10.9034104334192,4.33850997494812));
#55967=CARTESIAN_POINT('Ctrl Pts',(117.38636,-11.014913595354,4.08129723752002));
#55968=CARTESIAN_POINT('Ctrl Pts',(117.38636,-11.1171584437568,3.8205625901497));
#55969=CARTESIAN_POINT('Ctrl Pts',(117.38636,-11.2200231885224,3.55824714470407));
#55970=CARTESIAN_POINT('Ctrl Pts',(117.38636,-11.313517322248,3.2923664039607));
#55971=CARTESIAN_POINT('Ctrl Pts',(117.38636,-11.3974521500579,3.02343941709135));
#55972=CARTESIAN_POINT('Ctrl Pts',(117.38636,-11.4811108269362,2.75539721714456));
#55973=CARTESIAN_POINT('Ctrl Pts',(117.38636,-11.5552732415844,2.48432819553525));
#55974=CARTESIAN_POINT('Ctrl Pts',(117.38636,-11.6197046335814,2.21072714127617));
#55975=CARTESIAN_POINT('Ctrl Pts',(117.38636,-11.6316456897028,2.16002071630966));
#55976=CARTESIAN_POINT('Ctrl Pts',(117.38636,-11.6432523742739,2.10922728434781));
#55977=CARTESIAN_POINT('Ctrl Pts',(117.38636,-11.654523000657,2.05834994746899));
#55978=CARTESIAN_POINT('Ctrl Pts',(117.38636,-11.6617905024604,2.02554332919));
#55979=CARTESIAN_POINT('Ctrl Pts',(117.38636,-11.6689182842477,1.99270157512914));
#55980=CARTESIAN_POINT('Ctrl Pts',(117.38636,-11.6759028644632,1.95984029488391));
#55981=CARTESIAN_POINT('Ctrl Pts',(117.38636,-11.7290005457511,1.71002459639411));
#55982=CARTESIAN_POINT('Ctrl Pts',(117.38636,-11.7738715396368,1.45887320689027));
#55983=CARTESIAN_POINT('Ctrl Pts',(117.38636,-11.8104156759069,1.20677663752006));
#55984=CARTESIAN_POINT('Ctrl Pts',(117.38636,-11.8505820658636,0.929692263785574));
#55985=CARTESIAN_POINT('Ctrl Pts',(117.38636,-11.8806903110308,0.651465919625066));
#55986=CARTESIAN_POINT('Ctrl Pts',(117.38636,-11.9009063549852,0.372629730453109));
#55987=CARTESIAN_POINT('Ctrl Pts',(117.38636,-11.9213338464699,0.0908770842498219));
#55988=CARTESIAN_POINT('Ctrl Pts',(117.38636,-11.931661168529,-0.191498807233445));
#55989=CARTESIAN_POINT('Ctrl Pts',(117.38636,-11.9320077592467,-0.473963199932295));
#55990=CARTESIAN_POINT('Ctrl Pts',(117.38636,-11.932355959454,-0.75773929399841));
#55991=CARTESIAN_POINT('Ctrl Pts',(117.38636,-11.9226305225265,-1.04160533140647));
#55992=CARTESIAN_POINT('Ctrl Pts',(117.38636,-11.9029002560441,-1.32502434709932));
#55993=CARTESIAN_POINT('Ctrl Pts',(117.38636,-11.8832211539417,-1.60770840271309));
#55994=CARTESIAN_POINT('Ctrl Pts',(117.38636,-11.8535889969035,-1.889948378621));
#55995=CARTESIAN_POINT('Ctrl Pts',(117.38636,-11.8140205502011,-2.17120735959316));
#55996=CARTESIAN_POINT('Ctrl Pts',(117.38636,-11.7991823826877,-2.27667947745771));
#55997=CARTESIAN_POINT('Ctrl Pts',(117.38636,-11.7829464081973,-2.38201355312953));
#55998=CARTESIAN_POINT('Ctrl Pts',(117.38636,-11.7653116551779,-2.48718084494898));
#55999=CARTESIAN_POINT('Ctrl Pts',(117.38636,-11.7600470974409,-2.51857676408778));
#56000=CARTESIAN_POINT('Ctrl Pts',(117.38636,-11.7546578709007,-2.54995781703081));
#56001=CARTESIAN_POINT('Ctrl Pts',(117.38636,-11.7491439322613,-2.58132323346777));
#56002=CARTESIAN_POINT('Ctrl Pts',(117.38636,-11.7438282333261,-2.61156098576466));
#56003=CARTESIAN_POINT('Ctrl Pts',(117.38636,-11.7383980260217,-2.64177618345329));
#56004=CARTESIAN_POINT('Ctrl Pts',(117.38636,-11.7328543766207,-2.67196331422791));
#56005=CARTESIAN_POINT('Ctrl Pts',(117.38636,-11.6810079485269,-2.95428544390265));
#56006=CARTESIAN_POINT('Ctrl Pts',(117.38636,-11.6192195647412,-3.23428733063864));
#56007=CARTESIAN_POINT('Ctrl Pts',(117.38636,-11.5476371290337,-3.51142874506684));
#56008=CARTESIAN_POINT('Ctrl Pts',(117.38636,-11.4756696433579,-3.7900609343167));
#56009=CARTESIAN_POINT('Ctrl Pts',(117.38636,-11.3938024458907,-4.06580242731433));
#56010=CARTESIAN_POINT('Ctrl Pts',(117.38636,-11.3021334566762,-4.33810671920979));
#56011=CARTESIAN_POINT('Ctrl Pts',(117.38636,-11.2677183953176,-4.44033724443006));
#56012=CARTESIAN_POINT('Ctrl Pts',(117.38636,-11.2319212866881,-4.54208328651749));
#56013=CARTESIAN_POINT('Ctrl Pts',(117.38636,-11.1947454245643,-4.64331573484444));
#56014=CARTESIAN_POINT('Ctrl Pts',(117.38636,-11.0961898713248,-4.91168933482804));
#56015=CARTESIAN_POINT('Ctrl Pts',(117.38636,-10.9879479086506,-5.17645443756622));
#56016=CARTESIAN_POINT('Ctrl Pts',(117.38636,-10.8703739909169,-5.43719361311492));
#56017=CARTESIAN_POINT('Ctrl Pts',(117.38636,-10.7523359767629,-5.69896199752504));
#56018=CARTESIAN_POINT('Ctrl Pts',(117.38636,-10.6248919031944,-5.95667315088571));
#56019=CARTESIAN_POINT('Ctrl Pts',(117.38636,-10.488351543623,-6.20988512596418));
#56020=CARTESIAN_POINT('Ctrl Pts',(117.38636,-10.402408064239,-6.369265972977));
#56021=CARTESIAN_POINT('Ctrl Pts',(117.38636,-10.3128597651542,-6.52686387259263));
#56022=CARTESIAN_POINT('Ctrl Pts',(117.38636,-10.2197748068755,-6.68256318039236));
#56023=CARTESIAN_POINT('Ctrl Pts',(117.38636,-10.1765977533944,-6.75478362786477));
#56024=CARTESIAN_POINT('Ctrl Pts',(117.38636,-10.1326596830689,-6.82659552196018));
#56025=CARTESIAN_POINT('Ctrl Pts',(117.38636,-10.0879669200322,-6.8979869548852));
#56026=CARTESIAN_POINT('Ctrl Pts',(117.38636,-10.0639646559907,-6.93632774894085));
#56027=CARTESIAN_POINT('Ctrl Pts',(117.38636,-10.0397410183703,-6.97455292077738));
#56028=CARTESIAN_POINT('Ctrl Pts',(117.38636,-10.0153169542022,-7.01262974883411));
#56029=CARTESIAN_POINT('Ctrl Pts',(117.38636,-9.85868284503341,-7.25682047817356));
#56030=CARTESIAN_POINT('Ctrl Pts',(117.38636,-9.69369422294742,-7.49510168726722));
#56031=CARTESIAN_POINT('Ctrl Pts',(117.38636,-9.52075996409615,-7.72707136358586));
#56032=CARTESIAN_POINT('Ctrl Pts',(117.38636,-9.346793083249,-7.96042617314377));
#56033=CARTESIAN_POINT('Ctrl Pts',(117.38636,-9.16478509439432,-8.18739439224378));
#56034=CARTESIAN_POINT('Ctrl Pts',(117.38636,-8.97510211448885,-8.40754900414395));
#56035=CARTESIAN_POINT('Ctrl Pts',(117.38636,-8.78560397283429,-8.62748908444294));
#56036=CARTESIAN_POINT('Ctrl Pts',(117.38636,-8.58844544212308,-8.84062935769821));
#56037=CARTESIAN_POINT('Ctrl Pts',(117.38636,-8.38394663465303,-9.04651838120069));
#56038=CARTESIAN_POINT('Ctrl Pts',(117.38636,-8.19583745966281,-9.23590635284578));
#56039=CARTESIAN_POINT('Ctrl Pts',(117.38636,-8.00151675320351,-9.41915884654599));
#56040=CARTESIAN_POINT('Ctrl Pts',(117.38636,-7.80120380491192,-9.59589947210861));
#56041=CARTESIAN_POINT('Ctrl Pts',(117.38636,-7.60816020747953,-9.76622618569375));
#56042=CARTESIAN_POINT('Ctrl Pts',(117.38636,-7.40955096338507,-9.93050511826213));
#56043=CARTESIAN_POINT('Ctrl Pts',(117.38636,-7.20570423293078,-10.0885700721869));
#56044=CARTESIAN_POINT('Ctrl Pts',(117.38636,-7.11652128835703,-10.157723489529));
#56045=CARTESIAN_POINT('Ctrl Pts',(117.38636,-7.02633560821988,-10.2256871780914));
#56046=CARTESIAN_POINT('Ctrl Pts',(117.38636,-6.93517361060053,-10.2924456014955));
#56047=CARTESIAN_POINT('Ctrl Pts',(117.38636,-6.89807959236754,-10.3196097514662));
#56048=CARTESIAN_POINT('Ctrl Pts',(117.38636,-6.86082391907642,-10.346574334626));
#56049=CARTESIAN_POINT('Ctrl Pts',(117.38636,-6.82340834383462,-10.3733382551376));
#56050=CARTESIAN_POINT('Ctrl Pts',(117.38636,-6.7881148669079,-10.3985842069889));
#56051=CARTESIAN_POINT('Ctrl Pts',(117.38636,-6.7526742587066,-10.4236549403665));
#56052=CARTESIAN_POINT('Ctrl Pts',(117.38636,-6.7171154240662,-10.4485305135992));
#56053=CARTESIAN_POINT('Ctrl Pts',(117.38636,-6.47938551746104,-10.6148370801999));
#56054=CARTESIAN_POINT('Ctrl Pts',(117.38636,-6.2361868719198,-10.7725611084642));
#56055=CARTESIAN_POINT('Ctrl Pts',(117.38636,-5.98806594605025,-10.9215634745735));
#56056=CARTESIAN_POINT('Ctrl Pts',(117.38636,-5.73703327091479,-11.0723144135959));
#56057=CARTESIAN_POINT('Ctrl Pts',(117.38636,-5.48096165954196,-11.2141381368804));
#56058=CARTESIAN_POINT('Ctrl Pts',(117.38636,-5.22037762132249,-11.3468546933849));
#56059=CARTESIAN_POINT('Ctrl Pts',(117.38636,-4.95798157512453,-11.4804941132424));
#56060=CARTESIAN_POINT('Ctrl Pts',(117.38636,-4.69100962319276,-11.6048996158117));
#56061=CARTESIAN_POINT('Ctrl Pts',(117.38636,-4.41996688550316,-11.7198460929511));
#56062=CARTESIAN_POINT('Ctrl Pts',(117.38636,-4.14963820346103,-11.8344897463297));
#56063=CARTESIAN_POINT('Ctrl Pts',(117.38636,-3.87525960444849,-11.9397244361644));
#56064=CARTESIAN_POINT('Ctrl Pts',(117.38636,-3.59730806781764,-12.0352811531028));
#56065=CARTESIAN_POINT('Ctrl Pts',(117.38636,-3.32284233014359,-12.1296394902508));
#56066=CARTESIAN_POINT('Ctrl Pts',(117.38636,-3.0448921588925,-12.2145612801996));
#56067=CARTESIAN_POINT('Ctrl Pts',(117.38636,-2.76390145338711,-12.2897393778152));
#56068=CARTESIAN_POINT('Ctrl Pts',(117.38636,-2.62739354564631,-12.3262615994132));
#56069=CARTESIAN_POINT('Ctrl Pts',(117.38636,-2.49016785801523,-12.3604834582857));
#56070=CARTESIAN_POINT('Ctrl Pts',(117.38636,-2.35227454062139,-12.3923653325402));
#56071=CARTESIAN_POINT('',(111.683757644765,-0.266838057499402,11.5945698937334));
#56072=CARTESIAN_POINT('Ctrl Pts',(111.683757644765,-0.266838057499279,
11.5945698937334));
#56073=CARTESIAN_POINT('Ctrl Pts',(111.731403025286,-2.17999073594025,11.550540494705));
#56074=CARTESIAN_POINT('Ctrl Pts',(111.826693786327,-5.98222730491411,10.4970119083172));
#56075=CARTESIAN_POINT('Ctrl Pts',(111.969629927889,-10.2510956213232,6.39473628056006));
#56076=CARTESIAN_POINT('Ctrl Pts',(112.070960292334,-11.5321871571861,2.39851641577062));
#56077=CARTESIAN_POINT('Ctrl Pts',(112.124645276257,-11.5984351167873,0.242765543188727));
#56078=CARTESIAN_POINT('Ctrl Pts',(112.13068487966,-11.5982247539793,0.000228379848985077));
#56079=CARTESIAN_POINT('',(111.124564900463,-1.48350560638763,12.5260977628875));
#56080=CARTESIAN_POINT('Ctrl Pts',(111.124564900463,-1.48350560638763,12.5260977628875));
#56081=CARTESIAN_POINT('Ctrl Pts',(111.125186002198,-1.48282544712551,12.5250728625007));
#56082=CARTESIAN_POINT('Ctrl Pts',(111.125806921632,-1.48214462968221,12.5240482877431));
#56083=CARTESIAN_POINT('Ctrl Pts',(111.227713712044,-1.37026603047416,12.3558966615763));
#56084=CARTESIAN_POINT('Ctrl Pts',(111.325614137126,-1.23992587748691,12.195106414339));
#56085=CARTESIAN_POINT('Ctrl Pts',(111.462555136982,-0.999462399074982,
11.9695764102533));
#56086=CARTESIAN_POINT('Ctrl Pts',(111.509793721761,-0.901990255586121,
11.89160363544));
#56087=CARTESIAN_POINT('Ctrl Pts',(111.612711002011,-0.636927615232599,
11.7200941523355));
#56088=CARTESIAN_POINT('Ctrl Pts',(111.660213206423,-0.459521768746652,
11.6391913870854));
#56089=CARTESIAN_POINT('Ctrl Pts',(111.683757644765,-0.266838057499457,
11.5945698937334));
#56090=CARTESIAN_POINT('',(111.958879057757,-1.68935314531936,-12.5));
#56091=CARTESIAN_POINT('Ctrl Pts',(111.958879057757,-1.68955541748203,-12.5010268514762));
#56092=CARTESIAN_POINT('Ctrl Pts',(111.957514912052,-1.74859600312425,-12.4930639346948));
#56093=CARTESIAN_POINT('Ctrl Pts',(111.956150766346,-1.80757882738274,-12.4846753467372));
#56094=CARTESIAN_POINT('Ctrl Pts',(111.954786620641,-1.86649787319551,-12.4758604898197));
#56095=CARTESIAN_POINT('Ctrl Pts',(111.90714124012,-3.92435748925813,-12.167984864517));
#56096=CARTESIAN_POINT('Ctrl Pts',(111.859495859599,-5.90441452319975,-11.3401087063937));
#56097=CARTESIAN_POINT('Ctrl Pts',(111.811850479079,-7.56900845551407,-10.091622733907));
#56098=CARTESIAN_POINT('Ctrl Pts',(111.764205098558,-9.23360238782844,-8.84313676142033));
#56099=CARTESIAN_POINT('Ctrl Pts',(111.716559718037,-10.5827332185155,-7.17404097457016));
#56100=CARTESIAN_POINT('Ctrl Pts',(111.668914337517,-11.4544119717758,-5.2846582934502));
#56101=CARTESIAN_POINT('Ctrl Pts',(111.621268956996,-12.326090725036,-3.3952756123304));
#56102=CARTESIAN_POINT('Ctrl Pts',(111.573623576475,-12.7203174008696,-1.28560603694085));
#56103=CARTESIAN_POINT('Ctrl Pts',(111.525978195955,-12.5898622105802,0.791041652371061));
#56104=CARTESIAN_POINT('Ctrl Pts',(111.478332815434,-12.4594070202909,2.86768934168309));
#56105=CARTESIAN_POINT('Ctrl Pts',(111.430687434913,-11.8042699638786,4.91131514491748));
#56106=CARTESIAN_POINT('Ctrl Pts',(111.383042054393,-10.7028950384141,6.67673663054116));
#56107=CARTESIAN_POINT('Ctrl Pts',(111.335396673872,-9.60152011294972,8.44215811616485));
#56108=CARTESIAN_POINT('Ctrl Pts',(111.287751293351,-8.05390731843317,9.92937528417784));
#56109=CARTESIAN_POINT('Ctrl Pts',(111.240105912831,-6.24626896752157,10.9594393521967));
#56110=CARTESIAN_POINT('Ctrl Pts',(111.201592242041,-4.78508243501816,11.792081425234));
#56111=CARTESIAN_POINT('Ctrl Pts',(111.163078571252,-3.15399164476227,12.326013405269));
#56112=CARTESIAN_POINT('Ctrl Pts',(111.124564900463,-1.48342384617797,12.525386988334));
#56113=CARTESIAN_POINT('',(112.036457811713,1.68935314531921,-12.5));
#56114=CARTESIAN_POINT('Ctrl Pts',(112.036457811713,1.68935476636984,-12.4990499102299));
#56115=CARTESIAN_POINT('Ctrl Pts',(112.036959716875,1.68016666683514,-12.4990469281187));
#56116=CARTESIAN_POINT('Ctrl Pts',(112.037455888181,1.67097827090242,-12.4990440417202));
#56117=CARTESIAN_POINT('Ctrl Pts',(112.03794632125,1.66178956373823,-12.4990412518299));
#56118=CARTESIAN_POINT('Ctrl Pts',(112.051134336919,1.41470016127385,-12.4989662301422));
#56119=CARTESIAN_POINT('Ctrl Pts',(112.060155252986,1.16771479025901,-12.4989633235238));
#56120=CARTESIAN_POINT('Ctrl Pts',(112.064958360416,0.920535224591733,-12.4990345406596));
#56121=CARTESIAN_POINT('Ctrl Pts',(112.067089749543,0.810848767133786,-12.4990661434149));
#56122=CARTESIAN_POINT('Ctrl Pts',(112.068390584884,0.701123401188886,-12.4991120949476));
#56123=CARTESIAN_POINT('Ctrl Pts',(112.068856435388,0.591330175829491,-12.499171086687));
#56124=CARTESIAN_POINT('Ctrl Pts',(112.069609416395,0.41386506032584,-12.4992664384341));
#56125=CARTESIAN_POINT('Ctrl Pts',(112.068179861252,0.236483378848915,-12.4993959394646));
#56126=CARTESIAN_POINT('Ctrl Pts',(112.064568253644,0.0590651986240468,
-12.4995480142417));
#56127=CARTESIAN_POINT('Ctrl Pts',(112.06429895486,0.0458360482258664,-12.4995593536664));
#56128=CARTESIAN_POINT('Ctrl Pts',(112.064017534671,0.0326072159344261,
-12.4995708149892));
#56129=CARTESIAN_POINT('Ctrl Pts',(112.063723996146,0.0193786521511954,
-12.4995823918539));
#56130=CARTESIAN_POINT('Ctrl Pts',(112.0636433441,0.0157439989356551,-12.4995855726896));
#56131=CARTESIAN_POINT('Ctrl Pts',(112.063561777294,0.0121093694575251,
-12.4995887622436));
#56132=CARTESIAN_POINT('Ctrl Pts',(112.063479295797,0.00847476268296781,
-12.4995919603811));
#56133=CARTESIAN_POINT('Ctrl Pts',(112.063430842536,0.00633963470445853,
-12.4995938391078));
#56134=CARTESIAN_POINT('Ctrl Pts',(112.063382073633,0.00420451497177115,
-12.4995957207963));
#56135=CARTESIAN_POINT('Ctrl Pts',(112.063332989103,0.00206940332587123,
-12.4995976054189));
#56136=CARTESIAN_POINT('Ctrl Pts',(112.063290610866,0.000226006437914865,
-12.4995992325505));
#56137=CARTESIAN_POINT('Ctrl Pts',(112.06324799736,-0.00161738424863261,
-12.499600861869));
#56138=CARTESIAN_POINT('Ctrl Pts',(112.063205148597,-0.00346076885055268,
-12.4996024933568));
#56139=CARTESIAN_POINT('Ctrl Pts',(112.063152964918,-0.00570574826303019,
-12.4996044802761));
#56140=CARTESIAN_POINT('Ctrl Pts',(112.063100432316,-0.00795071835605086,
-12.4996064704126));
#56141=CARTESIAN_POINT('Ctrl Pts',(112.06304755081,-0.0101956793305864,
-12.4996084637338));
#56142=CARTESIAN_POINT('Ctrl Pts',(112.062947782304,-0.0144311185522634,
-12.4996122244186));
#56143=CARTESIAN_POINT('Ctrl Pts',(112.062846771942,-0.0186665236572616,
-12.4996159964381));
#56144=CARTESIAN_POINT('Ctrl Pts',(112.062744519841,-0.0229018962879318,
-12.4996197795738));
#56145=CARTESIAN_POINT('Ctrl Pts',(112.06216208786,-0.0470267451542903,
-12.4996413284631));
#56146=CARTESIAN_POINT('Ctrl Pts',(112.061539374057,-0.0711502837398535,
-12.4996632379714));
#56147=CARTESIAN_POINT('Ctrl Pts',(112.060876403028,-0.095272811780564,
-12.49968546635));
#56148=CARTESIAN_POINT('Ctrl Pts',(112.060028749769,-0.126115093862099,
-12.499713886834));
#56149=CARTESIAN_POINT('Ctrl Pts',(112.059115308853,-0.156954914672159,
-12.4997428280354));
#56150=CARTESIAN_POINT('Ctrl Pts',(112.058136142119,-0.187792898288806,
-12.4997721971628));
#56151=CARTESIAN_POINT('Ctrl Pts',(112.053314345881,-0.33965107353463,-12.4999168221212));
#56152=CARTESIAN_POINT('Ctrl Pts',(112.046900761756,-0.491400509089169,
-12.5000720390346));
#56153=CARTESIAN_POINT('Ctrl Pts',(112.03890688688,-0.643114186770904,-12.5002246390813));
#56154=CARTESIAN_POINT('Ctrl Pts',(112.026216652062,-0.883958861557406,
-12.5004668908622));
#56155=CARTESIAN_POINT('Ctrl Pts',(112.009565615222,-1.1242936415883,-12.500703677216));
#56156=CARTESIAN_POINT('Ctrl Pts',(111.989043361922,-1.36439140510506,-12.5008640626113));
#56157=CARTESIAN_POINT('Ctrl Pts',(111.979775372988,-1.4728211853372,-12.5009364937449));
#56158=CARTESIAN_POINT('Ctrl Pts',(111.969717854519,-1.58120197427212,-12.5009931418907));
#56159=CARTESIAN_POINT('Ctrl Pts',(111.958879057757,-1.68955541748221,-12.5010268514762));
#56160=CARTESIAN_POINT('',(113.773164772043,-1.68935314531927,-12.5));
#56161=CARTESIAN_POINT('Ctrl Pts',(113.773164772043,-1.68901173527894,-12.4997638206505));
#56162=CARTESIAN_POINT('Ctrl Pts',(113.738783287824,-3.17726068106174,-12.2972111654493));
#56163=CARTESIAN_POINT('Ctrl Pts',(113.704401803605,-4.63022107289222,-11.8298957681816));
#56164=CARTESIAN_POINT('Ctrl Pts',(113.670020319386,-5.95395763049549,-11.1212072985898));
#56165=CARTESIAN_POINT('Ctrl Pts',(113.622374938865,-7.78837325939539,-10.1391167178218));
#56166=CARTESIAN_POINT('Ctrl Pts',(113.574729558344,-9.37462705959716,-8.6934925839394));
#56167=CARTESIAN_POINT('Ctrl Pts',(113.527084177824,-10.5223094586549,-6.95786367206226));
#56168=CARTESIAN_POINT('Ctrl Pts',(113.479438797303,-11.6699918577127,-5.22223476018512));
#56169=CARTESIAN_POINT('Ctrl Pts',(113.431793416782,-12.3791028556264,-3.19660107031332));
#56170=CARTESIAN_POINT('Ctrl Pts',(113.384148036262,-12.5645226998369,-1.12411413582959));
#56171=CARTESIAN_POINT('Ctrl Pts',(113.336502655741,-12.7499425440475,0.94837279865413));
#56172=CARTESIAN_POINT('Ctrl Pts',(113.28885727522,-12.4116712345548,3.06771297774975));
#56173=CARTESIAN_POINT('Ctrl Pts',(113.2412118947,-11.5903139457204,4.97950658623459));
#56174=CARTESIAN_POINT('Ctrl Pts',(113.193566514179,-10.768956656886,6.89130019471944));
#56175=CARTESIAN_POINT('Ctrl Pts',(113.145921133658,-9.46451338870981,8.5955472325935));
#56176=CARTESIAN_POINT('Ctrl Pts',(113.098275753138,-7.83356592756815,9.88767455482333));
#56177=CARTESIAN_POINT('Ctrl Pts',(113.050630372617,-6.20261846642654,11.1798018770531));
#56178=CARTESIAN_POINT('Ctrl Pts',(113.002984992096,-4.24516681231946,12.0598094836387));
#56179=CARTESIAN_POINT('Ctrl Pts',(112.955339611575,-2.19617816272136,12.4220636309878));
#56180=CARTESIAN_POINT('Ctrl Pts',(112.907694231055,-0.14718951312322,12.7843177783369));
#56181=CARTESIAN_POINT('Ctrl Pts',(112.860048850534,1.99333613196602,12.6288184664494));
#56182=CARTESIAN_POINT('Ctrl Pts',(112.812403470013,3.96845601763776,11.974231479739));
#56183=CARTESIAN_POINT('Ctrl Pts',(112.764758089493,5.94357590330954,11.3196444930286));
#56184=CARTESIAN_POINT('Ctrl Pts',(112.717112708972,7.75329002956387,10.1659698314953));
#56185=CARTESIAN_POINT('Ctrl Pts',(112.669467328451,9.18036504385502,8.65169129805265));
#56186=CARTESIAN_POINT('Ctrl Pts',(112.621821947931,10.6074400581462,7.13741276460996));
#56187=CARTESIAN_POINT('Ctrl Pts',(112.57417656741,11.6518759604741,5.26253035925789));
#56188=CARTESIAN_POINT('Ctrl Pts',(112.526531186889,12.1883019673065,3.25210017371475));
#56189=CARTESIAN_POINT('Ctrl Pts',(112.478885806369,12.7247279741389,1.24166998817161));
#56190=CARTESIAN_POINT('Ctrl Pts',(112.431240425848,12.7531440854758,-0.90430797756259));
#56191=CARTESIAN_POINT('Ctrl Pts',(112.383595045327,12.2701383463594,-2.92823708869029));
#56192=CARTESIAN_POINT('Ctrl Pts',(112.335949664806,11.7871326072431,-4.95216619981793));
#56193=CARTESIAN_POINT('Ctrl Pts',(112.288304284286,10.7927050176734,-6.85404645633905));
#56194=CARTESIAN_POINT('Ctrl Pts',(112.240658903765,9.40622600807702,-8.40557984913739));
#56195=CARTESIAN_POINT('Ctrl Pts',(112.193013523244,8.01974699848061,-9.95711324193578));
#56196=CARTESIAN_POINT('Ctrl Pts',(112.145368142724,6.24121656885751,-11.1582997710113));
#56197=CARTESIAN_POINT('Ctrl Pts',(112.097722762203,4.28412025495413,-11.864955489308));
#56198=CARTESIAN_POINT('Ctrl Pts',(112.07730111204,3.44527426775002,-12.1678405897586));
#56199=CARTESIAN_POINT('Ctrl Pts',(112.056879461876,2.57362339298663,-12.3798739146441));
#56200=CARTESIAN_POINT('Ctrl Pts',(112.036457811713,1.68935476637002,-12.4990499102299));
#56201=CARTESIAN_POINT('',(113.850743525999,1.68935314531929,-12.5));
#56202=CARTESIAN_POINT('Ctrl Pts',(113.850743525998,1.68901803546276,-12.4998490738946));
#56203=CARTESIAN_POINT('Ctrl Pts',(113.851245431161,1.67983313575413,-12.4998578124018));
#56204=CARTESIAN_POINT('Ctrl Pts',(113.851741602467,1.67064795642428,-12.4998665822449));
#56205=CARTESIAN_POINT('Ctrl Pts',(113.852232035536,1.66146248209855,-12.4998753809702));
#56206=CARTESIAN_POINT('Ctrl Pts',(113.865298014292,1.41674567995777,-12.5001097941157));
#56207=CARTESIAN_POINT('Ctrl Pts',(113.874273658148,1.17214237386868,-12.5003668415169));
#56208=CARTESIAN_POINT('Ctrl Pts',(113.879109652811,0.927352163801529,-12.500585695352));
#56209=CARTESIAN_POINT('Ctrl Pts',(113.881320847749,0.815425060722326,-12.5006857633889));
#56210=CARTESIAN_POINT('Ctrl Pts',(113.882666584728,0.703458199116043,-12.5007775539845));
#56211=CARTESIAN_POINT('Ctrl Pts',(113.883142149674,0.591419750083688,-12.5008534506478));
#56212=CARTESIAN_POINT('Ctrl Pts',(113.88389513068,0.414024790970592,-12.5009736208714));
#56213=CARTESIAN_POINT('Ctrl Pts',(113.882465575537,0.236710970496718,-12.5010539805042));
#56214=CARTESIAN_POINT('Ctrl Pts',(113.878853967929,0.0593541582956196,
-12.5010583969255));
#56215=CARTESIAN_POINT('Ctrl Pts',(113.878745629308,0.0540339257122809,
-12.5010585294064));
#56216=CARTESIAN_POINT('Ctrl Pts',(113.878635328905,0.0487137387383808,
-12.501058593009));
#56217=CARTESIAN_POINT('Ctrl Pts',(113.87852306692,0.0433935940314725,-12.5010585866647));
#56218=CARTESIAN_POINT('Ctrl Pts',(113.87835627776,0.0354893826665526,-12.5010585772388));
#56219=CARTESIAN_POINT('Ctrl Pts',(113.878185158713,0.0275852645996462,
-12.5010584134173));
#56220=CARTESIAN_POINT('Ctrl Pts',(113.878009710432,0.0196812288965393,
-12.5010580987177));
#56221=CARTESIAN_POINT('Ctrl Pts',(113.877929058385,0.016047812504426,-12.501057954053));
#56222=CARTESIAN_POINT('Ctrl Pts',(113.877847491578,0.0124144169823269,
-12.5010577775052));
#56223=CARTESIAN_POINT('Ctrl Pts',(113.877765010083,0.00878104134032691,
-12.501057569414));
#56224=CARTESIAN_POINT('Ctrl Pts',(113.877716556822,0.00664663658689854,
-12.5010574471721));
#56225=CARTESIAN_POINT('Ctrl Pts',(113.87766778792,0.00451223907795595,
-12.5010573140449));
#56226=CARTESIAN_POINT('Ctrl Pts',(113.877618703389,0.00237784854568333,
-12.5010571701012));
#56227=CARTESIAN_POINT('Ctrl Pts',(113.877576325151,0.000535074307108699,
-12.5010570458241));
#56228=CARTESIAN_POINT('Ctrl Pts',(113.877533711646,-0.00130769448144772,
-12.5010569134842));
#56229=CARTESIAN_POINT('Ctrl Pts',(113.877490862883,-0.003150457944898,
-12.5010567731257));
#56230=CARTESIAN_POINT('Ctrl Pts',(113.877438679203,-0.00539468091234346,
-12.501056602189));
#56231=CARTESIAN_POINT('Ctrl Pts',(113.877386146601,-0.00763889568166643,
-12.5010564193593));
#56232=CARTESIAN_POINT('Ctrl Pts',(113.877333265096,-0.00988310241490448,
-12.5010562247161));
#56233=CARTESIAN_POINT('Ctrl Pts',(113.87723349659,-0.0141171186989501,
-12.501055857494));
#56234=CARTESIAN_POINT('Ctrl Pts',(113.877132486228,-0.0183511048866481,
-12.501055448223));
#56235=CARTESIAN_POINT('Ctrl Pts',(113.877030234127,-0.0225850627128733,
-12.501054997436));
#56236=CARTESIAN_POINT('Ctrl Pts',(113.876447802145,-0.0467018526614194,
-12.5010524297353));
#56237=CARTESIAN_POINT('Ctrl Pts',(113.875825088342,-0.0708174645771705,
-12.5010485152761));
#56238=CARTESIAN_POINT('Ctrl Pts',(113.875162117312,-0.0949322080277007,
-12.5010433511533));
#56239=CARTESIAN_POINT('Ctrl Pts',(113.874314464092,-0.125764535557451,
-12.5010367484736));
#56240=CARTESIAN_POINT('Ctrl Pts',(113.87340102322,-0.156594634349324,-12.5010281033168));
#56241=CARTESIAN_POINT('Ctrl Pts',(113.872421856537,-0.187423148993577,
-12.5010176130637));
#56242=CARTESIAN_POINT('Ctrl Pts',(113.867600060503,-0.339234696795374,
-12.5009659549938));
#56243=CARTESIAN_POINT('Ctrl Pts',(113.861186476698,-0.490943663131368,
-12.5008698967933));
#56244=CARTESIAN_POINT('Ctrl Pts',(113.853192602255,-0.642625450334506,
-12.5007507198107));
#56245=CARTESIAN_POINT('Ctrl Pts',(113.840649972264,-0.88061874718513,-12.5005637275323));
#56246=CARTESIAN_POINT('Ctrl Pts',(113.824238143371,-1.11813508366469,-12.5003220898495));
#56247=CARTESIAN_POINT('Ctrl Pts',(113.804043611354,-1.3554470748682,-12.5000866508592));
#56248=CARTESIAN_POINT('Ctrl Pts',(113.794578642875,-1.46667275290384,-12.4999763030373));
#56249=CARTESIAN_POINT('Ctrl Pts',(113.784282727988,-1.57785288254529,-12.4998670128323));
#56250=CARTESIAN_POINT('Ctrl Pts',(113.773164772043,-1.68901173527787,-12.4997638206507));
#56251=CARTESIAN_POINT('Ctrl Pts',(115.587450486329,-1.68938454186076,-12.4990815932618));
#56252=CARTESIAN_POINT('Ctrl Pts',(115.567697044117,-2.54471940650875,-12.3838651769404));
#56253=CARTESIAN_POINT('Ctrl Pts',(115.547943601905,-3.38823356963067,-12.1817460641902));
#56254=CARTESIAN_POINT('Ctrl Pts',(115.528190159693,-4.20164592391042,-11.8944119192506));
#56255=CARTESIAN_POINT('Ctrl Pts',(115.480544779172,-6.16359973044633,-11.2013608284406));
#56256=CARTESIAN_POINT('Ctrl Pts',(115.432899398651,-7.95042834650364,-10.0125488741543));
#56257=CARTESIAN_POINT('Ctrl Pts',(115.385254018131,-9.34764570429239,-8.4706778377342));
#56258=CARTESIAN_POINT('Ctrl Pts',(115.33760863761,-10.7448630620811,-6.92880680131414));
#56259=CARTESIAN_POINT('Ctrl Pts',(115.289963257089,-11.7524691616013,-5.03387668276034));
#56260=CARTESIAN_POINT('Ctrl Pts',(115.242317876569,-12.2495137367818,-3.01334970010246));
#56261=CARTESIAN_POINT('Ctrl Pts',(115.194672496048,-12.7465583119623,-0.99282271744458));
#56262=CARTESIAN_POINT('Ctrl Pts',(115.147027115527,-12.7330413628031,1.15330112931739));
#56263=CARTESIAN_POINT('Ctrl Pts',(115.099381735007,-12.2105854182327,3.16740698507967));
#56264=CARTESIAN_POINT('Ctrl Pts',(115.051736354486,-11.6881294736624,5.18151284084189));
#56265=CARTESIAN_POINT('Ctrl Pts',(115.004090973965,-10.656734533681,7.06360070560443));
#56266=CARTESIAN_POINT('Ctrl Pts',(114.956445593445,-9.24020643457968,8.58774989558119));
#56267=CARTESIAN_POINT('Ctrl Pts',(114.908800212924,-7.82367833547828,10.111899085558));
#56268=CARTESIAN_POINT('Ctrl Pts',(114.861154832403,-6.02201707725687,11.278109600749));
#56269=CARTESIAN_POINT('Ctrl Pts',(114.813509451882,-4.05148915570895,11.9463927134979));
#56270=CARTESIAN_POINT('Ctrl Pts',(114.765864071362,-2.08096123416109,12.6146758262467));
#56271=CARTESIAN_POINT('Ctrl Pts',(114.718218690841,0.058433350713282,12.7850315365535));
#56272=CARTESIAN_POINT('Ctrl Pts',(114.67057331032,2.10988751401252,12.4370108110418));
#56273=CARTESIAN_POINT('Ctrl Pts',(114.6229279298,4.16134167731182,12.0889900855301));
#56274=CARTESIAN_POINT('Ctrl Pts',(114.575282549279,6.12485541903599,11.2225929241999));
#56275=CARTESIAN_POINT('Ctrl Pts',(114.527637168758,7.76473391175164,9.94181927604152));
#56276=CARTESIAN_POINT('Ctrl Pts',(114.479991788238,9.4046124044673,8.66104562788315));
#56277=CARTESIAN_POINT('Ctrl Pts',(114.432346407717,10.7208556481745,6.96589549289665));
#56278=CARTESIAN_POINT('Ctrl Pts',(114.384701027196,11.5554653978966,5.05985006458397));
#56279=CARTESIAN_POINT('Ctrl Pts',(114.337055646676,12.3900751476188,3.15380463627128));
#56280=CARTESIAN_POINT('Ctrl Pts',(114.289410266155,12.7430514033559,1.03686391463243));
#56281=CARTESIAN_POINT('Ctrl Pts',(114.241764885634,12.5720238593694,-1.03686031681585));
#56282=CARTESIAN_POINT('Ctrl Pts',(114.194119505113,12.4009963153829,-3.11058454826412));
#56283=CARTESIAN_POINT('Ctrl Pts',(114.146474124593,11.7059649716726,-5.14109228952181));
#56284=CARTESIAN_POINT('Ctrl Pts',(114.098828744072,10.570359492693,-6.88464693599394));
#56285=CARTESIAN_POINT('Ctrl Pts',(114.051183363551,9.43475401371345,-8.62820158246606));
#56286=CARTESIAN_POINT('Ctrl Pts',(114.003537983031,7.85857439946455,-10.0848031341526));
#56287=CARTESIAN_POINT('Ctrl Pts',(113.95589260251,6.03102094707087,-11.0796051181335));
#56288=CARTESIAN_POINT('Ctrl Pts',(113.92084291034,4.68660549206775,-11.8114180017347));
#56289=CARTESIAN_POINT('Ctrl Pts',(113.885793218169,3.20615621736254,-12.2933227819493));
#56290=CARTESIAN_POINT('Ctrl Pts',(113.850743525998,1.68901803546259,-12.4998490738946));
#56291=CARTESIAN_POINT('Ctrl Pts',(110.227483930805,1.91900181571061,-12.4668097796068));
#56292=CARTESIAN_POINT('Ctrl Pts',(110.259102396748,3.28412020033192,-12.2566786630614));
#56293=CARTESIAN_POINT('Ctrl Pts',(110.353957794575,7.2847919271857,-10.9560812916465));
#56294=CARTESIAN_POINT('Ctrl Pts',(110.480431658344,11.2946802597942,-6.74182720966569));
#56295=CARTESIAN_POINT('Ctrl Pts',(110.638523988057,13.1491225142247,0.0172659150134116));
#56296=CARTESIAN_POINT('Ctrl Pts',(110.796616317769,11.5505961778161,7.1230034539131));
#56297=CARTESIAN_POINT('Ctrl Pts',(110.954708647481,5.90917860665286,11.7527359321285));
#56298=CARTESIAN_POINT('Ctrl Pts',(111.049564045308,1.78853735160741,12.562354535742));
#56299=CARTESIAN_POINT('Ctrl Pts',(111.08118251125,0.408063986721388,12.6070376311147));
#56300=CARTESIAN_POINT('Ctrl Pts',(110.423013221971,1.86747807250454,-12.1320853929883));
#56301=CARTESIAN_POINT('Ctrl Pts',(110.454631687913,3.19594406392888,-11.9275961375395));
#56302=CARTESIAN_POINT('Ctrl Pts',(110.54948708574,7.08920078939042,-10.6619188190556));
#56303=CARTESIAN_POINT('Ctrl Pts',(110.67596094951,10.9914266617329,-6.56081426270191));
#56304=CARTESIAN_POINT('Ctrl Pts',(110.834053279222,12.7960785482098,0.0168023382913589));
#56305=CARTESIAN_POINT('Ctrl Pts',(110.992145608934,11.2404714314658,6.93175621391007));
#56306=CARTESIAN_POINT('Ctrl Pts',(111.150237938646,5.75052164312344,11.4371838866961));
#56307=CARTESIAN_POINT('Ctrl Pts',(111.245093336474,1.74051648030636,12.2250648448911));
#56308=CARTESIAN_POINT('Ctrl Pts',(111.276711802416,0.397107778190796,12.2685482330447));
#56309=CARTESIAN_POINT('Ctrl Pts',(110.618542513136,1.81595432929846,-11.7973610063697));
#56310=CARTESIAN_POINT('Ctrl Pts',(110.650160979079,3.10776792752583,-11.5985136120176));
#56311=CARTESIAN_POINT('Ctrl Pts',(110.745016376906,6.89360965159514,-10.3677563464648));
#56312=CARTESIAN_POINT('Ctrl Pts',(110.871490240676,10.6881730636716,-6.37980131573813));
#56313=CARTESIAN_POINT('Ctrl Pts',(111.029582570388,12.4430345821949,0.0163387615693034));
#56314=CARTESIAN_POINT('Ctrl Pts',(111.1876749001,10.9303466851155,6.74050897390706));
#56315=CARTESIAN_POINT('Ctrl Pts',(111.345767229812,5.59186467959401,11.1216318412638));
#56316=CARTESIAN_POINT('Ctrl Pts',(111.440622627639,1.6924956090053,11.8877751540402));
#56317=CARTESIAN_POINT('Ctrl Pts',(111.472241093582,0.386151569660204,11.9300588349748));
#56318=CARTESIAN_POINT('Ctrl Pts',(110.814071804302,1.76443058609239,-11.4626366197512));
#56319=CARTESIAN_POINT('Ctrl Pts',(110.845690270244,3.01959179112279,-11.2694310864958));
#56320=CARTESIAN_POINT('Ctrl Pts',(110.940545668071,6.69801851379986,-10.0735938738739));
#56321=CARTESIAN_POINT('Ctrl Pts',(111.067019531841,10.3849194656103,-6.19878836877434));
#56322=CARTESIAN_POINT('Ctrl Pts',(111.225111861553,12.0899906161801,0.0158751848472512));
#56323=CARTESIAN_POINT('Ctrl Pts',(111.383204191265,10.6202219387652,6.54926173390403));
#56324=CARTESIAN_POINT('Ctrl Pts',(111.541296520977,5.43320771606459,10.8060797958314));
#56325=CARTESIAN_POINT('Ctrl Pts',(111.636151918805,1.64447473770424,11.5504854631893));
#56326=CARTESIAN_POINT('Ctrl Pts',(111.667770384747,0.375195361129611,11.5915694369049));
#56327=CARTESIAN_POINT('',(110.231099956476,2.07496815725958,-12.4418013645918));
#56328=CARTESIAN_POINT('',(110.814071804302,1.7644305860926,-11.4626366197512));
#56329=CARTESIAN_POINT('Ctrl Pts',(110.231099956476,2.07498074443087,-12.4418052243385));
#56330=CARTESIAN_POINT('Ctrl Pts',(110.231972064293,2.07467345273846,-12.4403226893382));
#56331=CARTESIAN_POINT('Ctrl Pts',(110.232844150751,2.07436555040161,-12.438840267401));
#56332=CARTESIAN_POINT('Ctrl Pts',(110.233716214951,2.07405703700522,-12.4373579600969));
#56333=CARTESIAN_POINT('Ctrl Pts',(110.294415797386,2.05258311988967,-12.3341827185608));
#56334=CARTESIAN_POINT('Ctrl Pts',(110.355166952545,2.02809901882949,-12.2312926779149));
#56335=CARTESIAN_POINT('Ctrl Pts',(110.415658732524,2.00040603564854,-12.1292271991975));
#56336=CARTESIAN_POINT('Ctrl Pts',(110.452538273774,1.98352267536519,-12.067001752469));
#56337=CARTESIAN_POINT('Ctrl Pts',(110.489321408438,1.96544758855314,-12.0050823006931));
#56338=CARTESIAN_POINT('Ctrl Pts',(110.525937674498,1.94614368122397,-11.9435859633641));
#56339=CARTESIAN_POINT('Ctrl Pts',(110.583400229787,1.91584971732351,-11.847078671276));
#56340=CARTESIAN_POINT('Ctrl Pts',(110.640785053146,1.88235189016964,-11.7510557289317));
#56341=CARTESIAN_POINT('Ctrl Pts',(110.69768363355,1.84542156071811,-11.6561947635924));
#56342=CARTESIAN_POINT('Ctrl Pts',(110.736753032922,1.82006335705024,-11.5910584998511));
#56343=CARTESIAN_POINT('Ctrl Pts',(110.775593174595,1.79308780999508,-11.5264694206628));
#56344=CARTESIAN_POINT('Ctrl Pts',(110.814071804302,1.76443058609264,-11.4626366197512));
#56345=CARTESIAN_POINT('',(111.05480378529,1.55646560811612,12.5172412639667));
#56346=CARTESIAN_POINT('Ctrl Pts',(111.05480378529,1.55655218426862,12.5176530308837));
#56347=CARTESIAN_POINT('Ctrl Pts',(111.031978228001,2.54616542269904,12.3953416596267));
#56348=CARTESIAN_POINT('Ctrl Pts',(111.009152670712,3.52132431918197,12.1566148832709));
#56349=CARTESIAN_POINT('Ctrl Pts',(110.986327113423,4.45387699804358,11.8039175907423));
#56350=CARTESIAN_POINT('Ctrl Pts',(110.923090181538,7.03746212088551,10.8267894364854));
#56351=CARTESIAN_POINT('Ctrl Pts',(110.859853249654,9.29402914935078,8.97489644519926));
#56352=CARTESIAN_POINT('Ctrl Pts',(110.796616317769,10.7420179308651,6.62780244177627));
#56353=CARTESIAN_POINT('Ctrl Pts',(110.733379385884,12.1900067123795,4.28070843835325));
#56354=CARTESIAN_POINT('Ctrl Pts',(110.670142453999,12.829417246943,1.43841342279337));
#56355=CARTESIAN_POINT('Ctrl Pts',(110.606905522114,12.5480361572827,-1.31144308230768));
#56356=CARTESIAN_POINT('Ctrl Pts',(110.575287056172,12.4073456124525,-2.68637133485819));
#56357=CARTESIAN_POINT('Ctrl Pts',(110.543668590229,12.0364571615664,-4.038189959794));
#56358=CARTESIAN_POINT('Ctrl Pts',(110.512050124287,11.4550408332583,-5.29059021658293));
#56359=CARTESIAN_POINT('Ctrl Pts',(110.448813192402,10.2922081766421,-7.79539073016086));
#56360=CARTESIAN_POINT('Ctrl Pts',(110.385576260517,8.28726401033785,-9.90251777115129));
#56361=CARTESIAN_POINT('Ctrl Pts',(110.322339328632,5.84087296519027,-11.1829367276658));
#56362=CARTESIAN_POINT('Ctrl Pts',(110.29192620458,4.66430743428013,-11.7987404898432));
#56363=CARTESIAN_POINT('Ctrl Pts',(110.261513080528,3.38563409942451,-12.2233245355487));
#56364=CARTESIAN_POINT('Ctrl Pts',(110.231099956476,2.07498074443113,-12.4418052243385));
#56365=CARTESIAN_POINT('',(111.667770384747,0.375195361129818,11.5915694369049));
#56366=CARTESIAN_POINT('Ctrl Pts',(111.667770384747,0.375195361129768,11.5915694369049));
#56367=CARTESIAN_POINT('Ctrl Pts',(111.648728343226,0.485214774885859,11.6162974530754));
#56368=CARTESIAN_POINT('Ctrl Pts',(111.621953768639,0.590095044314391,11.6533229147721));
#56369=CARTESIAN_POINT('Ctrl Pts',(111.542930074451,0.829633389147557,11.7663849110434));
#56370=CARTESIAN_POINT('Ctrl Pts',(111.485269589771,0.956968090875436,11.8514792232639));
#56371=CARTESIAN_POINT('Ctrl Pts',(111.313120815466,1.26580623366652,12.1112516087257));
#56372=CARTESIAN_POINT('Ctrl Pts',(111.185217860899,1.42619077431694,12.3099604514317));
#56373=CARTESIAN_POINT('Ctrl Pts',(111.05480378529,1.55646560811609,12.5172412639668));
#56374=CARTESIAN_POINT('Ctrl Pts',(110.814071804302,1.76443058609239,-11.4626366197512));
#56375=CARTESIAN_POINT('Ctrl Pts',(110.845690270244,3.01959179112279,-11.2694310864958));
#56376=CARTESIAN_POINT('Ctrl Pts',(110.940545668071,6.69801851379986,-10.0735938738739));
#56377=CARTESIAN_POINT('Ctrl Pts',(111.067019531841,10.3849194656103,-6.19878836877434));
#56378=CARTESIAN_POINT('Ctrl Pts',(111.225111861553,12.0899906161801,0.0158751848472512));
#56379=CARTESIAN_POINT('Ctrl Pts',(111.383204191265,10.6202219387652,6.54926173390403));
#56380=CARTESIAN_POINT('Ctrl Pts',(111.541296520977,5.43320771606459,10.8060797958314));
#56381=CARTESIAN_POINT('Ctrl Pts',(111.636151918805,1.64447473770424,11.5504854631893));
#56382=CARTESIAN_POINT('Ctrl Pts',(111.667770384747,0.375195361129611,11.5915694369049));
#56383=CARTESIAN_POINT('Ctrl Pts',(109.326702434851,-2.19316391405416,12.421511425575));
#56384=CARTESIAN_POINT('Ctrl Pts',(109.386775022159,-4.77735704569893,11.965241739134));
#56385=CARTESIAN_POINT('Ctrl Pts',(109.47688390312,-8.4223533736891,10.0292554895209));
#56386=CARTESIAN_POINT('Ctrl Pts',(109.597029077735,-11.4845940933567,5.68566566705009));
#56387=CARTESIAN_POINT('Ctrl Pts',(109.71717425235,-13.0841517589515,0.621609920093159));
#56388=CARTESIAN_POINT('Ctrl Pts',(109.867355720619,-11.971562716397,-6.17807840082615));
#56389=CARTESIAN_POINT('Ctrl Pts',(110.017537188888,-7.07598515172816,-11.0249828325528));
#56390=CARTESIAN_POINT('Ctrl Pts',(110.107646069849,-3.28369789911874,-12.2491959409189));
#56391=CARTESIAN_POINT('Ctrl Pts',(110.137682363503,-1.98801473901782,-12.4559909861499));
#56392=CARTESIAN_POINT('Ctrl Pts',(109.522231726017,-2.13427912645707,12.0880032654038));
#56393=CARTESIAN_POINT('Ctrl Pts',(109.582304313324,-4.6490886326046,11.6439840739673));
#56394=CARTESIAN_POINT('Ctrl Pts',(109.672413194286,-8.1962195738854,9.75997758672801));
#56395=CARTESIAN_POINT('Ctrl Pts',(109.792558368901,-11.1762414529122,5.53300985641644));
#56396=CARTESIAN_POINT('Ctrl Pts',(109.912703543516,-12.732852208436,0.604920165224213));
#56397=CARTESIAN_POINT('Ctrl Pts',(110.062885011785,-11.6501353377852,-6.01220168178129));
#56398=CARTESIAN_POINT('Ctrl Pts',(110.213066480053,-6.88600031747581,-10.7289704058498));
#56399=CARTESIAN_POINT('Ctrl Pts',(110.303175361015,-3.19553310118293,-11.920314320811));
#56400=CARTESIAN_POINT('Ctrl Pts',(110.333211654668,-1.93463805116661,-12.1215570759298));
#56401=CARTESIAN_POINT('Ctrl Pts',(109.717761017183,-2.07539433885998,11.7544951052327));
#56402=CARTESIAN_POINT('Ctrl Pts',(109.77783360449,-4.52082021951027,11.3227264088006));
#56403=CARTESIAN_POINT('Ctrl Pts',(109.867942485451,-7.97008577408171,9.49069968393512));
#56404=CARTESIAN_POINT('Ctrl Pts',(109.988087660066,-10.8678888124676,5.38035404578278));
#56405=CARTESIAN_POINT('Ctrl Pts',(110.108232834681,-12.3815526579205,0.58823041035528));
#56406=CARTESIAN_POINT('Ctrl Pts',(110.25841430295,-11.3287079591734,-5.84632496273644));
#56407=CARTESIAN_POINT('Ctrl Pts',(110.408595771219,-6.69601548322346,-10.4329579791468));
#56408=CARTESIAN_POINT('Ctrl Pts',(110.49870465218,-3.10736830324712,-11.5914327007031));
#56409=CARTESIAN_POINT('Ctrl Pts',(110.528740945834,-1.8812613633154,-11.7871231657096));
#56410=CARTESIAN_POINT('Ctrl Pts',(109.913290308348,-2.01650955126289,11.4209869450615));
#56411=CARTESIAN_POINT('Ctrl Pts',(109.973362895656,-4.39255180641593,11.0014687436339));
#56412=CARTESIAN_POINT('Ctrl Pts',(110.063471776617,-7.74395197427801,9.22142178114223));
#56413=CARTESIAN_POINT('Ctrl Pts',(110.183616951232,-10.5595361720231,5.22769823514912));
#56414=CARTESIAN_POINT('Ctrl Pts',(110.303762125847,-12.0302531074049,0.571540655486336));
#56415=CARTESIAN_POINT('Ctrl Pts',(110.453943594116,-11.0072805805616,-5.68044824369158));
#56416=CARTESIAN_POINT('Ctrl Pts',(110.604125062384,-6.50603064897112,-10.1369455524438));
#56417=CARTESIAN_POINT('Ctrl Pts',(110.694233943346,-3.01920350531131,-11.2625510805952));
#56418=CARTESIAN_POINT('Ctrl Pts',(110.724270236999,-1.82788467546419,-11.4526892554894));
#56419=CARTESIAN_POINT('',(109.326702434851,-2.19316391405513,12.4215114255748));
#56420=CARTESIAN_POINT('',(109.916925613585,-2.16013089941446,11.3946911745123));
#56421=CARTESIAN_POINT('Ctrl Pts',(109.326702434851,-2.19316391405513,12.4215114255748));
#56422=CARTESIAN_POINT('Ctrl Pts',(109.327624760155,-2.19323679357333,12.4198905709872));
#56423=CARTESIAN_POINT('Ctrl Pts',(109.32854712709,-2.1933090913526,12.4182697125788));
#56424=CARTESIAN_POINT('Ctrl Pts',(109.329470288881,-2.19338086437603,12.4166475270919));
#56425=CARTESIAN_POINT('Ctrl Pts',(109.398328572974,-2.19873438667771,12.2956493335014));
#56426=CARTESIAN_POINT('Ctrl Pts',(109.467540319419,-2.20085626981063,12.1744176340077));
#56427=CARTESIAN_POINT('Ctrl Pts',(109.536874740044,-2.19969030210839,12.0534059975458));
#56428=CARTESIAN_POINT('Ctrl Pts',(109.566227462976,-2.19919668974957,12.002175728299));
#56429=CARTESIAN_POINT('Ctrl Pts',(109.59560217221,-2.1981144327467,11.9509847056692));
#56430=CARTESIAN_POINT('Ctrl Pts',(109.6249813567,-2.19644190302192,11.8998664254177));
#56431=CARTESIAN_POINT('Ctrl Pts',(109.690063492132,-2.19273683741327,11.7866268343208));
#56432=CARTESIAN_POINT('Ctrl Pts',(109.755392190482,-2.18612067777798,11.6733542830029));
#56433=CARTESIAN_POINT('Ctrl Pts',(109.820754601349,-2.17648427702135,11.5604583010507));
#56434=CARTESIAN_POINT('Ctrl Pts',(109.852811866484,-2.17175806435727,11.5050879990986));
#56435=CARTESIAN_POINT('Ctrl Pts',(109.884877241005,-2.16630611914395,11.4498080248238));
#56436=CARTESIAN_POINT('Ctrl Pts',(109.916925613585,-2.16011982372873,11.394665082805));
#56437=CARTESIAN_POINT('',(110.134936209547,-2.10638458259796,-12.4365211389598));
#56438=CARTESIAN_POINT('Ctrl Pts',(110.134936209547,-2.10638646513139,-12.4365237339679));
#56439=CARTESIAN_POINT('Ctrl Pts',(110.105815300545,-3.36065871434644,-12.224149455599));
#56440=CARTESIAN_POINT('Ctrl Pts',(110.076694391543,-4.58342315705692,-11.8229864006375));
#56441=CARTESIAN_POINT('Ctrl Pts',(110.047573482542,-5.71689598821299,-11.2459505852671));
#56442=CARTESIAN_POINT('Ctrl Pts',(109.987500895234,-8.05510066466195,-10.0556019462074));
#56443=CARTESIAN_POINT('Ctrl Pts',(109.927428307927,-10.0133316905295,-8.11684017351675));
#56444=CARTESIAN_POINT('Ctrl Pts',(109.867355720619,-11.2149650119742,-5.78752162298753));
#56445=CARTESIAN_POINT('Ctrl Pts',(109.807283133311,-12.4165983334188,-3.45820307245836));
#56446=CARTESIAN_POINT('Ctrl Pts',(109.747210546004,-12.8616339504406,-0.73832774409066));
#56447=CARTESIAN_POINT('Ctrl Pts',(109.687137958696,-12.476793267583,1.85631594768421));
#56448=CARTESIAN_POINT('Ctrl Pts',(109.657101665043,-12.2843729261541,3.15363779357164));
#56449=CARTESIAN_POINT('Ctrl Pts',(109.627065371389,-11.8844835097554,4.41965173031087));
#56450=CARTESIAN_POINT('Ctrl Pts',(109.597029077735,-11.3017587115976,5.59560742648933));
#56451=CARTESIAN_POINT('Ctrl Pts',(109.566992784081,-10.7190339134398,6.77156312266779));
#56452=CARTESIAN_POINT('Ctrl Pts',(109.536956490428,-9.9534737335229,7.85746057828549));
#56453=CARTESIAN_POINT('Ctrl Pts',(109.506920196774,-9.03810068824607,8.7965017986543));
#56454=CARTESIAN_POINT('Ctrl Pts',(109.446847609466,-7.20735459769238,10.6745842393919));
#56455=CARTESIAN_POINT('Ctrl Pts',(109.386775022159,-4.77735704569893,11.965241739134));
#56456=CARTESIAN_POINT('Ctrl Pts',(109.326702434851,-2.19316391405416,12.421511425575));
#56457=CARTESIAN_POINT('',(110.724270236999,-1.82788467546431,-11.4526892554894));
#56458=CARTESIAN_POINT('Ctrl Pts',(110.724270236999,-1.82788467546435,-11.4526892554894));
#56459=CARTESIAN_POINT('Ctrl Pts',(110.667526075141,-1.86589045855304,-11.5451485282515));
#56460=CARTESIAN_POINT('Ctrl Pts',(110.610252804328,-1.90043345022693,-11.6392079111746));
#56461=CARTESIAN_POINT('Ctrl Pts',(110.552831053726,-1.93172806060983,-11.7341940513259));
#56462=CARTESIAN_POINT('Ctrl Pts',(110.511546885066,-1.95422775732101,-11.8024856618947));
#56463=CARTESIAN_POINT('Ctrl Pts',(110.470185965843,-1.97504883978107,-11.8712554904881));
#56464=CARTESIAN_POINT('Ctrl Pts',(110.428889752719,-1.99428382657138,-11.9402424301157));
#56465=CARTESIAN_POINT('Ctrl Pts',(110.368519311111,-2.02240322442872,-12.0410936146522));
#56466=CARTESIAN_POINT('Ctrl Pts',(110.307888837394,-2.04731573305252,-12.1430752821224));
#56467=CARTESIAN_POINT('Ctrl Pts',(110.247288094794,-2.06919976167528,-12.2456458555069));
#56468=CARTESIAN_POINT('Ctrl Pts',(110.209803232032,-2.08273622631927,-12.3090913464659));
#56469=CARTESIAN_POINT('Ctrl Pts',(110.172329744684,-2.09511475306599,-12.3727616097936));
#56470=CARTESIAN_POINT('Ctrl Pts',(110.134936209547,-2.1063864651313,-12.4365237339679));
#56471=CARTESIAN_POINT('Ctrl Pts',(109.916925613585,-2.16011982372873,11.394665082805));
#56472=CARTESIAN_POINT('Ctrl Pts',(109.97578643248,-4.48246569417521,10.9533734556446));
#56473=CARTESIAN_POINT('Ctrl Pts',(110.064683545029,-7.7723495857832,9.18114161129006));
#56474=CARTESIAN_POINT('Ctrl Pts',(110.183616951232,-10.5595361720231,5.22769823514912));
#56475=CARTESIAN_POINT('Ctrl Pts',(110.303762125847,-12.0302531074049,0.571540655486336));
#56476=CARTESIAN_POINT('Ctrl Pts',(110.453943594116,-11.0072805805616,-5.68044824369158));
#56477=CARTESIAN_POINT('Ctrl Pts',(110.604125062384,-6.50603064897112,-10.1369455524438));
#56478=CARTESIAN_POINT('Ctrl Pts',(110.694233943346,-3.01920350531131,-11.2625510805952));
#56479=CARTESIAN_POINT('Ctrl Pts',(110.724270236999,-1.82788467546419,-11.4526892554894));
#56480=CARTESIAN_POINT('Ctrl Pts',(95.8594371265034,7.72546925504647,-9.97100992071173));
#56481=CARTESIAN_POINT('Ctrl Pts',(95.9065289275864,9.35161189059968,-8.71108589744992));
#56482=CARTESIAN_POINT('Ctrl Pts',(96.0007125297526,11.9743288123158,-5.38178778629994));
#56483=CARTESIAN_POINT('Ctrl Pts',(96.1419879330016,13.0987023614745,0.877951574918655));
#56484=CARTESIAN_POINT('Ctrl Pts',(96.283263336251,11.1494228248783,6.93064159208696));
#56485=CARTESIAN_POINT('Ctrl Pts',(96.4245387395001,6.58412487715065,11.3576480982333));
#56486=CARTESIAN_POINT('Ctrl Pts',(96.5658141427494,0.473894921020247,13.1194575864302));
#56487=CARTESIAN_POINT('Ctrl Pts',(96.7070895459985,-5.74751161001273,11.803044595664));
#56488=CARTESIAN_POINT('Ctrl Pts',(96.8483649492477,-10.6203344167321,7.71711632322287));
#56489=CARTESIAN_POINT('Ctrl Pts',(96.9896403524969,-13.0012049341669,1.82047628794835));
#56490=CARTESIAN_POINT('Ctrl Pts',(97.130915755746,-12.3314833773792,-4.50333217630157));
#56491=CARTESIAN_POINT('Ctrl Pts',(97.2721911589953,-8.76830984429102,-9.77047550087133));
#56492=CARTESIAN_POINT('Ctrl Pts',(97.4134665622445,-3.14774639686187,-12.7450839923031));
#56493=CARTESIAN_POINT('Ctrl Pts',(97.5547419654936,3.21140238251377,-12.7291930343172));
#56494=CARTESIAN_POINT('Ctrl Pts',(97.6960173687429,8.81702974551029,-9.72653341454518));
#56495=CARTESIAN_POINT('Ctrl Pts',(97.837292771992,12.3538351844813,-4.44164615268785));
#56496=CARTESIAN_POINT('Ctrl Pts',(97.9785681752412,12.9919449574235,1.8854258374657));
#56497=CARTESIAN_POINT('Ctrl Pts',(98.1198435784903,10.5816334489112,7.77010284454564));
#56498=CARTESIAN_POINT('Ctrl Pts',(98.2611189817397,5.68845452531083,11.8316080695515));
#56499=CARTESIAN_POINT('Ctrl Pts',(98.4023943849887,-0.539459568553354,
13.1169526921166));
#56500=CARTESIAN_POINT('Ctrl Pts',(98.5436697882381,-6.64079523061034,11.3245442816751));
#56501=CARTESIAN_POINT('Ctrl Pts',(98.6849451914871,-11.1839391316803,6.8749523638787));
#56502=CARTESIAN_POINT('Ctrl Pts',(98.8262205947364,-13.1028910201469,0.812226210291635));
#56503=CARTESIAN_POINT('Ctrl Pts',(98.9674959979855,-11.9473893053074,-5.44108015819797));
#56504=CARTESIAN_POINT('Ctrl Pts',(99.1087714012348,-7.98856013847796,-10.4176951105853));
#56505=CARTESIAN_POINT('Ctrl Pts',(99.2500468044839,-2.15530055285767,-12.9499090355197));
#56506=CARTESIAN_POINT('Ctrl Pts',(99.3913222077332,4.18367731586822,-12.4435649481564));
#56507=CARTESIAN_POINT('Ctrl Pts',(99.5325976109823,9.54099993169075,-9.01747108702972));
#56508=CARTESIAN_POINT('Ctrl Pts',(99.6738730142315,12.6596286918811,-3.4755238289693));
#56509=CARTESIAN_POINT('Ctrl Pts',(99.8151484174807,12.8078106257487,2.88191802051974));
#56510=CARTESIAN_POINT('Ctrl Pts',(99.9564238207299,9.95077642323533,8.56314854926595));
#56511=CARTESIAN_POINT('Ctrl Pts',(100.097699223979,4.75889868263185,12.2351276180707));
#56512=CARTESIAN_POINT('Ctrl Pts',(100.238974627228,-1.5496038684364,13.0362645091662));
#56513=CARTESIAN_POINT('Ctrl Pts',(100.380250030477,-7.49450840213069,10.7785809971637));
#56514=CARTESIAN_POINT('Ctrl Pts',(100.521525433727,-11.6809064867182,5.99181843437947));
#56515=CARTESIAN_POINT('Ctrl Pts',(100.662800836976,-13.1265044699315,-0.20086040648071));
#56516=CARTESIAN_POINT('Ctrl Pts',(100.804076240225,-11.4921082058848,-6.34640949563288));
#56517=CARTESIAN_POINT('Ctrl Pts',(100.945351643474,-7.16121134306135,-11.0028412967757));
#56518=CARTESIAN_POINT('Ctrl Pts',(101.086627046723,-1.15001263060479,-13.0775737601236));
#56519=CARTESIAN_POINT('Ctrl Pts',(101.227902449973,5.13102427789648,-12.0837930453008));
#56520=CARTESIAN_POINT('Ctrl Pts',(101.369177853222,10.2081210746434,-8.25467919591338));
#56521=CARTESIAN_POINT('Ctrl Pts',(101.510453256471,12.8899911560635,-2.48869292975802));
#56522=CARTESIAN_POINT('Ctrl Pts',(101.65172865972,12.5473623163237,3.86123858430473));
#56523=CARTESIAN_POINT('Ctrl Pts',(101.793004062969,9.26062875768555,9.30517165421206));
#56524=CARTESIAN_POINT('Ctrl Pts',(101.934279466218,3.80098744854767,12.5657454581098));
#56525=CARTESIAN_POINT('Ctrl Pts',(102.075554869468,-2.55051501846751,12.8779011349908));
#56526=CARTESIAN_POINT('Ctrl Pts',(102.216830272717,-8.30356634394493,10.1683946851865));
#56527=CARTESIAN_POINT('Ctrl Pts',(102.358105675966,-12.1082744048711,5.07298289356143));
#56528=CARTESIAN_POINT('Ctrl Pts',(102.499381079215,-13.0719050413637,-1.21275021813858));
#56529=CARTESIAN_POINT('Ctrl Pts',(102.640656482464,-10.9683526040717,-7.21392442813049));
#56530=CARTESIAN_POINT('Ctrl Pts',(102.781931885714,-6.29119323282064,-11.5224282253931));
#56531=CARTESIAN_POINT('Ctrl Pts',(102.923207288963,-0.13787248061121,-13.1273171547394));
#56532=CARTESIAN_POINT('Ctrl Pts',(103.064482692212,6.04779857842274,-11.6520211490045));
#56533=CARTESIAN_POINT('Ctrl Pts',(103.205758095461,10.8144182157478,-7.44270267825699));
#56534=CARTESIAN_POINT('Ctrl Pts',(103.347033498711,13.0435499812424,-1.48703341887253));
#56535=CARTESIAN_POINT('Ctrl Pts',(103.48830890196,12.2121518853349,4.81755236936213));
#56536=CARTESIAN_POINT('Ctrl Pts',(103.629584305209,8.51530262230923,9.99175088523157));
#56537=CARTESIAN_POINT('Ctrl Pts',(103.770859708458,2.8204284357127,12.8214916425883));
#56538=CARTESIAN_POINT('Ctrl Pts',(103.912135111707,-3.53622919650101,12.6428061589234));
#56539=CARTESIAN_POINT('Ctrl Pts',(104.053410514956,-9.06314837034476,9.49762107680137));
#56540=CARTESIAN_POINT('Ctrl Pts',(104.194685918206,-12.4634964600336,4.12392052468528));
#56541=CARTESIAN_POINT('Ctrl Pts',(104.335961321455,-12.9394180592167,-2.21741398690574));
#56542=CARTESIAN_POINT('Ctrl Pts',(104.477236724704,-10.3792432419859,-8.03845596033345));
#56543=CARTESIAN_POINT('Ctrl Pts',(104.618512127953,-5.3836897176547,-11.9733599933665));
#56544=CARTESIAN_POINT('Ctrl Pts',(104.759787531202,0.875089167220108,-13.0988428279727));
#56545=CARTESIAN_POINT('Ctrl Pts',(104.901062934452,6.92853771680435,-11.1508219275598));
#56546=CARTESIAN_POINT('Ctrl Pts',(105.042338337701,11.3562787952667,-6.58637960659581));
#56547=CARTESIAN_POINT('Ctrl Pts',(105.18361374095,13.1193902093838,-0.47651358412637));
#56548=CARTESIAN_POINT('Ctrl Pts',(105.324889144199,11.8041766362049,5.74516129508806));
#56549=CARTESIAN_POINT('Ctrl Pts',(105.466164547448,7.71923898892298,10.6187953056317));
#56550=CARTESIAN_POINT('Ctrl Pts',(105.607439950697,1.82306414753622,13.0008423923777));
#56551=CARTESIAN_POINT('Ctrl Pts',(105.748715353947,-4.50087301923505,12.332380250059));
#56552=CARTESIAN_POINT('Ctrl Pts',(105.889990757196,-9.76872882267729,8.77025715351674));
#56553=CARTESIAN_POINT('Ctrl Pts',(106.031266160445,-12.7444556205367,3.15028569732799));
#56554=CARTESIAN_POINT('Ctrl Pts',(106.172541563694,-12.7298339305292,-3.20886445301767));
#56555=CARTESIAN_POINT('Ctrl Pts',(106.313816966943,-9.72828818742371,-8.81509345370888));
#56556=CARTESIAN_POINT('Ctrl Pts',(106.455092370193,-4.44411238783274,-12.3529450963602));
#56557=CARTESIAN_POINT('Ctrl Pts',(106.596367773442,1.88284570183887,-12.9923301796687));
#56558=CARTESIAN_POINT('Ctrl Pts',(106.737643176691,7.76797513005415,-10.5831614434048));
#56559=CARTESIAN_POINT('Ctrl Pts',(106.87891857994,11.8305132965046,-5.69085458103121));
#56560=CARTESIAN_POINT('Ctrl Pts',(107.020193983189,13.116978503713,0.536933086160893));
#56561=CARTESIAN_POINT('Ctrl Pts',(107.161469386439,11.3260374316532,6.63834908837963));
#56562=CARTESIAN_POINT('Ctrl Pts',(107.302744789688,6.87682287379193,11.1829109557715));
#56563=CARTESIAN_POINT('Ctrl Pts',(107.396928391854,2.83606438077655,12.4616371835023));
#56564=CARTESIAN_POINT('Ctrl Pts',(107.444020192937,0.782909338906897,12.5893195613048));
#56565=CARTESIAN_POINT('Ctrl Pts',(96.0549664176689,7.51804626524795,-9.70329586726262));
#56566=CARTESIAN_POINT('Ctrl Pts',(96.102058218752,9.10052820445122,-8.47719984838426));
#56567=CARTESIAN_POINT('Ctrl Pts',(96.1962418209181,11.6528271661266,-5.23729086627577));
#56568=CARTESIAN_POINT('Ctrl Pts',(96.3375172241673,12.7470121383177,0.854379241050541));
#56569=CARTESIAN_POINT('Ctrl Pts',(96.4787926274164,10.850069278768,6.74455912216921));
#56570=CARTESIAN_POINT('Ctrl Pts',(96.6200680306657,6.40734611819909,11.0527038614704));
#56571=CARTESIAN_POINT('Ctrl Pts',(96.7613434339148,0.461171201835904,12.767210101226));
#56572=CARTESIAN_POINT('Ctrl Pts',(96.9026188371641,-5.59319528272015,11.4861418007744));
#56573=CARTESIAN_POINT('Ctrl Pts',(97.0438942404132,-10.3351864930717,7.50991760330816));
#56574=CARTESIAN_POINT('Ctrl Pts',(97.1851696436624,-12.6521324429824,1.77159788043193));
#56575=CARTESIAN_POINT('Ctrl Pts',(97.3264450469117,-12.0003924020166,-4.38242112310514));
#56576=CARTESIAN_POINT('Ctrl Pts',(97.4677204501608,-8.53288737565654,-9.50814564449139));
#56577=CARTESIAN_POINT('Ctrl Pts',(97.6089958534101,-3.06323179364365,-12.4028881541422));
#56578=CARTESIAN_POINT('Ctrl Pts',(97.7502712566591,3.12517866436332,-12.387423856325));
#56579=CARTESIAN_POINT('Ctrl Pts',(97.8915466599084,8.58029918448171,-9.4653833698534));
#56580=CARTESIAN_POINT('Ctrl Pts',(98.0328220631576,12.0221440800517,-4.32239132243712));
#56581=CARTESIAN_POINT('Ctrl Pts',(98.1740974664068,12.6431210895909,1.83480358380842));
#56582=CARTESIAN_POINT('Ctrl Pts',(98.3153728696559,10.2975246168824,7.56148147672324));
#56583=CARTESIAN_POINT('Ctrl Pts',(98.4566482729052,5.53572383594821,11.5139383670531));
#56584=CARTESIAN_POINT('Ctrl Pts',(98.5979236761543,-0.524975488312981,
12.7647724614247));
#56585=CARTESIAN_POINT('Ctrl Pts',(98.7391990794036,-6.46249491565236,11.0204888572779));
#56586=CARTESIAN_POINT('Ctrl Pts',(98.8804744826528,-10.8836588489127,6.69036510749853));
#56587=CARTESIAN_POINT('Ctrl Pts',(99.0217498859019,-12.7510883346818,0.790418552611623));
#56588=CARTESIAN_POINT('Ctrl Pts',(99.1630252891511,-11.626610964448,-5.2949912829611));
#56589=CARTESIAN_POINT('Ctrl Pts',(99.3043006924003,-7.77407335801136,-10.1379878985948));
#56590=CARTESIAN_POINT('Ctrl Pts',(99.4455760956495,-2.09743236778966,-12.6022138003064));
#56591=CARTESIAN_POINT('Ctrl Pts',(99.5868514988987,4.07134875321906,-12.1094646676313));
#56592=CARTESIAN_POINT('Ctrl Pts',(99.7281269021479,9.28483132028813,-8.77535882801427));
#56593=CARTESIAN_POINT('Ctrl Pts',(99.8694023053971,12.3197272637194,-3.38220865031525));
#56594=CARTESIAN_POINT('Ctrl Pts',(100.010677708646,12.4639306250573,2.80454070757788));
#56595=CARTESIAN_POINT('Ctrl Pts',(100.151953111896,9.68360562384654,8.33323450578991));
#56596=CARTESIAN_POINT('Ctrl Pts',(100.293228515145,4.63112586258534,11.9066237217606));
#56597=CARTESIAN_POINT('Ctrl Pts',(100.434503918394,-1.50799817992959,12.6862506949854));
#56598=CARTESIAN_POINT('Ctrl Pts',(100.575779321643,-7.29328653605122,10.4891842728473));
#56599=CARTESIAN_POINT('Ctrl Pts',(100.717054724892,-11.3672830074131,5.83094265415717));
#56600=CARTESIAN_POINT('Ctrl Pts',(100.858330128141,-12.7740677812503,-0.195467456917545));
#56601=CARTESIAN_POINT('Ctrl Pts',(100.999605531391,-11.1835538172183,-6.1760132143701));
#56602=CARTESIAN_POINT('Ctrl Pts',(101.14088093464,-6.96893825021501,-10.7074233535142));
#56603=CARTESIAN_POINT('Ctrl Pts',(101.282156337889,-1.11913566374736,-12.7264508238872));
#56604=CARTESIAN_POINT('Ctrl Pts',(101.423431741138,4.99326016787109,-11.7593523674837));
#56605=CARTESIAN_POINT('Ctrl Pts',(101.564707144387,9.93404076655794,-8.03304732060357));
#56606=CARTESIAN_POINT('Ctrl Pts',(101.705982547637,12.5439046704665,-2.42187341224537));
#56607=CARTESIAN_POINT('Ctrl Pts',(101.847257950886,12.2104751551927,3.75756725703116));
#56608=CARTESIAN_POINT('Ctrl Pts',(101.988533354135,9.01198789964593,9.0553348531861));
#56609=CARTESIAN_POINT('Ctrl Pts',(102.129808757384,3.6989338185692,12.2283647235653));
#56610=CARTESIAN_POINT('Ctrl Pts',(102.271084160633,-2.48203562476454,12.5321392572893));
#56611=CARTESIAN_POINT('Ctrl Pts',(102.412359563882,-8.08062188579097,9.89538100052581));
#56612=CARTESIAN_POINT('Ctrl Pts',(102.553634967132,-11.7831764211184,4.93677715068152));
#56613=CARTESIAN_POINT('Ctrl Pts',(102.694910370381,-12.7209343059263,-1.18018879464178));
#56614=CARTESIAN_POINT('Ctrl Pts',(102.83618577363,-10.6738606560499,-7.02023602893248));
#56615=CARTESIAN_POINT('Ctrl Pts',(102.977461176879,-6.12227946633329,-11.2130597672002));
#56616=CARTESIAN_POINT('Ctrl Pts',(103.118736580128,-0.134170709081827,
-12.7748586460875));
#56617=CARTESIAN_POINT('Ctrl Pts',(103.260011983378,5.88541977379334,-11.3391732191078));
#56618=CARTESIAN_POINT('Ctrl Pts',(103.401287386627,10.5240592892947,-7.24287175656932));
#56619=CARTESIAN_POINT('Ctrl Pts',(103.542562789876,12.6933405576622,-1.44710769947736));
#56620=CARTESIAN_POINT('Ctrl Pts',(103.683838193125,11.8842648700219,4.68820474231524));
#56621=CARTESIAN_POINT('Ctrl Pts',(103.825113596374,8.28667320568124,9.72347995261696));
#56622=CARTESIAN_POINT('Ctrl Pts',(103.966388999624,2.7447020714836,12.4772443169718));
#56623=CARTESIAN_POINT('Ctrl Pts',(104.107664402873,-3.44128412477325,12.3033564030119));
#56624=CARTESIAN_POINT('Ctrl Pts',(104.248939806122,-8.81980971091815,9.24261715475003));
#56625=CARTESIAN_POINT('Ctrl Pts',(104.390215209371,-12.1288610335325,4.01319638655437));
#56626=CARTESIAN_POINT('Ctrl Pts',(104.53149061262,-12.5920044987599,-2.15787810324605));
#56627=CARTESIAN_POINT('Ctrl Pts',(104.672766015869,-10.1005684335019,-7.82262951489559));
#56628=CARTESIAN_POINT('Ctrl Pts',(104.814041419119,-5.23914173221625,-11.6518843592313));
#56629=CARTESIAN_POINT('Ctrl Pts',(104.955316822368,0.851593686827586,-12.747148833397));
#56630=CARTESIAN_POINT('Ctrl Pts',(105.096592225617,6.74251173434216,-10.8514308166036));
#56631=CARTESIAN_POINT('Ctrl Pts',(105.237867628866,11.0513713232499,-6.40954030986884));
#56632=CARTESIAN_POINT('Ctrl Pts',(105.379143032115,12.7671445332022,-0.46371955582386));
#56633=CARTESIAN_POINT('Ctrl Pts',(105.520418435365,11.4872434468854,5.59090807196851));
#56634=CARTESIAN_POINT('Ctrl Pts',(105.661693838614,7.51198327704425,10.333688705937));
#56635=CARTESIAN_POINT('Ctrl Pts',(105.802969241863,1.77411625795274,12.6517796351653));
#56636=CARTESIAN_POINT('Ctrl Pts',(105.944244645112,-4.38002799254061,12.0012651943452));
#56637=CARTESIAN_POINT('Ctrl Pts',(106.085520048361,-9.50644586328202,8.53478240110655));
#56638=CARTESIAN_POINT('Ctrl Pts',(106.226795451611,-12.4022766536811,3.0657029158183));
#56639=CARTESIAN_POINT('Ctrl Pts',(106.36807085486,-12.3880475449599,-3.12270887634921));
#56640=CARTESIAN_POINT('Ctrl Pts',(106.509346258109,-9.46709102841112,-8.5784148806465));
#56641=CARTESIAN_POINT('Ctrl Pts',(106.650621661358,-4.32479134103899,-12.0212778901215));
#56642=CARTESIAN_POINT('Ctrl Pts',(106.791897064607,1.83229272286617,-12.6434959689111));
#56643=CARTESIAN_POINT('Ctrl Pts',(106.933172467857,7.559410889752,-10.2990115858828));
#56644=CARTESIAN_POINT('Ctrl Pts',(107.074447871106,11.5128729878322,-5.53805945199291));
#56645=CARTESIAN_POINT('Ctrl Pts',(107.215723274355,12.7647975799994,0.522516840056443));
#56646=CARTESIAN_POINT('Ctrl Pts',(107.356998677604,11.0219419173116,6.46011445048516));
#56647=CARTESIAN_POINT('Ctrl Pts',(107.498274080853,6.69218539563937,10.8826582787472));
#56648=CARTESIAN_POINT('Ctrl Pts',(107.592457683019,2.7599182032822,12.1270516771658));
#56649=CARTESIAN_POINT('Ctrl Pts',(107.639549484103,0.761888816986977,12.2513058799703));
#56650=CARTESIAN_POINT('Ctrl Pts',(96.2504957088345,7.31062327544942,-9.43558181381351));
#56651=CARTESIAN_POINT('Ctrl Pts',(96.2975875099175,8.84944451830277,-8.24331379931861));
#56652=CARTESIAN_POINT('Ctrl Pts',(96.3917711120837,11.3313255199374,-5.09279394625159));
#56653=CARTESIAN_POINT('Ctrl Pts',(96.5330465153328,12.3953219151609,0.830806907182416));
#56654=CARTESIAN_POINT('Ctrl Pts',(96.674321918582,10.5507157326577,6.55847665225147));
#56655=CARTESIAN_POINT('Ctrl Pts',(96.8155973218312,6.23056735924752,10.7477596247075));
#56656=CARTESIAN_POINT('Ctrl Pts',(96.9568727250804,0.448447482651565,12.4149626160218));
#56657=CARTESIAN_POINT('Ctrl Pts',(97.0981481283296,-5.43887895542757,11.1692390058848));
#56658=CARTESIAN_POINT('Ctrl Pts',(97.2394235315788,-10.0500385694113,7.30271888339345));
#56659=CARTESIAN_POINT('Ctrl Pts',(97.3806989348279,-12.3030599517979,1.72271947291551));
#56660=CARTESIAN_POINT('Ctrl Pts',(97.5219743380772,-11.669301426654,-4.26151006990871));
#56661=CARTESIAN_POINT('Ctrl Pts',(97.6632497413264,-8.29746490702205,-9.24581578811144));
#56662=CARTESIAN_POINT('Ctrl Pts',(97.8045251445756,-2.97871719042544,-12.0606923159813));
#56663=CARTESIAN_POINT('Ctrl Pts',(97.9458005478247,3.03895494621288,-12.0456546783329));
#56664=CARTESIAN_POINT('Ctrl Pts',(98.087075951074,8.3435686234531,-9.20423332516161));
#56665=CARTESIAN_POINT('Ctrl Pts',(98.2283513543231,11.6904529756221,-4.2031364921864));
#56666=CARTESIAN_POINT('Ctrl Pts',(98.3696267575724,12.2942972217584,1.78418133015115));
#56667=CARTESIAN_POINT('Ctrl Pts',(98.5109021608215,10.0134157848537,7.35286010890084));
#56668=CARTESIAN_POINT('Ctrl Pts',(98.6521775640708,5.38299314658557,11.1962686645548));
#56669=CARTESIAN_POINT('Ctrl Pts',(98.7934529673199,-0.510491408072604,
12.4125922307329));
#56670=CARTESIAN_POINT('Ctrl Pts',(98.9347283705691,-6.28419460069438,10.7164334328806));
#56671=CARTESIAN_POINT('Ctrl Pts',(99.0760037738183,-10.5833785661451,6.50577785111838));
#56672=CARTESIAN_POINT('Ctrl Pts',(99.2172791770675,-12.3992856492167,0.768610894931606));
#56673=CARTESIAN_POINT('Ctrl Pts',(99.3585545803167,-11.3058326235886,-5.14890240772422));
#56674=CARTESIAN_POINT('Ctrl Pts',(99.4998299835658,-7.55958657754477,-9.85828068660432));
#56675=CARTESIAN_POINT('Ctrl Pts',(99.641105386815,-2.03956418272164,-12.2545185650931));
#56676=CARTESIAN_POINT('Ctrl Pts',(99.7823807900642,3.95902019056991,-11.7753643871063));
#56677=CARTESIAN_POINT('Ctrl Pts',(99.9236561933134,9.02866270888552,-8.53324656899885));
#56678=CARTESIAN_POINT('Ctrl Pts',(100.064931596563,11.9798258355578,-3.28889347166121));
#56679=CARTESIAN_POINT('Ctrl Pts',(100.206206999812,12.120050624366,2.72716339463603));
#56680=CARTESIAN_POINT('Ctrl Pts',(100.347482403061,9.41643482445774,8.10332046231385));
#56681=CARTESIAN_POINT('Ctrl Pts',(100.48875780631,4.50335304253882,11.5781198254505));
#56682=CARTESIAN_POINT('Ctrl Pts',(100.630033209559,-1.46639249142279,12.3362368808045));
#56683=CARTESIAN_POINT('Ctrl Pts',(100.771308612809,-7.09206466997174,10.1997875485309));
#56684=CARTESIAN_POINT('Ctrl Pts',(100.912584016058,-11.053659528108,5.67006687393485));
#56685=CARTESIAN_POINT('Ctrl Pts',(101.053859419307,-12.4216310925691,-0.190074507354378));
#56686=CARTESIAN_POINT('Ctrl Pts',(101.195134822556,-10.8749994285517,-6.00561693310731));
#56687=CARTESIAN_POINT('Ctrl Pts',(101.336410225805,-6.77666515736867,-10.4120054102527));
#56688=CARTESIAN_POINT('Ctrl Pts',(101.477685629055,-1.08825869688992,-12.3753278876509));
#56689=CARTESIAN_POINT('Ctrl Pts',(101.618961032304,4.85549605784568,-11.4349116896665));
#56690=CARTESIAN_POINT('Ctrl Pts',(101.760236435553,9.65996045847248,-7.81141544529376));
#56691=CARTESIAN_POINT('Ctrl Pts',(101.901511838802,12.1978181848694,-2.35505389473272));
#56692=CARTESIAN_POINT('Ctrl Pts',(102.042787242051,11.8735879940617,3.65389592975758));
#56693=CARTESIAN_POINT('Ctrl Pts',(102.1840626453,8.76334704160629,8.80549805216015));
#56694=CARTESIAN_POINT('Ctrl Pts',(102.32533804855,3.59688018859073,11.8909839890208));
#56695=CARTESIAN_POINT('Ctrl Pts',(102.466613451799,-2.41355623106157,12.1863773795878));
#56696=CARTESIAN_POINT('Ctrl Pts',(102.607888855048,-7.85767742763701,9.62236731586513));
#56697=CARTESIAN_POINT('Ctrl Pts',(102.749164258297,-11.4580784373656,4.80057140780163));
#56698=CARTESIAN_POINT('Ctrl Pts',(102.890439661546,-12.369963570489,-1.14762737114499));
#56699=CARTESIAN_POINT('Ctrl Pts',(103.031715064796,-10.3793687080281,-6.82654762973446));
#56700=CARTESIAN_POINT('Ctrl Pts',(103.172990468045,-5.95336569984595,-10.9036913090074));
#56701=CARTESIAN_POINT('Ctrl Pts',(103.314265871294,-0.130468937552451,
-12.4224001374356));
#56702=CARTESIAN_POINT('Ctrl Pts',(103.455541274543,5.72304096916393,-11.026325289211));
#56703=CARTESIAN_POINT('Ctrl Pts',(103.596816677792,10.2337003628415,-7.04304083488165));
#56704=CARTESIAN_POINT('Ctrl Pts',(103.738092081042,12.3431311340821,-1.40718198008219));
#56705=CARTESIAN_POINT('Ctrl Pts',(103.879367484291,11.5563778547088,4.55885711526834));
#56706=CARTESIAN_POINT('Ctrl Pts',(104.02064288754,8.05804378905324,9.45520902000235));
#56707=CARTESIAN_POINT('Ctrl Pts',(104.161918290789,2.66897570725448,12.1329969913553));
#56708=CARTESIAN_POINT('Ctrl Pts',(104.303193694038,-3.34633905304549,11.9639066471004));
#56709=CARTESIAN_POINT('Ctrl Pts',(104.444469097287,-8.57647105149153,8.98761323269872));
#56710=CARTESIAN_POINT('Ctrl Pts',(104.585744500537,-11.7942256070314,3.90247224842346));
#56711=CARTESIAN_POINT('Ctrl Pts',(104.727019903786,-12.244590938303,-2.09834221958635));
#56712=CARTESIAN_POINT('Ctrl Pts',(104.868295307035,-9.82189362501795,-7.60680306945773));
#56713=CARTESIAN_POINT('Ctrl Pts',(105.009570710284,-5.0945937467778,-11.3304087250961));
#56714=CARTESIAN_POINT('Ctrl Pts',(105.150846113533,0.828098206435065,-12.3954548388212));
#56715=CARTESIAN_POINT('Ctrl Pts',(105.292121516783,6.55648575187998,-10.5520397056476));
#56716=CARTESIAN_POINT('Ctrl Pts',(105.433396920032,10.746463851233,-6.23270101314186));
#56717=CARTESIAN_POINT('Ctrl Pts',(105.574672323281,12.4148988570206,-0.450925527521354));
#56718=CARTESIAN_POINT('Ctrl Pts',(105.71594772653,11.1703102575659,5.43665484884896));
#56719=CARTESIAN_POINT('Ctrl Pts',(105.857223129779,7.30472756516552,10.0485821062422));
#56720=CARTESIAN_POINT('Ctrl Pts',(105.998498533029,1.72516836836926,12.3027168779528));
#56721=CARTESIAN_POINT('Ctrl Pts',(106.139773936278,-4.25918296584617,11.6701501386315));
#56722=CARTESIAN_POINT('Ctrl Pts',(106.281049339527,-9.24416290388675,8.29930764869637));
#56723=CARTESIAN_POINT('Ctrl Pts',(106.422324742776,-12.0600976868255,2.98112013430862));
#56724=CARTESIAN_POINT('Ctrl Pts',(106.563600146025,-12.0462611593905,-3.03655329968074));
#56725=CARTESIAN_POINT('Ctrl Pts',(106.704875549275,-9.20589386939853,-8.34173630758412));
#56726=CARTESIAN_POINT('Ctrl Pts',(106.846150952524,-4.20547029424524,-11.6896106838828));
#56727=CARTESIAN_POINT('Ctrl Pts',(106.987426355773,1.78173974389346,-12.2946617581534));
#56728=CARTESIAN_POINT('Ctrl Pts',(107.128701759022,7.35084664944984,-10.0148617283609));
#56729=CARTESIAN_POINT('Ctrl Pts',(107.269977162271,11.1952326791597,-5.38526432295461));
#56730=CARTESIAN_POINT('Ctrl Pts',(107.41125256552,12.4126166562858,0.508100593951989));
#56731=CARTESIAN_POINT('Ctrl Pts',(107.55252796877,10.7178464029699,6.2818798125907));
#56732=CARTESIAN_POINT('Ctrl Pts',(107.693803372019,6.5075479174868,10.5824056017229));
#56733=CARTESIAN_POINT('Ctrl Pts',(107.787986974185,2.68377202578785,11.7924661708293));
#56734=CARTESIAN_POINT('Ctrl Pts',(107.835078775268,0.740868295067057,11.9132921986358));
#56735=CARTESIAN_POINT('Ctrl Pts',(96.446025,7.1032002856509,-9.1678677603644));
#56736=CARTESIAN_POINT('Ctrl Pts',(96.4931168010831,8.59836083215431,-8.00942775025295));
#56737=CARTESIAN_POINT('Ctrl Pts',(96.5873004032492,11.0098238737483,-4.94829702622741));
#56738=CARTESIAN_POINT('Ctrl Pts',(96.7285758064984,12.0436316920041,0.807234573314296));
#56739=CARTESIAN_POINT('Ctrl Pts',(96.8698512097476,10.2513621865474,6.37239418233372));
#56740=CARTESIAN_POINT('Ctrl Pts',(97.0111266129968,6.05378860029595,10.4428153879447));
#56741=CARTESIAN_POINT('Ctrl Pts',(97.152402016246,0.435723763467222,12.0627151308176));
#56742=CARTESIAN_POINT('Ctrl Pts',(97.2936774194952,-5.28456262813498,10.8523362109951));
#56743=CARTESIAN_POINT('Ctrl Pts',(97.4349528227444,-9.76489064575089,7.09552016347875));
#56744=CARTESIAN_POINT('Ctrl Pts',(97.5762282259935,-11.9539874606134,1.6738410653991));
#56745=CARTESIAN_POINT('Ctrl Pts',(97.7175036292427,-11.3382104512914,-4.14059901671228));
#56746=CARTESIAN_POINT('Ctrl Pts',(97.8587790324919,-8.06204243838756,-8.9834859317315));
#56747=CARTESIAN_POINT('Ctrl Pts',(98.0000544357412,-2.89420258720722,-11.7184964778204));
#56748=CARTESIAN_POINT('Ctrl Pts',(98.1413298389903,2.95273122806244,-11.7038855003407));
#56749=CARTESIAN_POINT('Ctrl Pts',(98.2826052422396,8.10683806242452,-8.94308328046984));
#56750=CARTESIAN_POINT('Ctrl Pts',(98.4238806454887,11.3587618711925,-4.08388166193566));
#56751=CARTESIAN_POINT('Ctrl Pts',(98.5651560487379,11.9454733539258,1.73355907649387));
#56752=CARTESIAN_POINT('Ctrl Pts',(98.706431451987,9.7293069528249,7.14423874107845));
#56753=CARTESIAN_POINT('Ctrl Pts',(98.8477068552363,5.23026245722293,10.8785989620564));
#56754=CARTESIAN_POINT('Ctrl Pts',(98.9889822584854,-0.496007327832227,
12.0604120000411));
#56755=CARTESIAN_POINT('Ctrl Pts',(99.1302576617347,-6.10589428573641,10.4123780084834));
#56756=CARTESIAN_POINT('Ctrl Pts',(99.2715330649838,-10.2830982833774,6.32119059473821));
#56757=CARTESIAN_POINT('Ctrl Pts',(99.412808468233,-12.0474829637517,0.746803237251589));
#56758=CARTESIAN_POINT('Ctrl Pts',(99.5540838714822,-10.9850542827293,-5.00281353248734));
#56759=CARTESIAN_POINT('Ctrl Pts',(99.6953592747313,-7.34509979707817,-9.57857347461386));
#56760=CARTESIAN_POINT('Ctrl Pts',(99.8366346779806,-1.98169599765362,-11.9068233298798));
#56761=CARTESIAN_POINT('Ctrl Pts',(99.9779100812298,3.84669162792076,-11.4412641065812));
#56762=CARTESIAN_POINT('Ctrl Pts',(100.119185484479,8.77249409748291,-8.29113430998339));
#56763=CARTESIAN_POINT('Ctrl Pts',(100.260460887728,11.6399244073961,-3.19557829300717));
#56764=CARTESIAN_POINT('Ctrl Pts',(100.401736290977,11.7761706236747,2.64978608169418));
#56765=CARTESIAN_POINT('Ctrl Pts',(100.543011694227,9.14926402506894,7.8734064188378));
#56766=CARTESIAN_POINT('Ctrl Pts',(100.684287097476,4.37558022249231,11.2496159291403));
#56767=CARTESIAN_POINT('Ctrl Pts',(100.825562500725,-1.42478680291599,11.9862230666236));
#56768=CARTESIAN_POINT('Ctrl Pts',(100.966837903974,-6.89084280389226,9.91039082421449));
#56769=CARTESIAN_POINT('Ctrl Pts',(101.108113307223,-10.7400360488029,5.50919109371254));
#56770=CARTESIAN_POINT('Ctrl Pts',(101.249388710472,-12.0691944038879,-0.18468155779121));
#56771=CARTESIAN_POINT('Ctrl Pts',(101.390664113722,-10.5664450398852,-5.83522065184453));
#56772=CARTESIAN_POINT('Ctrl Pts',(101.531939516971,-6.58439206452233,-10.1165874669912));
#56773=CARTESIAN_POINT('Ctrl Pts',(101.67321492022,-1.05738173003248,-12.0242049514145));
#56774=CARTESIAN_POINT('Ctrl Pts',(101.814490323469,4.71773194782029,-11.1104710118493));
#56775=CARTESIAN_POINT('Ctrl Pts',(101.955765726718,9.38588015038702,-7.58978356998396));
#56776=CARTESIAN_POINT('Ctrl Pts',(102.097041129968,11.8517316992723,-2.28823437722007));
#56777=CARTESIAN_POINT('Ctrl Pts',(102.238316533217,11.5367008329307,3.55022460248401));
#56778=CARTESIAN_POINT('Ctrl Pts',(102.379591936466,8.51470618356667,8.55566125113419));
#56779=CARTESIAN_POINT('Ctrl Pts',(102.520867339715,3.49482655861225,11.5536032544763));
#56780=CARTESIAN_POINT('Ctrl Pts',(102.662142742964,-2.34507683735861,11.8406155018864));
#56781=CARTESIAN_POINT('Ctrl Pts',(102.803418146214,-7.63473296948303,9.34935363120446));
#56782=CARTESIAN_POINT('Ctrl Pts',(102.944693549463,-11.1329804536129,4.66436566492173));
#56783=CARTESIAN_POINT('Ctrl Pts',(103.085968952712,-12.0189928350517,-1.1150659476482));
#56784=CARTESIAN_POINT('Ctrl Pts',(103.227244355961,-10.0848767600063,-6.63285923053644));
#56785=CARTESIAN_POINT('Ctrl Pts',(103.36851975921,-5.7844519333586,-10.5943228508145));
#56786=CARTESIAN_POINT('Ctrl Pts',(103.50979516246,-0.126767166023071,-12.0699416287838));
#56787=CARTESIAN_POINT('Ctrl Pts',(103.651070565709,5.56066216453452,-10.7134773593142));
#56788=CARTESIAN_POINT('Ctrl Pts',(103.792345968958,9.94334143638835,-6.84320991319397));
#56789=CARTESIAN_POINT('Ctrl Pts',(103.933621372207,11.992921710502,-1.36725626068703));
#56790=CARTESIAN_POINT('Ctrl Pts',(104.074896775456,11.2284908393957,4.42950948822145));
#56791=CARTESIAN_POINT('Ctrl Pts',(104.216172178705,7.82941437242525,9.18693808738774));
#56792=CARTESIAN_POINT('Ctrl Pts',(104.357447581955,2.59324934302537,11.7887496657387));
#56793=CARTESIAN_POINT('Ctrl Pts',(104.498722985204,-3.25139398131772,11.6244568911889));
#56794=CARTESIAN_POINT('Ctrl Pts',(104.639998388453,-8.33313239206491,8.73260931064738));
#56795=CARTESIAN_POINT('Ctrl Pts',(104.781273791702,-11.4595901805303,3.79174811029255));
#56796=CARTESIAN_POINT('Ctrl Pts',(104.922549194952,-11.8971773778461,-2.03880633592666));
#56797=CARTESIAN_POINT('Ctrl Pts',(105.063824598201,-9.54321881653396,-7.39097662401987));
#56798=CARTESIAN_POINT('Ctrl Pts',(105.20510000145,-4.95004576133935,-11.0089330909609));
#56799=CARTESIAN_POINT('Ctrl Pts',(105.346375404699,0.80460272604254,-12.0437608442455));
#56800=CARTESIAN_POINT('Ctrl Pts',(105.487650807948,6.3704597694178,-10.2526485946914));
#56801=CARTESIAN_POINT('Ctrl Pts',(105.628926211197,10.4415563792162,-6.05586171641488));
#56802=CARTESIAN_POINT('Ctrl Pts',(105.770201614447,12.062653180839,-0.438131499218847));
#56803=CARTESIAN_POINT('Ctrl Pts',(105.911477017696,10.8533770682464,5.28240162572942));
#56804=CARTESIAN_POINT('Ctrl Pts',(106.052752420945,7.09747185328678,9.76347550654746));
#56805=CARTESIAN_POINT('Ctrl Pts',(106.194027824194,1.67622047878578,11.9536541207404));
#56806=CARTESIAN_POINT('Ctrl Pts',(106.335303227443,-4.13833793915172,11.3390350829177));
#56807=CARTESIAN_POINT('Ctrl Pts',(106.476578630693,-8.98187994449148,8.0638328962862));
#56808=CARTESIAN_POINT('Ctrl Pts',(106.617854033942,-11.7179187199699,2.89653735279891));
#56809=CARTESIAN_POINT('Ctrl Pts',(106.759129437191,-11.7044747738212,-2.95039772301226));
#56810=CARTESIAN_POINT('Ctrl Pts',(106.90040484044,-8.94469671038593,-8.10505773452174));
#56811=CARTESIAN_POINT('Ctrl Pts',(107.041680243689,-4.08614924745149,-11.3579434776441));
#56812=CARTESIAN_POINT('Ctrl Pts',(107.182955646938,1.73118676492076,-11.9458275473958));
#56813=CARTESIAN_POINT('Ctrl Pts',(107.324231050188,7.14228240914768,-9.73071187083892));
#56814=CARTESIAN_POINT('Ctrl Pts',(107.465506453437,10.8775923704873,-5.2324691939163));
#56815=CARTESIAN_POINT('Ctrl Pts',(107.606781856686,12.0604357325722,0.493684347847536));
#56816=CARTESIAN_POINT('Ctrl Pts',(107.748057259935,10.4137508886283,6.10364517469624));
#56817=CARTESIAN_POINT('Ctrl Pts',(107.889332663184,6.32291043933424,10.2821529246985));
#56818=CARTESIAN_POINT('Ctrl Pts',(107.983516265351,2.6076258482935,11.4578806644928));
#56819=CARTESIAN_POINT('Ctrl Pts',(108.030608066434,0.719847773147138,11.5752785173012));
#56820=CARTESIAN_POINT('',(97.5221720974271,1.68935314531923,-12.5));
#56821=CARTESIAN_POINT('',(97.4445933434715,-1.68935314531933,-12.5));
#56822=CARTESIAN_POINT('Ctrl Pts',(97.5221720974271,1.68964825725037,-12.4999689146901));
#56823=CARTESIAN_POINT('Ctrl Pts',(97.5226740025917,1.68046138054838,-12.4999601656737));
#56824=CARTESIAN_POINT('Ctrl Pts',(97.5231701738963,1.67127418506373,-12.4999514312872));
#56825=CARTESIAN_POINT('Ctrl Pts',(97.5236606069647,1.66208665598902,-12.499942714296));
#56826=CARTESIAN_POINT('Ctrl Pts',(97.5368990767983,1.41408374930089,-12.4997074128196));
#56827=CARTESIAN_POINT('Ctrl Pts',(97.5459385014033,1.16616936498662,-12.4994871938956));
#56828=CARTESIAN_POINT('Ctrl Pts',(97.5507275875153,0.918043487166526,-12.4993243210419));
#56829=CARTESIAN_POINT('Ctrl Pts',(97.5528264032038,0.809302388574192,-12.499252942058));
#56830=CARTESIAN_POINT('Ctrl Pts',(97.554108886876,0.700520005736422,-12.4991923547014));
#56831=CARTESIAN_POINT('Ctrl Pts',(97.5545707211021,0.591668272259118,-12.4991447798153));
#56832=CARTESIAN_POINT('Ctrl Pts',(97.5553237021087,0.414194877627063,-12.4990672130529));
#56833=CARTESIAN_POINT('Ctrl Pts',(97.5538941469657,0.236797874895364,-12.4990245774829));
#56834=CARTESIAN_POINT('Ctrl Pts',(97.550282539358,0.0593580377332334,-12.4990206764826));
#56835=CARTESIAN_POINT('Ctrl Pts',(97.5500132405737,0.0461272724853178,
-12.4990203856053));
#56836=CARTESIAN_POINT('Ctrl Pts',(97.5497318203845,0.0328967901787399,
-12.4990203069961));
#56837=CARTESIAN_POINT('Ctrl Pts',(97.5494382818607,0.019666541528909,-12.499020440678));
#56838=CARTESIAN_POINT('Ctrl Pts',(97.5493576298141,0.0160314253716483,
-12.4990204774082));
#56839=CARTESIAN_POINT('Ctrl Pts',(97.5492760630078,0.0123963303202657,
-12.4990205301634));
#56840=CARTESIAN_POINT('Ctrl Pts',(97.5491935815112,0.00876125536962051,
-12.4990205989413));
#56841=CARTESIAN_POINT('Ctrl Pts',(97.5491451282504,0.00662585237640505,
-12.4990206393444));
#56842=CARTESIAN_POINT('Ctrl Pts',(97.5490963593478,0.00449045672313693,
-12.4990206852768));
#56843=CARTESIAN_POINT('Ctrl Pts',(97.5490472748175,0.00235506818888803,
-12.4990207367377));
#56844=CARTESIAN_POINT('Ctrl Pts',(97.54900489658,0.00051143228506254,-12.4990207811677));
#56845=CARTESIAN_POINT('Ctrl Pts',(97.5489622830749,-0.0013321980916125,
-12.4990208297187));
#56846=CARTESIAN_POINT('Ctrl Pts',(97.5489194343114,-0.00317582307487278,
-12.4990208823902));
#56847=CARTESIAN_POINT('Ctrl Pts',(97.5488672506322,-0.00542109520812969,
-12.4990209465366));
#56848=CARTESIAN_POINT('Ctrl Pts',(97.5488147180309,-0.00766635902086035,
-12.4990210167944));
#56849=CARTESIAN_POINT('Ctrl Pts',(97.5487618365246,-0.00991161475866892,
-12.4990210931625));
#56850=CARTESIAN_POINT('Ctrl Pts',(97.5486620680182,-0.0141476100486029,
-12.499021237242));
#56851=CARTESIAN_POINT('Ctrl Pts',(97.5485610576552,-0.0183835747721428,
-12.4990214030707));
#56852=CARTESIAN_POINT('Ctrl Pts',(97.5484588055552,-0.0226195105238446,
-12.4990215906396));
#56853=CARTESIAN_POINT('Ctrl Pts',(97.5478763735732,-0.0467475671134927,
-12.4990226590391));
#56854=CARTESIAN_POINT('Ctrl Pts',(97.54725365977,-0.0708744282519931,-12.4990244329689));
#56855=CARTESIAN_POINT('Ctrl Pts',(97.5465906887396,-0.0950003918469058,
-12.4990269093195));
#56856=CARTESIAN_POINT('Ctrl Pts',(97.5457430355439,-0.12584706418141,-12.4990300755009));
#56857=CARTESIAN_POINT('Ctrl Pts',(97.5448295947004,-0.156691459857992,
-12.4990343900702));
#56858=CARTESIAN_POINT('Ctrl Pts',(97.5438504280495,-0.187534199123077,
-12.4990398408432));
#56859=CARTESIAN_POINT('Ctrl Pts',(97.5390286321437,-0.33941579535519,-12.499066682561));
#56860=CARTESIAN_POINT('Ctrl Pts',(97.53261504854,-0.491193024837094,-12.4991213508053));
#56861=CARTESIAN_POINT('Ctrl Pts',(97.5246211743698,-0.642938406805146,
-12.4992001598446));
#56862=CARTESIAN_POINT('Ctrl Pts',(97.5119506489805,-0.883459294926447,
-12.4993250744869));
#56863=CARTESIAN_POINT('Ctrl Pts',(97.4953316149638,-1.12348158708097,-12.4995120880141));
#56864=CARTESIAN_POINT('Ctrl Pts',(97.4748532411262,-1.36327506627391,-12.4997267108814));
#56865=CARTESIAN_POINT('Ctrl Pts',(97.4655588277245,-1.47210888991352,-12.4998241206498));
#56866=CARTESIAN_POINT('Ctrl Pts',(97.4554694162836,-1.58089492867098,-12.4999269917156));
#56867=CARTESIAN_POINT('Ctrl Pts',(97.4445933434715,-1.68965488935079,-12.5000313373793));
#56868=CARTESIAN_POINT('',(99.2588790577572,-1.68935314531934,-12.5));
#56869=CARTESIAN_POINT('Ctrl Pts',(99.2588790577572,-1.68959457872525,-12.5008760874903));
#56870=CARTESIAN_POINT('Ctrl Pts',(99.2559349733328,-1.81702349400399,-12.483721099136));
#56871=CARTESIAN_POINT('Ctrl Pts',(99.2529908889084,-1.94418354975578,-12.4645915828494));
#56872=CARTESIAN_POINT('Ctrl Pts',(99.2500468044839,-2.07101417234007,-12.4434827001368));
#56873=CARTESIAN_POINT('Ctrl Pts',(99.2029550034009,-4.0997204147311,-12.1058377272082));
#56874=CARTESIAN_POINT('Ctrl Pts',(99.1558632023178,-6.04414027660449,-11.2617664188968));
#56875=CARTESIAN_POINT('Ctrl Pts',(99.1087714012347,-7.67615506867945,-10.0102949393431));
#56876=CARTESIAN_POINT('Ctrl Pts',(99.0616796001517,-9.30816986075441,-8.75882345978953));
#56877=CARTESIAN_POINT('Ctrl Pts',(99.0145877990686,-10.6277795830309,-7.09995180899373));
#56878=CARTESIAN_POINT('Ctrl Pts',(98.9674959979855,-11.4801680633091,-5.22829825551425));
#56879=CARTESIAN_POINT('Ctrl Pts',(98.9204041969025,-12.3325565435872,-3.35664470203477));
#56880=CARTESIAN_POINT('Ctrl Pts',(98.8733123958194,-12.7177237818671,-1.27220924587156));
#56881=CARTESIAN_POINT('Ctrl Pts',(98.8262205947364,-12.5904820862625,0.78046284114121));
#56882=CARTESIAN_POINT('Ctrl Pts',(98.7791287936533,-12.463240390658,2.83313492815398));
#56883=CARTESIAN_POINT('Ctrl Pts',(98.7320369925702,-11.8235897611692,4.85404364601633));
#56884=CARTESIAN_POINT('Ctrl Pts',(98.6849451914871,-10.7465737962464,6.60609665791358));
#56885=CARTESIAN_POINT('Ctrl Pts',(98.6378533904041,-9.66955783132365,8.35814966981085));
#56886=CARTESIAN_POINT('Ctrl Pts',(98.5907615893211,-8.15517653096699,9.84134697574299));
#56887=CARTESIAN_POINT('Ctrl Pts',(98.543669788238,-6.38109660377915,10.8816803637826));
#56888=CARTESIAN_POINT('Ctrl Pts',(98.496577987155,-4.60701667659133,11.9220137518223));
#56889=CARTESIAN_POINT('Ctrl Pts',(98.4494861860718,-2.57323812257234,12.5194832219694));
#56890=CARTESIAN_POINT('Ctrl Pts',(98.4023943849888,-0.518363163252151,
12.6039938532821));
#56891=CARTESIAN_POINT('Ctrl Pts',(98.3553025839057,1.53651179606804,12.6885044845949));
#56892=CARTESIAN_POINT('Ctrl Pts',(98.3082107828227,3.61248316068944,12.2600562770732));
#56893=CARTESIAN_POINT('Ctrl Pts',(98.2611189817396,5.4659986636002,11.3689146358113));
#56894=CARTESIAN_POINT('Ctrl Pts',(98.2140271806566,7.31951416651096,10.4777729945495));
#56895=CARTESIAN_POINT('Ctrl Pts',(98.1669353795735,8.95057380771109,9.12393791954758));
#56896=CARTESIAN_POINT('Ctrl Pts',(98.1198435784904,10.1678222130632,7.46624088086662));
#56897=CARTESIAN_POINT('Ctrl Pts',(98.0727517774073,11.3850706184153,5.80854384218565));
#56898=CARTESIAN_POINT('Ctrl Pts',(98.0256599763243,12.1885077879194,3.84698483982568));
#56899=CARTESIAN_POINT('Ctrl Pts',(97.9785681752412,12.4838747438477,1.81169334028676));
#56900=CARTESIAN_POINT('Ctrl Pts',(97.9314763741582,12.7792416997761,-0.22359815925215));
#56901=CARTESIAN_POINT('Ctrl Pts',(97.8843845730751,12.5665384421287,-2.33262215597));
#56902=CARTESIAN_POINT('Ctrl Pts',(97.837292771992,11.8707192401432,-4.26794869797181));
#56903=CARTESIAN_POINT('Ctrl Pts',(97.790200970909,11.1749000381577,-6.20327523997362));
#56904=CARTESIAN_POINT('Ctrl Pts',(97.7431091698259,9.99596489183397,-7.96490432725939));
#56905=CARTESIAN_POINT('Ctrl Pts',(97.6960173687429,8.47222609150605,-9.34616214086427));
#56906=CARTESIAN_POINT('Ctrl Pts',(97.6489255676598,6.94848729117811,-10.7274199544692));
#56907=CARTESIAN_POINT('Ctrl Pts',(97.6018337665767,5.07994483684591,-11.7283064943932));
#56908=CARTESIAN_POINT('Ctrl Pts',(97.5547419654936,3.08581547978386,-12.2313982573528));
#56909=CARTESIAN_POINT('Ctrl Pts',(97.5438853428048,2.62608555813135,-12.3473818749403));
#56910=CARTESIAN_POINT('Ctrl Pts',(97.5330287201159,2.15968075993868,-12.4369079670506));
#56911=CARTESIAN_POINT('Ctrl Pts',(97.5221720974271,1.68964825725054,-12.49996891469));
#56912=CARTESIAN_POINT('',(99.3364578117128,1.68935314531923,-12.5));
#56913=CARTESIAN_POINT('Ctrl Pts',(99.3364578117128,1.68942947079535,-12.4991898294055));
#56914=CARTESIAN_POINT('Ctrl Pts',(99.3369597168759,1.68024149022573,-12.4991852446615));
#56915=CARTESIAN_POINT('Ctrl Pts',(99.3374558881813,1.67105320856025,-12.4991807450271));
#56916=CARTESIAN_POINT('Ctrl Pts',(99.3379463212505,1.66186461098037,-12.4991763316958));
#56917=CARTESIAN_POINT('Ctrl Pts',(99.3511455436766,1.4145681889693,-12.499057553938));
#56918=CARTESIAN_POINT('Ctrl Pts',(99.3601705813528,1.16737258467869,-12.4990036489936));
#56919=CARTESIAN_POINT('Ctrl Pts',(99.3649705958634,0.919979347945403,-12.4990246557219));
#56920=CARTESIAN_POINT('Ctrl Pts',(99.3670947285812,0.810501331341849,-12.4990339517519));
#56921=CARTESIAN_POINT('Ctrl Pts',(99.3683914769703,0.700983945056015,-12.4990576754726));
#56922=CARTESIAN_POINT('Ctrl Pts',(99.3688564353878,0.591398452065715,-12.499095244472));
#56923=CARTESIAN_POINT('Ctrl Pts',(99.3696094163945,0.413929259729071,-12.4991560859192));
#56924=CARTESIAN_POINT('Ctrl Pts',(99.3681798612514,0.236542179380863,-12.4992533708621));
#56925=CARTESIAN_POINT('Ctrl Pts',(99.3645682536437,0.059117500948294,-12.499378606766));
#56926=CARTESIAN_POINT('Ctrl Pts',(99.3642989548594,0.0458878660039798,
-12.4993879449556));
#56927=CARTESIAN_POINT('Ctrl Pts',(99.3640175346701,0.0326585430731007,
-12.4993974350326));
#56928=CARTESIAN_POINT('Ctrl Pts',(99.3637239961464,0.019429482677277,-12.4994070719177));
#56929=CARTESIAN_POINT('Ctrl Pts',(99.3636433440999,0.015794693005883,-12.4994097197286));
#56930=CARTESIAN_POINT('Ctrl Pts',(99.3635617772938,0.0121599266192257,
-12.4994123786186));
#56931=CARTESIAN_POINT('Ctrl Pts',(99.3634792957969,0.00852518249016221,
-12.4994150484795));
#56932=CARTESIAN_POINT('Ctrl Pts',(99.3634308425361,0.00638997384311283,
-12.4994166168733));
#56933=CARTESIAN_POINT('Ctrl Pts',(99.3633820736336,0.00425477328640055,
-12.4994181890527));
#56934=CARTESIAN_POINT('Ctrl Pts',(99.3633329891032,0.00211958059809694,
-12.4994197649956));
#56935=CARTESIAN_POINT('Ctrl Pts',(99.3632906108658,0.000276113782411228,
-12.4994211256215));
#56936=CARTESIAN_POINT('Ctrl Pts',(99.3632479973606,-0.00156734694744143,
-12.4994224890525));
#56937=CARTESIAN_POINT('Ctrl Pts',(99.3632051485971,-0.00341080172588726,
-12.4994238552745));
#56938=CARTESIAN_POINT('Ctrl Pts',(99.363152964918,-0.00565586657044135,
-12.4994255191379));
#56939=CARTESIAN_POINT('Ctrl Pts',(99.3631004323168,-0.00790092226674584,
-12.4994271871404));
#56940=CARTESIAN_POINT('Ctrl Pts',(99.3630475508104,-0.0101459690715854,
-12.499428859256));
#56941=CARTESIAN_POINT('Ctrl Pts',(99.3629477823041,-0.0143815701593871,
-12.4994320139407));
#56942=CARTESIAN_POINT('Ctrl Pts',(99.3628467719413,-0.0186171377382284,
-12.4994351832643));
#56943=CARTESIAN_POINT('Ctrl Pts',(99.3627445198409,-0.0228526734316162,
-12.4994383670504));
#56944=CARTESIAN_POINT('Ctrl Pts',(99.3621620878589,-0.0469784511889833,
-12.4994565020208));
#56945=CARTESIAN_POINT('Ctrl Pts',(99.3615393740557,-0.0711029382673367,
-12.499475106215));
#56946=CARTESIAN_POINT('Ctrl Pts',(99.3608764030252,-0.0952264338341105,
-12.4994941456146));
#56947=CARTESIAN_POINT('Ctrl Pts',(99.360028749832,-0.126069950534176,-12.4995184887716));
#56948=CARTESIAN_POINT('Ctrl Pts',(99.3591153089914,-0.156911037043278,
-12.4995435429306));
#56949=CARTESIAN_POINT('Ctrl Pts',(99.3581361423438,-0.187750316250194,
-12.4995692314194));
#56950=CARTESIAN_POINT('Ctrl Pts',(99.3533143464512,-0.33961487391151,-12.4996957314896));
#56951=CARTESIAN_POINT('Ctrl Pts',(99.346900762868,-0.491371413732186,-12.4998378380961));
#56952=CARTESIAN_POINT('Ctrl Pts',(99.3389068887258,-0.643092774867443,
-12.4999842439063));
#56953=CARTESIAN_POINT('Ctrl Pts',(99.3262196286907,-0.88389320872154,-12.500216607908));
#56954=CARTESIAN_POINT('Ctrl Pts',(99.3095734231148,-1.12418542037101,-12.5004609712747));
#56955=CARTESIAN_POINT('Ctrl Pts',(99.2890577945819,-1.36424153814148,-12.5006536540262));
#56956=CARTESIAN_POINT('Ctrl Pts',(99.2797858146812,-1.47273421704968,-12.5007407364471));
#56957=CARTESIAN_POINT('Ctrl Pts',(99.2697234810396,-1.58117802058591,-12.5008170568316));
#56958=CARTESIAN_POINT('Ctrl Pts',(99.2588790577572,-1.68959457872552,-12.5008760874902));
#56959=CARTESIAN_POINT('',(101.073164772043,-1.68935314531934,-12.5));
#56960=CARTESIAN_POINT('Ctrl Pts',(101.073164772043,-1.68928079698559,-12.5007909894091));
#56961=CARTESIAN_POINT('Ctrl Pts',(101.030560395853,-3.53307800378901,-12.2502869163015));
#56962=CARTESIAN_POINT('Ctrl Pts',(100.987956019664,-5.32172987995247,-11.5875155537485));
#56963=CARTESIAN_POINT('Ctrl Pts',(100.945351643474,-6.88116103478917,-10.5725580738099));
#56964=CARTESIAN_POINT('Ctrl Pts',(100.898259842391,-8.60484363066917,-9.45069736306145));
#56965=CARTESIAN_POINT('Ctrl Pts',(100.851168041308,-10.048475918277,-7.89855342934716));
#56966=CARTESIAN_POINT('Ctrl Pts',(100.804076240225,-11.042691439422,-6.09822328096466));
#56967=CARTESIAN_POINT('Ctrl Pts',(100.756984439142,-12.036906960567,-4.29789313258215));
#56968=CARTESIAN_POINT('Ctrl Pts',(100.709892638059,-12.5817057152493,-2.24937676953143));
#56969=CARTESIAN_POINT('Ctrl Pts',(100.662800836976,-12.6131720953882,-0.193005447862708));
#56970=CARTESIAN_POINT('Ctrl Pts',(100.615709035893,-12.6446384755271,1.86336587380602));
#56971=CARTESIAN_POINT('Ctrl Pts',(100.56861723481,-12.1627724811226,3.92759215409274));
#56972=CARTESIAN_POINT('Ctrl Pts',(100.521525433727,-11.2241064698225,5.75749905470014));
#56973=CARTESIAN_POINT('Ctrl Pts',(100.474433632644,-10.2854404585223,7.58740595530752));
#56974=CARTESIAN_POINT('Ctrl Pts',(100.42734183156,-8.88997443032653,9.18299347623558));
#56975=CARTESIAN_POINT('Ctrl Pts',(100.380250030477,-7.20142399394626,10.3570678220334));
#56976=CARTESIAN_POINT('Ctrl Pts',(100.333158229394,-5.51287355756596,11.5311421678312));
#56977=CARTESIAN_POINT('Ctrl Pts',(100.286066428311,-3.53123871300118,12.2837033384987));
#56978=CARTESIAN_POINT('Ctrl Pts',(100.238974627228,-1.48900419887407,12.5264611086499));
#56979=CARTESIAN_POINT('Ctrl Pts',(100.191882826145,0.553230315253027,12.7692188788011));
#56980=CARTESIAN_POINT('Ctrl Pts',(100.144791025062,2.65606449894247,12.5021732484359));
#56981=CARTESIAN_POINT('Ctrl Pts',(100.097699223979,4.57279454755443,11.7566539217858));
#56982=CARTESIAN_POINT('Ctrl Pts',(100.050607422896,6.48952459616636,11.0111345951358));
#56983=CARTESIAN_POINT('Ctrl Pts',(100.003515621813,8.22015050970083,9.78714157220086));
#56984=CARTESIAN_POINT('Ctrl Pts',(99.9564238207299,9.56163583355362,8.22827330594238));
#56985=CARTESIAN_POINT('Ctrl Pts',(99.9093320196468,10.9031211574064,6.66940503968388));
#56986=CARTESIAN_POINT('Ctrl Pts',(99.8622402185638,11.8554658915775,4.7756615301018));
#56987=CARTESIAN_POINT('Ctrl Pts',(99.8151484174807,12.3069412696852,2.76921613372925));
#56988=CARTESIAN_POINT('Ctrl Pts',(99.7680566163977,12.7584166477928,0.762770737356701));
#56989=CARTESIAN_POINT('Ctrl Pts',(99.7209648153146,12.7090226698369,-1.35637654580632));
#56990=CARTESIAN_POINT('Ctrl Pts',(99.6738730142315,12.1645542208273,-3.33960806373124));
#56991=CARTESIAN_POINT('Ctrl Pts',(99.6267812131484,11.6200857718176,-5.32283958165613));
#56992=CARTESIAN_POINT('Ctrl Pts',(99.5796894120654,10.5805428517542,-7.17015533434292));
#56993=CARTESIAN_POINT('Ctrl Pts',(99.5325976109823,9.16788428908538,-8.66482885420743));
#56994=CARTESIAN_POINT('Ctrl Pts',(99.4855058098992,7.75522572641657,-10.1595023740719));
#56995=CARTESIAN_POINT('Ctrl Pts',(99.4384140088162,5.96945152114239,-11.3015336611142));
#56996=CARTESIAN_POINT('Ctrl Pts',(99.3913222077331,4.02006810705099,-11.9569399858625));
#56997=CARTESIAN_POINT('Ctrl Pts',(99.3730340757264,3.26302377260614,-12.2114674643069));
#56998=CARTESIAN_POINT('Ctrl Pts',(99.3547459437195,2.481304513322,-12.3926039982175));
#56999=CARTESIAN_POINT('Ctrl Pts',(99.3364578117128,1.68942947079438,-12.4991898294056));
#57000=CARTESIAN_POINT('',(101.150743525999,1.68935314531923,-12.5));
#57001=CARTESIAN_POINT('Ctrl Pts',(101.150743525999,1.68914515608837,-12.4990650577849));
#57002=CARTESIAN_POINT('Ctrl Pts',(101.151245431163,1.67995781277747,-12.4990674945739));
#57003=CARTESIAN_POINT('Ctrl Pts',(101.151741602468,1.67077018456029,-12.4990700270579));
#57004=CARTESIAN_POINT('Ctrl Pts',(101.152232035536,1.66158225640466,-12.4990726548156));
#57005=CARTESIAN_POINT('Ctrl Pts',(101.165379558313,1.41527240811885,-12.4991430997065));
#57006=CARTESIAN_POINT('Ctrl Pts',(101.174385531785,1.16907402877139,-12.4992842339152));
#57007=CARTESIAN_POINT('Ctrl Pts',(101.179199712583,0.92268867358122,-12.4994739647979));
#57008=CARTESIAN_POINT('Ctrl Pts',(101.181357422249,0.812259073004665,-12.4995590019364));
#57009=CARTESIAN_POINT('Ctrl Pts',(101.182673075835,0.701791239333902,-12.4996535375347));
#57010=CARTESIAN_POINT('Ctrl Pts',(101.183142149673,0.591255341135298,-12.4997539904862));
#57011=CARTESIAN_POINT('Ctrl Pts',(101.18389513068,0.413817536922243,-12.4999152426352));
#57012=CARTESIAN_POINT('Ctrl Pts',(101.182465575537,0.236465021036391,-12.5000917228813));
#57013=CARTESIAN_POINT('Ctrl Pts',(101.17885396793,0.0590766675822643,-12.5002625611583));
#57014=CARTESIAN_POINT('Ctrl Pts',(101.178584669145,0.0458497412066224,
-12.5002752996796));
#57015=CARTESIAN_POINT('Ctrl Pts',(101.178303248956,0.0326231365233512,
-12.5002880031159));
#57016=CARTESIAN_POINT('Ctrl Pts',(101.178009710432,0.0193968034520138,
-12.5003006612721));
#57017=CARTESIAN_POINT('Ctrl Pts',(101.177929058386,0.0157627631540866,
-12.5003041392013));
#57018=CARTESIAN_POINT('Ctrl Pts',(101.17784749158,0.012128746826254,-12.5003076137077));
#57019=CARTESIAN_POINT('Ctrl Pts',(101.177765010083,0.0084947533778412,
-12.5003110845771));
#57020=CARTESIAN_POINT('Ctrl Pts',(101.177716556821,0.00635998568360754,
-12.5003131235185));
#57021=CARTESIAN_POINT('Ctrl Pts',(101.177667787917,0.00422522631192673,
-12.5003151612044));
#57022=CARTESIAN_POINT('Ctrl Pts',(101.177618703389,0.00209047518892369,
-12.500317197591));
#57023=CARTESIAN_POINT('Ctrl Pts',(101.177576325151,0.000247389521649039,
-12.5003189557515));
#57024=CARTESIAN_POINT('Ctrl Pts',(101.177533711646,-0.00159568988858964,
-12.5003207129434));
#57025=CARTESIAN_POINT('Ctrl Pts',(101.177490862883,-0.00343876317675105,
-12.5003224691385));
#57026=CARTESIAN_POINT('Ctrl Pts',(101.177438679203,-0.00568336343521118,
-12.5003246079335));
#57027=CARTESIAN_POINT('Ctrl Pts',(101.177386146602,-0.00792795429388963,
-12.5003267452498));
#57028=CARTESIAN_POINT('Ctrl Pts',(101.177333265096,-0.0101725359711127,
-12.5003288810365));
#57029=CARTESIAN_POINT('Ctrl Pts',(101.177233496591,-0.0144072595541474,
-12.5003329105027));
#57030=CARTESIAN_POINT('Ctrl Pts',(101.177132486228,-0.0186419487436732,
-12.5003369345226));
#57031=CARTESIAN_POINT('Ctrl Pts',(101.177030234127,-0.0228766052639706,
-12.5003409527519));
#57032=CARTESIAN_POINT('Ctrl Pts',(101.176447802145,-0.0469973749059116,
-12.5003638407438));
#57033=CARTESIAN_POINT('Ctrl Pts',(101.175825088342,-0.07111682585345,-12.5003865408022));
#57034=CARTESIAN_POINT('Ctrl Pts',(101.175162117311,-0.0952352608502072,
-12.5004089879631));
#57035=CARTESIAN_POINT('Ctrl Pts',(101.174314464106,-0.12607230773492,-12.5004376881733));
#57036=CARTESIAN_POINT('Ctrl Pts',(101.173401023251,-0.156906884656046,
-12.5004659744033));
#57037=CARTESIAN_POINT('Ctrl Pts',(101.172421856587,-0.187739621969185,
-12.5004937054932));
#57038=CARTESIAN_POINT('Ctrl Pts',(101.16760006063,-0.339571964404762,-12.5006302641222));
#57039=CARTESIAN_POINT('Ctrl Pts',(101.161186476945,-0.491295520700995,
-12.5007535749172));
#57040=CARTESIAN_POINT('Ctrl Pts',(101.153192602665,-0.642984018431462,
-12.500844739625));
#57041=CARTESIAN_POINT('Ctrl Pts',(101.145167090904,-0.795272856108191,
-12.5009362651368));
#57042=CARTESIAN_POINT('Ctrl Pts',(101.13555745464,-0.947357522802301,-12.5009956204214));
#57043=CARTESIAN_POINT('Ctrl Pts',(101.124386353216,-1.09931002772209,-12.5010000674675));
#57044=CARTESIAN_POINT('Ctrl Pts',(101.109916044249,-1.29613929377952,-12.5010058278782));
#57045=CARTESIAN_POINT('Ctrl Pts',(101.092825767703,-1.49274779624088,-12.5009197918223));
#57046=CARTESIAN_POINT('Ctrl Pts',(101.073164772043,-1.68928079698559,-12.5007909894091));
#57047=CARTESIAN_POINT('',(102.887450486329,-1.68935314531934,-12.5));
#57048=CARTESIAN_POINT('Ctrl Pts',(102.887450486329,-1.68904238362358,-12.4999128886012));
#57049=CARTESIAN_POINT('Ctrl Pts',(102.852277619457,-3.21148927825508,-12.2926905183232));
#57050=CARTESIAN_POINT('Ctrl Pts',(102.817104752585,-4.69695204398918,-11.8079445987757));
#57051=CARTESIAN_POINT('Ctrl Pts',(102.781931885714,-6.04516633599424,-11.071825747407));
#57052=CARTESIAN_POINT('Ctrl Pts',(102.734840084631,-7.85024635657098,-10.0862602929722));
#57053=CARTESIAN_POINT('Ctrl Pts',(102.687748283548,-9.40929948032132,-8.65009236055137));
#57054=CARTESIAN_POINT('Ctrl Pts',(102.640656482464,-10.5394181150785,-6.93181269267563));
#57055=CARTESIAN_POINT('Ctrl Pts',(102.593564681381,-11.6695367498357,-5.21353302479987));
#57056=CARTESIAN_POINT('Ctrl Pts',(102.546472880298,-12.3707208955997,-3.21314162146922));
#57057=CARTESIAN_POINT('Ctrl Pts',(102.499381079215,-12.5607078623996,-1.16532373452056));
#57058=CARTESIAN_POINT('Ctrl Pts',(102.452289278132,-12.7506948291995,0.882494152428101));
#57059=CARTESIAN_POINT('Ctrl Pts',(102.405197477049,-12.4294846170353,2.97773852299478));
#57060=CARTESIAN_POINT('Ctrl Pts',(102.358105675966,-11.6347615007988,4.8745960068823));
#57061=CARTESIAN_POINT('Ctrl Pts',(102.311013874883,-10.8400383845624,6.77145349076979));
#57062=CARTESIAN_POINT('Ctrl Pts',(102.2639220738,-9.57180236425365,8.46992408797814));
#57063=CARTESIAN_POINT('Ctrl Pts',(102.216830272717,-7.97884246651973,9.77074379488302));
#57064=CARTESIAN_POINT('Ctrl Pts',(102.169738471634,-6.3858825687858,11.0715635017879));
#57065=CARTESIAN_POINT('Ctrl Pts',(102.122646670551,-4.46819879362666,11.9747323183893));
#57066=CARTESIAN_POINT('Ctrl Pts',(102.075554869468,-2.45077316154458,12.3742907805432));
#57067=CARTESIAN_POINT('Ctrl Pts',(102.028463068385,-0.433347529462455,
12.7738492426971));
#57068=CARTESIAN_POINT('Ctrl Pts',(101.981371267302,1.68381995954259,12.6697973504035));
#57069=CARTESIAN_POINT('Ctrl Pts',(101.934279466219,3.65234392223479,12.0743424369403));
#57070=CARTESIAN_POINT('Ctrl Pts',(101.887187665135,5.62086788492697,11.4788875234772));
#57071=CARTESIAN_POINT('Ctrl Pts',(101.840095864052,7.44074832130627,10.3920295888446));
#57072=CARTESIAN_POINT('Ctrl Pts',(101.793004062969,8.89847746593561,8.94127844321045));
#57073=CARTESIAN_POINT('Ctrl Pts',(101.745912261886,10.3562066105649,7.49052729757627));
#57074=CARTESIAN_POINT('Ctrl Pts',(101.698820460803,11.4517844634443,5.6758829409405));
#57075=CARTESIAN_POINT('Ctrl Pts',(101.65172865972,12.0566781965073,3.71023884361215));
#57076=CARTESIAN_POINT('Ctrl Pts',(101.604636858637,12.6615719295703,1.74459474628381));
#57077=CARTESIAN_POINT('Ctrl Pts',(101.557545057554,12.7757815428169,-0.372049091737104));
#57078=CARTESIAN_POINT('Ctrl Pts',(101.510453256471,12.3859080025369,-2.39136872177345));
#57079=CARTESIAN_POINT('Ctrl Pts',(101.463361455388,11.9960344622568,-4.4106883518098));
#57080=CARTESIAN_POINT('Ctrl Pts',(101.416269654305,11.1020777684501,-6.33268377386159));
#57081=CARTESIAN_POINT('Ctrl Pts',(101.369177853222,9.80891662208894,-7.93186712645206));
#57082=CARTESIAN_POINT('Ctrl Pts',(101.322086052139,8.51575547572777,-9.53105047904253));
#57083=CARTESIAN_POINT('Ctrl Pts',(101.274994251056,6.82338987681213,-10.8074217621717));
#57084=CARTESIAN_POINT('Ctrl Pts',(101.227902449973,4.9303675926041,-11.6112375228734));
#57085=CARTESIAN_POINT('Ctrl Pts',(101.202182808648,3.89647521538113,-12.0502492527479));
#57086=CARTESIAN_POINT('Ctrl Pts',(101.176463167323,2.80272888387535,-12.3483022271529));
#57087=CARTESIAN_POINT('Ctrl Pts',(101.150743525999,1.68914515608859,-12.4990650577849));
#57088=CARTESIAN_POINT('',(102.965029240284,1.68935314531922,-12.5));
#57089=CARTESIAN_POINT('Ctrl Pts',(102.965029240284,1.68902555333161,-12.4996661638321));
#57090=CARTESIAN_POINT('Ctrl Pts',(102.965531145447,1.67984017954619,-12.4996740615437));
#57091=CARTESIAN_POINT('Ctrl Pts',(102.966027316753,1.67065452637564,-12.4996820065689));
#57092=CARTESIAN_POINT('Ctrl Pts',(102.966517749822,1.6614685785147,-12.4996899968223));
#57093=CARTESIAN_POINT('Ctrl Pts',(102.97959948863,1.41644397031431,-12.4999031276523));
#57094=CARTESIAN_POINT('Ctrl Pts',(102.988581019146,1.17153336884166,-12.5001505770197));
#57095=CARTESIAN_POINT('Ctrl Pts',(102.993412848414,0.926436831441823,-12.5003783882217));
#57096=CARTESIAN_POINT('Ctrl Pts',(102.995613656082,0.814799952495679,-12.5004821519544));
#57097=CARTESIAN_POINT('Ctrl Pts',(102.996953553553,0.703123817408969,-12.5005815543068));
#57098=CARTESIAN_POINT('Ctrl Pts',(102.997427863959,0.591377000343097,-12.5006697352989));
#57099=CARTESIAN_POINT('Ctrl Pts',(102.998180844966,0.413975809754343,-12.5008097250847));
#57100=CARTESIAN_POINT('Ctrl Pts',(102.996751289823,0.236657100233925,-12.5009214411543));
#57101=CARTESIAN_POINT('Ctrl Pts',(102.993139682215,0.059297357029078,-12.5009714974348));
#57102=CARTESIAN_POINT('Ctrl Pts',(102.992870383431,0.0460725639711593,
-12.5009752298711));
#57103=CARTESIAN_POINT('Ctrl Pts',(102.992588963242,0.0328480636202189,
-12.5009786160395));
#57104=CARTESIAN_POINT('Ctrl Pts',(102.992295424718,0.0196238049059938,
-12.5009816405923));
#57105=CARTESIAN_POINT('Ctrl Pts',(102.992214772671,0.0159903345173654,
-12.5009824716123));
#57106=CARTESIAN_POINT('Ctrl Pts',(102.992133205864,0.0123568858355826,
-12.5009832753311));
#57107=CARTESIAN_POINT('Ctrl Pts',(102.992050724368,0.00872345786128001,
-12.5009840514279));
#57108=CARTESIAN_POINT('Ctrl Pts',(102.992002271108,0.00658902237049392,
-12.5009845073413));
#57109=CARTESIAN_POINT('Ctrl Pts',(102.991953502206,0.00445459441415752,
-12.5009849537224));
#57110=CARTESIAN_POINT('Ctrl Pts',(102.991904417675,0.00232017372424163,
-12.5009853905061));
#57111=CARTESIAN_POINT('Ctrl Pts',(102.991862039437,0.00047737344895807,
-12.5009857676132));
#57112=CARTESIAN_POINT('Ctrl Pts',(102.991819425932,-0.00136542115994614,
-12.5009861375661));
#57113=CARTESIAN_POINT('Ctrl Pts',(102.991776577169,-0.00320821022753773,
-12.5009865003228));
#57114=CARTESIAN_POINT('Ctrl Pts',(102.991724393489,-0.00545246436304751,
-12.5009869421087));
#57115=CARTESIAN_POINT('Ctrl Pts',(102.991671860887,-0.00769670997883713,
-12.5009873732213));
#57116=CARTESIAN_POINT('Ctrl Pts',(102.991618979382,-0.00994094727719665,
-12.5009877935844));
#57117=CARTESIAN_POINT('Ctrl Pts',(102.991519210876,-0.0141750211869177,
-12.5009885866594));
#57118=CARTESIAN_POINT('Ctrl Pts',(102.991418200513,-0.0184090638530525,
-12.5009893414724));
#57119=CARTESIAN_POINT('Ctrl Pts',(102.991315948412,-0.0226430769711849,
-12.5009900575103));
#57120=CARTESIAN_POINT('Ctrl Pts',(102.990733516431,-0.0467601819948663,
-12.5009941360904));
#57121=CARTESIAN_POINT('Ctrl Pts',(102.990110802628,-0.070876071614745,
-12.5009969567622));
#57122=CARTESIAN_POINT('Ctrl Pts',(102.989447831597,-0.0949910545696576,
-12.5009984234356));
#57123=CARTESIAN_POINT('Ctrl Pts',(102.989115137014,-0.107092524834283,
-12.5009991594471));
#57124=CARTESIAN_POINT('Ctrl Pts',(102.988772307999,-0.119193642114226,
-12.5009995544426));
#57125=CARTESIAN_POINT('Ctrl Pts',(102.98841934829,-0.131294445324536,-12.5009995960793));
#57126=CARTESIAN_POINT('Ctrl Pts',(102.98787302245,-0.15002457604026,-12.5009996605264));
#57127=CARTESIAN_POINT('Ctrl Pts',(102.987302425348,-0.168753954322204,
-12.5009988784369));
#57128=CARTESIAN_POINT('Ctrl Pts',(102.986707570848,-0.187482725158803,
-12.5009972959589));
#57129=CARTESIAN_POINT('Ctrl Pts',(102.981885774851,-0.33929516374844,-12.5009844686436));
#57130=CARTESIAN_POINT('Ctrl Pts',(102.975472191106,-0.491003527350138,
-12.5009193887239));
#57131=CARTESIAN_POINT('Ctrl Pts',(102.967478316743,-0.642683527375726,
-12.5008245034654));
#57132=CARTESIAN_POINT('Ctrl Pts',(102.954945096181,-0.880495483007408,
-12.5006757373205));
#57133=CARTESIAN_POINT('Ctrl Pts',(102.938548479827,-1.11782828523526,-12.5004559196816));
#57134=CARTESIAN_POINT('Ctrl Pts',(102.91837476894,-1.35495512994139,-12.5002302445128));
#57135=CARTESIAN_POINT('Ctrl Pts',(102.908897314919,-1.46635549550954,-12.5001242240564));
#57136=CARTESIAN_POINT('Ctrl Pts',(102.898586237988,-1.57770974440371,-12.5000166025227));
#57137=CARTESIAN_POINT('Ctrl Pts',(102.887450486329,-1.68904238362393,-12.4999128886011));
#57138=CARTESIAN_POINT('',(104.701736200614,-1.68935314531934,-12.5));
#57139=CARTESIAN_POINT('Ctrl Pts',(104.701736200614,-1.68908803070059,-12.4991653468105));
#57140=CARTESIAN_POINT('Ctrl Pts',(104.673994843061,-2.89014759230633,-12.336307880009));
#57141=CARTESIAN_POINT('Ctrl Pts',(104.646253485507,-4.0681811144386,-12.0019612113943));
#57142=CARTESIAN_POINT('Ctrl Pts',(104.618512127953,-5.17315215756407,-11.5051231269621));
#57143=CARTESIAN_POINT('Ctrl Pts',(104.57142032687,-7.04887422576513,-10.6617253156888));
#57144=CARTESIAN_POINT('Ctrl Pts',(104.524328525787,-8.71405873387556,-9.35009063801111));
#57145=CARTESIAN_POINT('Ctrl Pts',(104.477236724704,-9.97334679080258,-7.72409963693427));
#57146=CARTESIAN_POINT('Ctrl Pts',(104.430144923621,-11.2326348477296,-6.09810863585747));
#57147=CARTESIAN_POINT('Ctrl Pts',(104.383053122538,-12.0860264534732,-4.15776131138159));
#57148=CARTESIAN_POINT('Ctrl Pts',(104.335961321455,-12.4334019898144,-2.13069856387849));
#57149=CARTESIAN_POINT('Ctrl Pts',(104.288869520372,-12.7807775261557,-0.103635816375385));
#57150=CARTESIAN_POINT('Ctrl Pts',(104.241777719289,-12.6221369930946,2.01014235415493));
#57151=CARTESIAN_POINT('Ctrl Pts',(104.194685918206,-11.9760920449493,3.9626481981061));
#57152=CARTESIAN_POINT('Ctrl Pts',(104.147594117122,-11.330047096804,5.9151540420573));
#57153=CARTESIAN_POINT('Ctrl Pts',(104.100502316039,-10.1965977335744,7.70638755942933));
#57154=CARTESIAN_POINT('Ctrl Pts',(104.053410514956,-8.70871985631894,9.12620183180236));
#57155=CARTESIAN_POINT('Ctrl Pts',(104.006318713873,-7.2208419790635,10.5460161041754));
#57156=CARTESIAN_POINT('Ctrl Pts',(103.95922691279,-5.37853558778224,11.5944111315494));
#57157=CARTESIAN_POINT('Ctrl Pts',(103.912135111707,-3.39793945343931,12.1483895591806));
#57158=CARTESIAN_POINT('Ctrl Pts',(103.865043310624,-1.41734331909643,12.7023679868117));
#57159=CARTESIAN_POINT('Ctrl Pts',(103.817951509541,0.701542558308156,12.7619298147));
#57160=CARTESIAN_POINT('Ctrl Pts',(103.770859708458,2.71013119477651,12.3200872690847));
#57161=CARTESIAN_POINT('Ctrl Pts',(103.723767907375,4.71871983124487,11.8782447234694));
#57162=CARTESIAN_POINT('Ctrl Pts',(103.676676106292,6.61701122677704,10.9349978043505));
#57163=CARTESIAN_POINT('Ctrl Pts',(103.629584305209,8.18229846838074,9.60100792547948));
#57164=CARTESIAN_POINT('Ctrl Pts',(103.582492504126,9.74758570998446,8.26701804660844));
#57165=CARTESIAN_POINT('Ctrl Pts',(103.535400703043,10.9798687976597,6.54228520798529));
#57166=CARTESIAN_POINT('Ctrl Pts',(103.48830890196,11.7345766908152,4.62915449063459));
#57167=CARTESIAN_POINT('Ctrl Pts',(103.441217100877,12.4892845839708,2.7160237732839));
#57168=CARTESIAN_POINT('Ctrl Pts',(103.394125299794,12.7664172826066,0.61449517720567));
#57169=CARTESIAN_POINT('Ctrl Pts',(103.34703349871,12.5334616710087,-1.4288806640642));
#57170=CARTESIAN_POINT('Ctrl Pts',(103.299941697627,12.3005060594108,-3.47225650533403));
#57171=CARTESIAN_POINT('Ctrl Pts',(103.252849896544,11.5574621375793,-5.4574795917955));
#57172=CARTESIAN_POINT('Ctrl Pts',(103.205758095461,10.3915035704427,-7.15164421348415));
#57173=CARTESIAN_POINT('Ctrl Pts',(103.158666294378,9.22554500330613,-8.84580883517282));
#57174=CARTESIAN_POINT('Ctrl Pts',(103.111574493295,7.63667179086451,-10.2489149920886));
#57175=CARTESIAN_POINT('Ctrl Pts',(103.064482692212,5.81129000813801,-11.196350738169));
#57176=CARTESIAN_POINT('Ctrl Pts',(103.031331541569,4.52627849726565,-11.8633157813431));
#57177=CARTESIAN_POINT('Ctrl Pts',(102.998180390927,3.12406000128176,-12.3044634049023));
#57178=CARTESIAN_POINT('Ctrl Pts',(102.965029240284,1.68902555333143,-12.4996661638321));
#57179=CARTESIAN_POINT('',(104.77931495457,1.68935314531922,-12.5));
#57180=CARTESIAN_POINT('Ctrl Pts',(104.77931495457,1.68919355642484,-12.5005864930275));
#57181=CARTESIAN_POINT('Ctrl Pts',(104.779816859733,1.68001010168838,-12.5005940984057));
#57182=CARTESIAN_POINT('Ctrl Pts',(104.780313031038,1.67082635357051,-12.5006016453638));
#57183=CARTESIAN_POINT('Ctrl Pts',(104.780803464108,1.66164229630986,-12.5006091300974));
#57184=CARTESIAN_POINT('Ctrl Pts',(104.793749705728,1.41920549540073,-12.5008067088801));
#57185=CARTESIAN_POINT('Ctrl Pts',(104.802680236919,1.17687017443894,-12.5009631542608));
#57186=CARTESIAN_POINT('Ctrl Pts',(104.807547086755,0.93433729498524,-12.5009942749996));
#57187=CARTESIAN_POINT('Ctrl Pts',(104.80821046687,0.901278644165153,-12.5009985169384));
#57188=CARTESIAN_POINT('Ctrl Pts',(104.808798346689,0.868216252236512,-12.5010003947653));
#57189=CARTESIAN_POINT('Ctrl Pts',(104.809310604728,0.835149297560743,-12.500999658972));
#57190=CARTESIAN_POINT('Ctrl Pts',(104.810567363188,0.754023825900984,-12.5009978537989));
#57191=CARTESIAN_POINT('Ctrl Pts',(104.811368952344,0.672870923199062,-12.5009803357246));
#57192=CARTESIAN_POINT('Ctrl Pts',(104.811713578245,0.59167861130207,-12.5009506355434));
#57193=CARTESIAN_POINT('Ctrl Pts',(104.812466559252,0.414279673417628,-12.5008857429387));
#57194=CARTESIAN_POINT('Ctrl Pts',(104.811037004109,0.23695338523688,-12.5007631174331));
#57195=CARTESIAN_POINT('Ctrl Pts',(104.807425396501,0.059578059847195,-12.5006153254265));
#57196=CARTESIAN_POINT('Ctrl Pts',(104.807156097717,0.0463521049043557,
-12.5006043053457));
#57197=CARTESIAN_POINT('Ctrl Pts',(104.806874677527,0.0331263982138967,
-12.5005931427019));
#57198=CARTESIAN_POINT('Ctrl Pts',(104.806581139004,0.0199008894796828,
-12.5005818495349));
#57199=CARTESIAN_POINT('Ctrl Pts',(104.806500486957,0.0162670756548309,
-12.5005787466474));
#57200=CARTESIAN_POINT('Ctrl Pts',(104.806418920151,0.0126332802390204,
-12.5005756339081));
#57201=CARTESIAN_POINT('Ctrl Pts',(104.806336438654,0.00899950219642152,
-12.500572511564));
#57202=CARTESIAN_POINT('Ctrl Pts',(104.806287985393,0.00686486105990187,
-12.5005706773617));
#57203=CARTESIAN_POINT('Ctrl Pts',(104.80623921649,0.0047302263253564,-12.5005688398452));
#57204=CARTESIAN_POINT('Ctrl Pts',(104.80619013196,0.00259559779005463,
-12.5005669990643));
#57205=CARTESIAN_POINT('Ctrl Pts',(104.806147753723,0.000752618029680907,
-12.5005654097846));
#57206=CARTESIAN_POINT('Ctrl Pts',(104.806105140217,-0.00109035690604705,
-12.5005638180718));
#57207=CARTESIAN_POINT('Ctrl Pts',(104.806062291454,-0.0029333271355872,
-12.500562223958));
#57208=CARTESIAN_POINT('Ctrl Pts',(104.806010107776,-0.00517780184503334,
-12.5005602825548));
#57209=CARTESIAN_POINT('Ctrl Pts',(104.805957575176,-0.00742226928008383,
-12.5005583375906));
#57210=CARTESIAN_POINT('Ctrl Pts',(104.805904693668,-0.00966672981599251,
-12.5005563891231));
#57211=CARTESIAN_POINT('Ctrl Pts',(104.805804925161,-0.0139012246850115,
-12.5005527130612));
#57212=CARTESIAN_POINT('Ctrl Pts',(104.805703914798,-0.0181356927295366,
-12.5005490245313));
#57213=CARTESIAN_POINT('Ctrl Pts',(104.805601662698,-0.0223701355818334,
-12.5005453239189));
#57214=CARTESIAN_POINT('Ctrl Pts',(104.805019230717,-0.0464896885183316,
-12.5005242450852));
#57215=CARTESIAN_POINT('Ctrl Pts',(104.804396516915,-0.0706081685829107,
-12.5005027746528));
#57216=CARTESIAN_POINT('Ctrl Pts',(104.803733545885,-0.0947258798446518,
-12.5004809824714));
#57217=CARTESIAN_POINT('Ctrl Pts',(104.802885892622,-0.125562003504238,
-12.5004531196947));
#57218=CARTESIAN_POINT('Ctrl Pts',(104.801972451701,-0.156396061231039,
-12.5004247318868));
#57219=CARTESIAN_POINT('Ctrl Pts',(104.800993284962,-0.187228686091773,
-12.5003959593782));
#57220=CARTESIAN_POINT('Ctrl Pts',(104.796171488701,-0.339060472613246,
-12.500254272402));
#57221=CARTESIAN_POINT('Ctrl Pts',(104.789757904542,-0.490793335817318,
-12.5001036262456));
#57222=CARTESIAN_POINT('Ctrl Pts',(104.781764029618,-0.642501306198806,
-12.4999584778234));
#57223=CARTESIAN_POINT('Ctrl Pts',(104.76917486863,-0.881418737418034,-12.4997298907024));
#57224=CARTESIAN_POINT('Ctrl Pts',(104.752687747525,-1.11986127288837,-12.4995172107899));
#57225=CARTESIAN_POINT('Ctrl Pts',(104.732390128302,-1.35809925406382,-12.4993555671229));
#57226=CARTESIAN_POINT('Ctrl Pts',(104.722987028528,-1.46846567106078,-12.499280683881));
#57227=CARTESIAN_POINT('Ctrl Pts',(104.712766154114,-1.57878753286359,-12.4992164728357));
#57228=CARTESIAN_POINT('Ctrl Pts',(104.701736200614,-1.68908803070068,-12.4991653468104));
#57229=CARTESIAN_POINT('',(106.5160219149,-1.68935314531935,-12.5));
#57230=CARTESIAN_POINT('Ctrl Pts',(106.5160219149,-1.68934693203252,-12.4990807809333));
#57231=CARTESIAN_POINT('Ctrl Pts',(106.495712066664,-2.56876383854141,-12.3805352414928));
#57232=CARTESIAN_POINT('Ctrl Pts',(106.475402218428,-3.43570307962652,-12.1701285355112));
#57233=CARTESIAN_POINT('Ctrl Pts',(106.455092370193,-4.27031533948596,-11.8698673364697));
#57234=CARTESIAN_POINT('Ctrl Pts',(106.40800056911,-6.2055043210297,-11.1736612154764));
#57235=CARTESIAN_POINT('Ctrl Pts',(106.360908768026,-7.96689625422667,-9.99437733459268));
#57236=CARTESIAN_POINT('Ctrl Pts',(106.313816966943,-9.34784984467607,-8.47036389403563));
#57237=CARTESIAN_POINT('Ctrl Pts',(106.26672516586,-10.7288034351255,-6.94635045347851));
#57238=CARTESIAN_POINT('Ctrl Pts',(106.219633364777,-11.7293186828274,-5.07760745324805));
#57239=CARTESIAN_POINT('Ctrl Pts',(106.172541563694,-12.2320132550129,-3.08337759474184));
#57240=CARTESIAN_POINT('Ctrl Pts',(106.125449762611,-12.7347078271983,-1.08914773623572));
#57241=CARTESIAN_POINT('Ctrl Pts',(106.078357961528,-12.7395817238675,1.03056898054615));
#57242=CARTESIAN_POINT('Ctrl Pts',(106.031266160445,-12.2460642058922,3.02708924830187));
#57243=CARTESIAN_POINT('Ctrl Pts',(105.984174359362,-11.7525466879169,5.02360951605759));
#57244=CARTESIAN_POINT('Ctrl Pts',(105.937082558279,-10.7606377552971,6.89693333478716));
#57245=CARTESIAN_POINT('Ctrl Pts',(105.889990757196,-9.38670732174682,8.42728242690899));
#57246=CARTESIAN_POINT('Ctrl Pts',(105.842898956113,-8.01277688819656,9.95763151903081));
#57247=CARTESIAN_POINT('Ctrl Pts',(105.79580715503,-6.25682495371582,11.1450058845449));
#57248=CARTESIAN_POINT('Ctrl Pts',(105.748715353947,-4.32485945868025,11.850103424355));
#57249=CARTESIAN_POINT('Ctrl Pts',(105.701623552864,-2.39289396364465,12.5552009641652));
#57250=CARTESIAN_POINT('Ctrl Pts',(105.654531751781,-0.284914908054215,
12.7780216782715));
#57251=CARTESIAN_POINT('Ctrl Pts',(105.607439950697,1.7517704266388,12.4924241875336));
#57252=CARTESIAN_POINT('Ctrl Pts',(105.560348149614,3.78845576133182,12.2068266967957));
#57253=CARTESIAN_POINT('Ctrl Pts',(105.513256348531,5.75384737512741,11.4128110012137));
#57254=CARTESIAN_POINT('Ctrl Pts',(105.466164547448,7.41736612323887,10.2035308183321));
#57255=CARTESIAN_POINT('Ctrl Pts',(105.419072746365,9.08088487135031,8.9942506354505));
#57256=CARTESIAN_POINT('Ctrl Pts',(105.371980945282,10.4425307537776,7.36970596526928));
#57257=CARTESIAN_POINT('Ctrl Pts',(105.324889144199,11.3425559571878,5.52048781697627));
#57258=CARTESIAN_POINT('Ctrl Pts',(105.277797343116,12.2425811605979,3.67126966868326));
#57259=CARTESIAN_POINT('Ctrl Pts',(105.230705542033,12.6809856849908,1.59737804227846));
#57260=CARTESIAN_POINT('Ctrl Pts',(105.18361374095,12.6063360448345,-0.457878774668838));
#57261=CARTESIAN_POINT('Ctrl Pts',(105.136521939867,12.5316864046781,-2.51313559161616));
#57262=CARTESIAN_POINT('Ctrl Pts',(105.089430138784,11.9439825999724,-4.54975759910599));
#57263=CARTESIAN_POINT('Ctrl Pts',(105.042338337701,10.9121738512091,-6.32880898967823));
#57264=CARTESIAN_POINT('Ctrl Pts',(104.995246536618,9.88036510244591,-8.10786038025044));
#57265=CARTESIAN_POINT('Ctrl Pts',(104.948154735535,8.40445140962515,-9.62934115390508));
#57266=CARTESIAN_POINT('Ctrl Pts',(104.901062934452,6.65758647161741,-10.7147516908012));
#57267=CARTESIAN_POINT('Ctrl Pts',(104.860480274491,5.15217737394656,-11.6501341931341));
#57268=CARTESIAN_POINT('Ctrl Pts',(104.81989761453,3.44554344694001,-12.2616644876296));
#57269=CARTESIAN_POINT('Ctrl Pts',(104.77931495457,1.6891935564243,-12.5005864930276));
#57270=CARTESIAN_POINT('',(106.593600668856,1.68935314531922,-12.5));
#57271=CARTESIAN_POINT('Ctrl Pts',(106.593600668856,1.68952807354336,-12.5009853194712));
#57272=CARTESIAN_POINT('Ctrl Pts',(106.594102574019,1.68034421904941,-12.5009832688272));
#57273=CARTESIAN_POINT('Ctrl Pts',(106.594598745324,1.67116003522182,-12.5009810445824));
#57274=CARTESIAN_POINT('Ctrl Pts',(106.595089178393,1.66197550718774,-12.500978651551));
#57275=CARTESIAN_POINT('Ctrl Pts',(106.608363594638,1.41338042703455,-12.50091388003));
#57276=CARTESIAN_POINT('Ctrl Pts',(106.617416131364,1.1648664983038,-12.5007274931519));
#57277=CARTESIAN_POINT('Ctrl Pts',(106.622195076342,0.916129042150179,-12.5005048281007));
#57278=CARTESIAN_POINT('Ctrl Pts',(106.624270835107,0.808088678176874,-12.5004081124168));
#57279=CARTESIAN_POINT('Ctrl Pts',(106.625540319729,0.70000547944534,-12.5003043542637));
#57280=CARTESIAN_POINT('Ctrl Pts',(106.625999292531,0.59185171030578,-12.5001993366535));
#57281=CARTESIAN_POINT('Ctrl Pts',(106.626752273537,0.41441693946698,-12.5000270469983));
#57282=CARTESIAN_POINT('Ctrl Pts',(106.625322718394,0.237052919580531,-12.4998518560448));
#57283=CARTESIAN_POINT('Ctrl Pts',(106.621711110787,0.0596396457159169,
-12.49969399153));
#57284=CARTESIAN_POINT('Ctrl Pts',(106.621441812002,0.0464108611478938,
-12.4996822203947));
#57285=CARTESIAN_POINT('Ctrl Pts',(106.621160391813,0.0331823237433037,
-12.4996705429826));
#57286=CARTESIAN_POINT('Ctrl Pts',(106.620866853289,0.0199539839213671,
-12.4996589661652));
#57287=CARTESIAN_POINT('Ctrl Pts',(106.620786201243,0.0163193922582425,
-12.4996557853424));
#57288=CARTESIAN_POINT('Ctrl Pts',(106.620704634438,0.0126848189755927,
-12.4996526121156));
#57289=CARTESIAN_POINT('Ctrl Pts',(106.62062215294,0.00905026296460605,
-12.4996494466242));
#57290=CARTESIAN_POINT('Ctrl Pts',(106.620573699678,0.00691516480986947,
-12.4996475870753));
#57291=CARTESIAN_POINT('Ctrl Pts',(106.620524930774,0.00478007305231262,
-12.4996457301962));
#57292=CARTESIAN_POINT('Ctrl Pts',(106.620475846246,0.00264498761126058,
-12.4996438760151));
#57293=CARTESIAN_POINT('Ctrl Pts',(106.620433468009,0.000801613303429549,
-12.4996422751659));
#57294=CARTESIAN_POINT('Ctrl Pts',(106.620390854503,-0.00104175618109215,
-12.499640676328));
#57295=CARTESIAN_POINT('Ctrl Pts',(106.62034800574,-0.00288512096233046,
-12.4996390795193));
#57296=CARTESIAN_POINT('Ctrl Pts',(106.620295822061,-0.00513007619243232,
-12.4996371348342));
#57297=CARTESIAN_POINT('Ctrl Pts',(106.620243289461,-0.00737502414715744,
-12.4996351931592));
#57298=CARTESIAN_POINT('Ctrl Pts',(106.620190407953,-0.0096199651517339,
-12.4996332545265));
#57299=CARTESIAN_POINT('Ctrl Pts',(106.620090639447,-0.0138553665431028,
-12.4996295970193));
#57300=CARTESIAN_POINT('Ctrl Pts',(106.619989629084,-0.0180907410943302,
-12.4996259503431));
#57301=CARTESIAN_POINT('Ctrl Pts',(106.619887376984,-0.0223260904432372,
-12.4996223147132));
#57302=CARTESIAN_POINT('Ctrl Pts',(106.619304945002,-0.0464508067240482,
-12.4996016060229));
#57303=CARTESIAN_POINT('Ctrl Pts',(106.618682231199,-0.07057444882255,-12.4995812561438));
#57304=CARTESIAN_POINT('Ctrl Pts',(106.618019260169,-0.0946973165648927,
-12.4995613035175));
#57305=CARTESIAN_POINT('Ctrl Pts',(106.617171606944,-0.125540031735592,
-12.4995357927375));
#57306=CARTESIAN_POINT('Ctrl Pts',(106.616258166066,-0.156380671725298,
-12.4995109322356));
#57307=CARTESIAN_POINT('Ctrl Pts',(106.615278999377,-0.187219860747437,
-12.499486796637));
#57308=CARTESIAN_POINT('Ctrl Pts',(106.610457203316,-0.339083973146112,
-12.4993679436004));
#57309=CARTESIAN_POINT('Ctrl Pts',(106.604043619468,-0.490848708425859,
-12.4992670176415));
#57310=CARTESIAN_POINT('Ctrl Pts',(106.596049744968,-0.642587048357201,
-12.4991906401119));
#57311=CARTESIAN_POINT('Ctrl Pts',(106.583417868099,-0.882363145197298,
-12.4990699487565));
#57312=CARTESIAN_POINT('Ctrl Pts',(106.566861534007,-1.12165729659649,-12.4990125535785));
#57313=CARTESIAN_POINT('Ctrl Pts',(106.546469098015,-1.36073855108457,-12.4990236220852));
#57314=CARTESIAN_POINT('Ctrl Pts',(106.537122978201,-1.47031261327066,-12.4990286949264));
#57315=CARTESIAN_POINT('Ctrl Pts',(106.526971081869,-1.57984130388627,-12.4990478927983));
#57316=CARTESIAN_POINT('Ctrl Pts',(106.5160219149,-1.68934693203216,-12.4990807809333));
#57317=CARTESIAN_POINT('',(107.444020192937,0.782909338907702,12.5893195613048));
#57318=CARTESIAN_POINT('Ctrl Pts',(107.444020192937,0.782909338906896,12.5893195613048));
#57319=CARTESIAN_POINT('Ctrl Pts',(107.396928391854,2.83606438077655,12.4616371835023));
#57320=CARTESIAN_POINT('Ctrl Pts',(107.349836590771,4.85644362728424,11.8222740696369));
#57321=CARTESIAN_POINT('Ctrl Pts',(107.302744789688,6.60816901018162,10.7451655348056));
#57322=CARTESIAN_POINT('Ctrl Pts',(107.255652988605,8.35989439307901,9.66805699997423));
#57323=CARTESIAN_POINT('Ctrl Pts',(107.208561187522,9.84296591236608,8.15320304417694));
#57324=CARTESIAN_POINT('Ctrl Pts',(107.161469386439,10.8829918506863,6.37887339924185));
#57325=CARTESIAN_POINT('Ctrl Pts',(107.114377585355,11.9230177890065,4.60454375430671));
#57326=CARTESIAN_POINT('Ctrl Pts',(107.067285784272,12.5199981463597,2.57073842023375));
#57327=CARTESIAN_POINT('Ctrl Pts',(107.020193983189,12.6040774571683,0.515871141998574));
#57328=CARTESIAN_POINT('Ctrl Pts',(106.973102182106,12.6881567679768,-1.53899613623655));
#57329=CARTESIAN_POINT('Ctrl Pts',(106.926010381023,12.2593350322407,-3.61492535863389));
#57330=CARTESIAN_POINT('Ctrl Pts',(106.87891857994,11.3678344699642,-5.46827444689482));
#57331=CARTESIAN_POINT('Ctrl Pts',(106.831826778857,10.4763339076878,-7.32162353515575));
#57332=CARTESIAN_POINT('Ctrl Pts',(106.784734977774,9.12215451887095,-8.95239248928027));
#57333=CARTESIAN_POINT('Ctrl Pts',(106.737643176691,7.46420991976001,-10.1693050890532));
#57334=CARTESIAN_POINT('Ctrl Pts',(106.690551375608,5.80626532064906,-11.3862176888261));
#57335=CARTESIAN_POINT('Ctrl Pts',(106.643459574525,3.84455551124398,-12.1892739342474));
#57336=CARTESIAN_POINT('Ctrl Pts',(106.596367773442,1.80920759159618,-12.4842378764066));
#57337=CARTESIAN_POINT('Ctrl Pts',(106.595445405246,1.76934204930534,-12.4900152166819));
#57338=CARTESIAN_POINT('Ctrl Pts',(106.594523037051,1.7294482568701,-12.4955976350495));
#57339=CARTESIAN_POINT('Ctrl Pts',(106.593600668856,1.68952807354336,-12.5009853194712));
#57340=CARTESIAN_POINT('Ctrl Pts',(108.008153428708,1.61683638546961,11.4839173606684));
#57341=CARTESIAN_POINT('Ctrl Pts',(107.966031738243,1.57797833705833,11.5652727241384));
#57342=CARTESIAN_POINT('Ctrl Pts',(107.924174837091,1.5363367640964,11.6463102940928));
#57343=CARTESIAN_POINT('Ctrl Pts',(107.883039431048,1.49176115295735,11.7261593831322));
#57344=CARTESIAN_POINT('Ctrl Pts',(107.843254818669,1.44864930403286,11.8033864087513));
#57345=CARTESIAN_POINT('Ctrl Pts',(107.804145094866,1.40279277474693,11.8795015989354));
#57346=CARTESIAN_POINT('Ctrl Pts',(107.766123435132,1.35410262839987,11.9537045620535));
#57347=CARTESIAN_POINT('Ctrl Pts',(107.751995478605,1.33601051259738,11.9812766418754));
#57348=CARTESIAN_POINT('Ctrl Pts',(107.738017750126,1.31752765476251,12.0085845828291));
#57349=CARTESIAN_POINT('Ctrl Pts',(107.72421144694,1.2986513057777,12.0355869118102));
#57350=CARTESIAN_POINT('Ctrl Pts',(107.693743691972,1.2569949718699,12.0951756613734));
#57351=CARTESIAN_POINT('Ctrl Pts',(107.663609982109,1.21276627861128,12.1542515643353));
#57352=CARTESIAN_POINT('Ctrl Pts',(107.634283495276,1.16587466320814,12.2119162262066));
#57353=CARTESIAN_POINT('Ctrl Pts',(107.60566926689,1.120121914161,12.2681803745155));
#57354=CARTESIAN_POINT('Ctrl Pts',(107.577823527304,1.07183375384895,12.3231008875987));
#57355=CARTESIAN_POINT('Ctrl Pts',(107.55118580849,1.02097382111972,12.3758332678361));
#57356=CARTESIAN_POINT('Ctrl Pts',(107.525353444986,0.971651569493986,12.4269713560586));
#57357=CARTESIAN_POINT('Ctrl Pts',(107.500657160734,0.919910564744948,12.4760514858375));
#57358=CARTESIAN_POINT('Ctrl Pts',(107.477497814894,0.865765955833377,12.5222957773865));
#57359=CARTESIAN_POINT('Ctrl Pts',(107.465939154467,0.838742776824957,12.5453759656779));
#57360=CARTESIAN_POINT('Ctrl Pts',(107.454763335443,0.811121652850066,12.5677496555355));
#57361=CARTESIAN_POINT('Ctrl Pts',(107.444020192937,0.782909338907791,12.5893195613048));
#57362=CARTESIAN_POINT('',(96.446025,7.1032002856509,-9.1678677603644));
#57363=CARTESIAN_POINT('Ctrl Pts',(96.446025,7.1032002856509,-9.1678677603644));
#57364=CARTESIAN_POINT('Ctrl Pts',(96.4931168010831,8.59836083215431,-8.00942775025295));
#57365=CARTESIAN_POINT('Ctrl Pts',(96.5873004032492,11.0098238737483,-4.94829702622741));
#57366=CARTESIAN_POINT('Ctrl Pts',(96.7285758064984,12.0436316920041,0.807234573314296));
#57367=CARTESIAN_POINT('Ctrl Pts',(96.8698512097476,10.2513621865474,6.37239418233372));
#57368=CARTESIAN_POINT('Ctrl Pts',(97.0111266129968,6.05378860029595,10.4428153879447));
#57369=CARTESIAN_POINT('Ctrl Pts',(97.152402016246,0.435723763467222,12.0627151308176));
#57370=CARTESIAN_POINT('Ctrl Pts',(97.2936774194952,-5.28456262813498,10.8523362109951));
#57371=CARTESIAN_POINT('Ctrl Pts',(97.4349528227444,-9.76489064575089,7.09552016347875));
#57372=CARTESIAN_POINT('Ctrl Pts',(97.5425267380375,-11.4317746886518,2.9671918442554));
#57373=CARTESIAN_POINT('Ctrl Pts',(97.6030088522475,-11.5978336888622,0.538110614070643));
#57374=CARTESIAN_POINT('Ctrl Pts',(97.6163991653745,-11.5973549676912,0.00026415572522899));
#57375=CARTESIAN_POINT('',(96.446025,5.49758084898117,11.3528330610334));
#57376=CARTESIAN_POINT('Ctrl Pts',(96.446025,5.4978005759398,11.3530041107288));
#57377=CARTESIAN_POINT('Ctrl Pts',(96.446025,5.75802350928769,11.2143077748595));
#57378=CARTESIAN_POINT('Ctrl Pts',(96.446025,6.01305469750609,11.0665970670471));
#57379=CARTESIAN_POINT('Ctrl Pts',(96.446025,6.26237325434567,10.910023872863));
#57380=CARTESIAN_POINT('Ctrl Pts',(96.446025,6.27759354024327,10.9004654636952));
#57381=CARTESIAN_POINT('Ctrl Pts',(96.446025,6.29279252804283,10.8908740118952));
#57382=CARTESIAN_POINT('Ctrl Pts',(96.446025,6.30797009589712,10.8812495466477));
#57383=CARTESIAN_POINT('Ctrl Pts',(96.446025,6.55734691236906,10.7231136366833));
#57384=CARTESIAN_POINT('Ctrl Pts',(96.446025,6.80094385595134,10.5560686290167));
#57385=CARTESIAN_POINT('Ctrl Pts',(96.446025,7.03838271553362,10.3805320487659));
#57386=CARTESIAN_POINT('Ctrl Pts',(96.446025,7.21294398807995,10.2514803472839));
#57387=CARTESIAN_POINT('Ctrl Pts',(96.446025,7.38417623425726,10.1178380533548));
#57388=CARTESIAN_POINT('Ctrl Pts',(96.446025,7.55191654776048,9.97975830214868));
#57389=CARTESIAN_POINT('Ctrl Pts',(96.446025,7.62992441658677,9.91554411955476));
#57390=CARTESIAN_POINT('Ctrl Pts',(96.446025,7.70717691379675,9.85037009448964));
#57391=CARTESIAN_POINT('Ctrl Pts',(96.446025,7.78365677159635,9.78425093759342));
#57392=CARTESIAN_POINT('Ctrl Pts',(96.446025,7.83453670777231,9.74026368945153));
#57393=CARTESIAN_POINT('Ctrl Pts',(96.446025,7.88507467175993,9.69585812919905));
#57394=CARTESIAN_POINT('Ctrl Pts',(96.446025,7.93526543264948,9.65103849064499));
#57395=CARTESIAN_POINT('Ctrl Pts',(96.446025,7.96671726405787,9.62295245069256));
#57396=CARTESIAN_POINT('Ctrl Pts',(96.446025,7.99802688312031,9.59470901524118));
#57397=CARTESIAN_POINT('Ctrl Pts',(96.446025,8.02918789242708,9.5663142635499));
#57398=CARTESIAN_POINT('Ctrl Pts',(96.446025,8.24626937643572,9.36850376343036));
#57399=CARTESIAN_POINT('Ctrl Pts',(96.446025,8.45622333104263,9.16327984499431));
#57400=CARTESIAN_POINT('Ctrl Pts',(96.446025,8.65868156283819,8.95105692458998));
#57401=CARTESIAN_POINT('Ctrl Pts',(96.446025,8.86053340792298,8.73946963731111));
#57402=CARTESIAN_POINT('Ctrl Pts',(96.446025,9.0549347499723,8.52092472280692));
#57403=CARTESIAN_POINT('Ctrl Pts',(96.446025,9.24148137322108,8.29579970571171));
#57404=CARTESIAN_POINT('Ctrl Pts',(96.446025,9.42654383520758,8.07246577882077));
#57405=CARTESIAN_POINT('Ctrl Pts',(96.446025,9.60387640350412,7.84265555342141));
#57406=CARTESIAN_POINT('Ctrl Pts',(96.446025,9.77304034211128,7.60671216649778));
#57407=CARTESIAN_POINT('Ctrl Pts',(96.446025,9.81546086641513,7.54754564281823));
#57408=CARTESIAN_POINT('Ctrl Pts',(96.446025,9.8573674867971,7.48799333868432));
#57409=CARTESIAN_POINT('Ctrl Pts',(96.446025,9.89875280632189,7.42806046573141));
#57410=CARTESIAN_POINT('Ctrl Pts',(96.446025,9.91788263026291,7.40035727723286));
#57411=CARTESIAN_POINT('Ctrl Pts',(96.446025,9.93689621068264,7.37257979211348));
#57412=CARTESIAN_POINT('Ctrl Pts',(96.446025,9.95579098474034,7.34473162572225));
#57413=CARTESIAN_POINT('Ctrl Pts',(96.446025,10.119018138577,7.10415838966613));
#57414=CARTESIAN_POINT('Ctrl Pts',(96.446025,10.27343184152,6.8582414172292));
#57415=CARTESIAN_POINT('Ctrl Pts',(96.446025,10.4186815916346,6.60737648542902));
#57416=CARTESIAN_POINT('Ctrl Pts',(96.446025,10.437263930765,6.57528240447552));
#57417=CARTESIAN_POINT('Ctrl Pts',(96.446025,10.4556962275322,6.54310729772208));
#57418=CARTESIAN_POINT('Ctrl Pts',(96.446025,10.4739776980424,6.51085195781411));
#57419=CARTESIAN_POINT('Ctrl Pts',(96.446025,10.6166099532034,6.25919540373678));
#57420=CARTESIAN_POINT('Ctrl Pts',(96.446025,10.7500650514451,6.00265698749348));
#57421=CARTESIAN_POINT('Ctrl Pts',(96.446025,10.8742414607825,5.74178192512992));
#57422=CARTESIAN_POINT('Ctrl Pts',(96.446025,10.9989235002189,5.47984461362972));
#57423=CARTESIAN_POINT('Ctrl Pts',(96.446025,11.1142513075349,5.21353465970876));
#57424=CARTESIAN_POINT('Ctrl Pts',(96.446025,11.2200732858474,4.94338427334107));
#57425=CARTESIAN_POINT('Ctrl Pts',(96.446025,11.3256004400896,4.67398653626053));
#57426=CARTESIAN_POINT('Ctrl Pts',(96.446025,11.4216747837927,4.40076911982243));
#57427=CARTESIAN_POINT('Ctrl Pts',(96.446025,11.5080953785583,4.12424946024983));
#57428=CARTESIAN_POINT('Ctrl Pts',(96.446025,11.5919051535307,3.85608363117774));
#57429=CARTESIAN_POINT('Ctrl Pts',(96.446025,11.6666355551521,3.58481151953519));
#57430=CARTESIAN_POINT('Ctrl Pts',(96.446025,11.7320558790342,3.31090391283863));
#57431=CARTESIAN_POINT('Ctrl Pts',(96.446025,11.7470314809477,3.24820273626922));
#57432=CARTESIAN_POINT('Ctrl Pts',(96.446025,11.7615190232195,3.18536347007864));
#57433=CARTESIAN_POINT('Ctrl Pts',(96.446025,11.7755153823783,3.12239179797609));
#57434=CARTESIAN_POINT('Ctrl Pts',(96.446025,11.7841026482886,3.08375642951829));
#57435=CARTESIAN_POINT('Ctrl Pts',(96.446025,11.7925058566515,3.04506702517162));
#57436=CARTESIAN_POINT('Ctrl Pts',(96.446025,11.8007185497336,3.00635254211889));
#57437=CARTESIAN_POINT('Ctrl Pts',(96.446025,11.8603768204461,2.72512455912071));
#57438=CARTESIAN_POINT('Ctrl Pts',(96.446025,11.9100466496312,2.44231213195589));
#57439=CARTESIAN_POINT('Ctrl Pts',(96.446025,11.9496224947969,2.15843752916402));
#57440=CARTESIAN_POINT('Ctrl Pts',(96.446025,11.9891050030404,1.87523242519441));
#57441=CARTESIAN_POINT('Ctrl Pts',(96.446025,12.0185411852995,1.59096953933644));
#57442=CARTESIAN_POINT('Ctrl Pts',(96.446025,12.0377756152134,1.30615747712036));
#57443=CARTESIAN_POINT('Ctrl Pts',(96.446025,12.0489742493925,1.14033472548109));
#57444=CARTESIAN_POINT('Ctrl Pts',(96.446025,12.0567137609233,0.974325676220046));
#57445=CARTESIAN_POINT('Ctrl Pts',(96.446025,12.0609553233804,0.808230381556516));
#57446=CARTESIAN_POINT('Ctrl Pts',(96.446025,12.0682685793829,0.521850675269838));
#57447=CARTESIAN_POINT('Ctrl Pts',(96.446025,12.0651858299839,0.23521395735393));
#57448=CARTESIAN_POINT('Ctrl Pts',(96.446025,12.0518194398101,-0.0511360161595567));
#57449=CARTESIAN_POINT('Ctrl Pts',(96.446025,12.0384958623745,-0.336568806627351));
#57450=CARTESIAN_POINT('Ctrl Pts',(96.446025,12.0149542352207,-0.62171729672152));
#57451=CARTESIAN_POINT('Ctrl Pts',(96.446025,11.981256120355,-0.906029323615214));
#57452=CARTESIAN_POINT('Ctrl Pts',(96.446025,11.9609240474986,-1.0775716448339));
#57453=CARTESIAN_POINT('Ctrl Pts',(96.446025,11.9368936343814,-1.24880915430181));
#57454=CARTESIAN_POINT('Ctrl Pts',(96.446025,11.9091700093926,-1.41961674289046));
#57455=CARTESIAN_POINT('Ctrl Pts',(96.446025,11.9018068261626,-1.46498193493737));
#57456=CARTESIAN_POINT('Ctrl Pts',(96.446025,11.8941830925326,-1.51031678185175));
#57457=CARTESIAN_POINT('Ctrl Pts',(96.446025,11.8862988316856,-1.55561889700612));
#57458=CARTESIAN_POINT('Ctrl Pts',(96.446025,11.8799799710488,-1.59192639085565));
#57459=CARTESIAN_POINT('Ctrl Pts',(96.446025,11.8734931827204,-1.6282157770847));
#57460=CARTESIAN_POINT('Ctrl Pts',(96.446025,11.8668430364879,-1.66446169168796));
#57461=CARTESIAN_POINT('Ctrl Pts',(96.446025,11.8155846022351,-1.94384033475061));
#57462=CARTESIAN_POINT('Ctrl Pts',(96.446025,11.754576219872,-2.22092831643957));
#57463=CARTESIAN_POINT('Ctrl Pts',(96.446025,11.6839893564517,-2.49521102281565));
#57464=CARTESIAN_POINT('Ctrl Pts',(96.446025,11.6133492547656,-2.76970059963333));
#57465=CARTESIAN_POINT('Ctrl Pts',(96.446025,11.5331160419521,-3.04138128031828));
#57466=CARTESIAN_POINT('Ctrl Pts',(96.446025,11.44341031998,-3.30972710363197));
#57467=CARTESIAN_POINT('Ctrl Pts',(96.446025,11.3545530114623,-3.57553498174052));
#57468=CARTESIAN_POINT('Ctrl Pts',(96.446025,11.2564012837368,-3.83807134091528));
#57469=CARTESIAN_POINT('Ctrl Pts',(96.446025,11.149025305932,-4.09680634848039));
#57470=CARTESIAN_POINT('Ctrl Pts',(96.446025,11.0425657924693,-4.35333302776457));
#57471=CARTESIAN_POINT('Ctrl Pts',(96.446025,10.9270386065772,-4.60612349036155));
#57472=CARTESIAN_POINT('Ctrl Pts',(96.446025,10.8024689941292,-4.85463493583518));
#57473=CARTESIAN_POINT('Ctrl Pts',(96.446025,10.6953943412341,-5.06824462957723));
#57474=CARTESIAN_POINT('Ctrl Pts',(96.446025,10.5816377838971,-5.27869247154203));
#57475=CARTESIAN_POINT('Ctrl Pts',(96.446025,10.4613871615161,-5.48570603579521));
#57476=CARTESIAN_POINT('Ctrl Pts',(96.446025,10.4087775142244,-5.57627447015598));
#57477=CARTESIAN_POINT('Ctrl Pts',(96.446025,10.3549246251689,-5.66618531594217));
#57478=CARTESIAN_POINT('Ctrl Pts',(96.446025,10.2998431779684,-5.75541454179228));
#57479=CARTESIAN_POINT('Ctrl Pts',(96.446025,10.2799271554621,-5.78767751527195));
#57480=CARTESIAN_POINT('Ctrl Pts',(96.446025,10.2598505107673,-5.81985136917303));
#57481=CARTESIAN_POINT('Ctrl Pts',(96.446025,10.2396139191792,-5.85193494173057));
#57482=CARTESIAN_POINT('Ctrl Pts',(96.446025,10.22069632276,-5.88192734804515));
#57483=CARTESIAN_POINT('Ctrl Pts',(96.446025,10.2016377782411,-5.91184258810781));
#57484=CARTESIAN_POINT('Ctrl Pts',(96.446025,10.1824512248116,-5.94166071224686));
#57485=CARTESIAN_POINT('Ctrl Pts',(96.446025,10.0316611993092,-6.17600586005514));
#57486=CARTESIAN_POINT('Ctrl Pts',(96.446025,9.872806361262,-6.40461413627334));
#57487=CARTESIAN_POINT('Ctrl Pts',(96.446025,9.70628844661517,-6.62713123184326));
#57488=CARTESIAN_POINT('Ctrl Pts',(96.446025,9.53861194535784,-6.85119654117794));
#57489=CARTESIAN_POINT('Ctrl Pts',(96.446025,9.36316496265846,-7.06908609777102));
#57490=CARTESIAN_POINT('Ctrl Pts',(96.446025,9.18031378687851,-7.28040897935406));
#57491=CARTESIAN_POINT('Ctrl Pts',(96.446025,8.99786583245493,-7.4912658540953));
#57492=CARTESIAN_POINT('Ctrl Pts',(96.446025,8.80804585445648,-7.69558542180113));
#57493=CARTESIAN_POINT('Ctrl Pts',(96.446025,8.61118064520521,-7.89294354453129));
#57494=CARTESIAN_POINT('Ctrl Pts',(96.446025,8.41581792234265,-8.08879541892925));
#57495=CARTESIAN_POINT('Ctrl Pts',(96.446025,8.213516645606,-8.27779209165663));
#57496=CARTESIAN_POINT('Ctrl Pts',(96.446025,8.0045663838185,-8.45947766735397));
#57497=CARTESIAN_POINT('Ctrl Pts',(96.446025,7.79927809976704,-8.63797909517099));
#57498=CARTESIAN_POINT('Ctrl Pts',(96.446025,7.58757139889719,-8.80942372620072));
#57499=CARTESIAN_POINT('Ctrl Pts',(96.446025,7.36969868465615,-8.97333427215897));
#57500=CARTESIAN_POINT('Ctrl Pts',(96.446025,7.28186302611182,-9.03941501474648));
#57501=CARTESIAN_POINT('Ctrl Pts',(96.446025,7.19302498107236,-9.1042706958156));
#57502=CARTESIAN_POINT('Ctrl Pts',(96.446025,7.10320028565113,-9.16786776036423));
#57503=CARTESIAN_POINT('Ctrl Pts',(97.4445933434715,-1.68965488935083,-12.5000313373793));
#57504=CARTESIAN_POINT('Ctrl Pts',(97.4342177497292,-2.13885530702409,-12.4397673843726));
#57505=CARTESIAN_POINT('Ctrl Pts',(97.4238421559868,-2.58473989646664,-12.3553149612025));
#57506=CARTESIAN_POINT('Ctrl Pts',(97.4134665622445,-3.02464884153746,-12.2466674174002));
#57507=CARTESIAN_POINT('Ctrl Pts',(97.3663747611614,-5.02126754600492,-11.7535478284925));
#57508=CARTESIAN_POINT('Ctrl Pts',(97.3192829600784,-6.89478869514797,-10.7620116646819));
#57509=CARTESIAN_POINT('Ctrl Pts',(97.2721911589953,-8.42541152523419,-9.388386362015));
#57510=CARTESIAN_POINT('Ctrl Pts',(97.2250993579122,-9.95603435532041,-8.01476105934808));
#57511=CARTESIAN_POINT('Ctrl Pts',(97.1780075568291,-11.1437588663498,-6.25904661782482));
#57512=CARTESIAN_POINT('Ctrl Pts',(97.1309157557461,-11.8492413813291,-4.32722131968821));
#57513=CARTESIAN_POINT('Ctrl Pts',(97.083823954663,-12.5547238963084,-2.3953960215516));
#57514=CARTESIAN_POINT('Ctrl Pts',(97.0367321535799,-12.7779644152377,-0.287459866801626));
#57515=CARTESIAN_POINT('Ctrl Pts',(96.9896403524969,-12.4927729217965,1.74928154978578));
#57516=CARTESIAN_POINT('Ctrl Pts',(96.9425485514138,-12.2075814283553,3.78602296637319));
#57517=CARTESIAN_POINT('Ctrl Pts',(96.8954567503308,-11.4139579225437,5.75156964479803));
#57518=CARTESIAN_POINT('Ctrl Pts',(96.8483649492477,-10.2050090351847,7.4153310294173));
#57519=CARTESIAN_POINT('Ctrl Pts',(96.8012731481646,-8.99606014782565,9.07909241403658));
#57520=CARTESIAN_POINT('Ctrl Pts',(96.7541813470815,-7.37178587891919,10.4410685048503));
#57521=CARTESIAN_POINT('Ctrl Pts',(96.7070895459985,-5.52274765596046,11.3414587153849));
#57522=CARTESIAN_POINT('Ctrl Pts',(96.6599977449154,-3.67370943300174,12.2418489259194));
#57523=CARTESIAN_POINT('Ctrl Pts',(96.6129059438324,-1.59990725599075,12.6806532561748));
#57524=CARTESIAN_POINT('Ctrl Pts',(96.5658141427493,0.455365491869809,12.606420506603));
#57525=CARTESIAN_POINT('Ctrl Pts',(96.5258844284996,2.19805639856598,12.5434776500929));
#57526=CARTESIAN_POINT('Ctrl Pts',(96.4859547142498,3.92742547663266,12.1116841397094));
#57527=CARTESIAN_POINT('Ctrl Pts',(96.446025,5.49780057593998,11.3530041107288));
#57528=CARTESIAN_POINT('Ctrl Pts',(107.482029246699,-0.87623857414724,12.583168122964));
#57529=CARTESIAN_POINT('Ctrl Pts',(107.513300150711,-2.23895227724843,12.4882745078976));
#57530=CARTESIAN_POINT('Ctrl Pts',(107.607112862745,-6.28931688652167,11.5416513005363));
#57531=CARTESIAN_POINT('Ctrl Pts',(107.73219647879,-10.6085644348937,7.75715356972124));
#57532=CARTESIAN_POINT('Ctrl Pts',(107.888550998846,-13.0749717130243,1.27479764955593));
#57533=CARTESIAN_POINT('Ctrl Pts',(108.013634614891,-12.3768301122727,-4.42234600477363));
#57534=CARTESIAN_POINT('Ctrl Pts',(108.169989134948,-8.39216919057065,-10.1004171650069));
#57535=CARTESIAN_POINT('Ctrl Pts',(108.263801846982,-4.56292341074069,-12.0725978039739));
#57536=CARTESIAN_POINT('Ctrl Pts',(108.326343655004,-1.86078767833722,-12.47563157783));
#57537=CARTESIAN_POINT('Ctrl Pts',(107.677558537865,-0.852712233050537,
12.2453196030831));
#57538=CARTESIAN_POINT('Ctrl Pts',(107.708829441876,-2.17883810682964,12.1529738096052));
#57539=CARTESIAN_POINT('Ctrl Pts',(107.80264215391,-6.12045349850929,11.2317667173564));
#57540=CARTESIAN_POINT('Ctrl Pts',(107.927725769955,-10.3237325263182,7.54887988010594));
#57541=CARTESIAN_POINT('Ctrl Pts',(108.084080290012,-12.7239186397789,1.24057029958798));
#57542=CARTESIAN_POINT('Ctrl Pts',(108.209163906057,-12.0445216114733,-4.30360936885544));
#57543=CARTESIAN_POINT('Ctrl Pts',(108.365518426114,-8.16684581318923,-9.82922862520268));
#57544=CARTESIAN_POINT('Ctrl Pts',(108.459331138147,-4.44041237809897,-11.7484577098948));
#57545=CARTESIAN_POINT('Ctrl Pts',(108.52187294617,-1.81082694056469,-12.1406703326204));
#57546=CARTESIAN_POINT('Ctrl Pts',(107.873087829031,-0.829185891953833,
11.9074710832022));
#57547=CARTESIAN_POINT('Ctrl Pts',(107.904358733042,-2.11872393641085,11.8176731113129));
#57548=CARTESIAN_POINT('Ctrl Pts',(107.998171445076,-5.95159011049691,10.9218821341765));
#57549=CARTESIAN_POINT('Ctrl Pts',(108.123255061121,-10.0389006177427,7.34060619049065));
#57550=CARTESIAN_POINT('Ctrl Pts',(108.279609581177,-12.3728655665335,1.20634294962002));
#57551=CARTESIAN_POINT('Ctrl Pts',(108.404693197223,-11.7122131106739,-4.18487273293724));
#57552=CARTESIAN_POINT('Ctrl Pts',(108.561047717279,-7.9415224358078,-9.55804008539851));
#57553=CARTESIAN_POINT('Ctrl Pts',(108.654860429313,-4.31790134545723,-11.4243176158158));
#57554=CARTESIAN_POINT('Ctrl Pts',(108.717402237336,-1.76086620279216,-11.8057090874109));
#57555=CARTESIAN_POINT('Ctrl Pts',(108.068617120196,-0.80565955085713,11.5696225633213));
#57556=CARTESIAN_POINT('Ctrl Pts',(108.099888024207,-2.05860976599205,11.4823724130206));
#57557=CARTESIAN_POINT('Ctrl Pts',(108.193700736241,-5.78272672248452,10.6119975509966));
#57558=CARTESIAN_POINT('Ctrl Pts',(108.318784352286,-9.75406870916728,7.13233250087535));
#57559=CARTESIAN_POINT('Ctrl Pts',(108.475138872343,-12.0218124932882,1.17211559965207));
#57560=CARTESIAN_POINT('Ctrl Pts',(108.600222488388,-11.3799046098746,-4.06613609701905));
#57561=CARTESIAN_POINT('Ctrl Pts',(108.756577008445,-7.71619905842638,-9.28685154559433));
#57562=CARTESIAN_POINT('Ctrl Pts',(108.850389720479,-4.1953903128155,-11.1001775217368));
#57563=CARTESIAN_POINT('Ctrl Pts',(108.912931528501,-1.71090546501964,-11.4707478422013));
#57564=CARTESIAN_POINT('',(108.902670614213,-2.11726001551285,-11.4025478033388));
#57565=CARTESIAN_POINT('',(108.326343655004,-1.8607876783373,-12.47563157783));
#57566=CARTESIAN_POINT('Ctrl Pts',(108.902670614213,-2.11721675886238,-11.4024697825115));
#57567=CARTESIAN_POINT('Ctrl Pts',(108.834581877771,-2.09803382047897,-11.5278634706509));
#57568=CARTESIAN_POINT('Ctrl Pts',(108.766763876508,-2.07538442706099,-11.6532854109009));
#57569=CARTESIAN_POINT('Ctrl Pts',(108.699537896827,-2.04914360253286,-11.7780872230819));
#57570=CARTESIAN_POINT('Ctrl Pts',(108.670954314328,-2.03798635683282,-11.8311512752736));
#57571=CARTESIAN_POINT('Ctrl Pts',(108.642477759625,-2.02618043104393,-11.8841030055665));
#57572=CARTESIAN_POINT('Ctrl Pts',(108.614132928961,-2.01371895975861,-11.936891665109));
#57573=CARTESIAN_POINT('Ctrl Pts',(108.550622506313,-1.98579734972971,-12.0551717888559));
#57574=CARTESIAN_POINT('Ctrl Pts',(108.487405157811,-1.95442030405157,-12.1733202167919));
#57575=CARTESIAN_POINT('Ctrl Pts',(108.424880007573,-1.9194031665709,-12.290556812487));
#57576=CARTESIAN_POINT('Ctrl Pts',(108.391821388282,-1.90088872538617,-12.3525427488559));
#57577=CARTESIAN_POINT('Ctrl Pts',(108.35895627321,-1.88135746538499,-12.4142734666444));
#57578=CARTESIAN_POINT('Ctrl Pts',(108.326343655004,-1.8607876783373,-12.47563157783));
#57579=CARTESIAN_POINT('',(108.090753740172,-1.68967307116025,11.4740625043632));
#57580=CARTESIAN_POINT('Ctrl Pts',(108.090753740172,-1.68975055635687,11.4740963971941));
#57581=CARTESIAN_POINT('Ctrl Pts',(108.114645770858,-2.63984049686771,11.3346921771064));
#57582=CARTESIAN_POINT('Ctrl Pts',(108.201079609567,-6.01700224455775,10.4067268014638));
#57583=CARTESIAN_POINT('Ctrl Pts',(108.318784352286,-9.75406870916728,7.13233250087535));
#57584=CARTESIAN_POINT('Ctrl Pts',(108.475138872343,-12.0218124932882,1.17211559965207));
#57585=CARTESIAN_POINT('Ctrl Pts',(108.600222488388,-11.3799046098746,-4.06613609701905));
#57586=CARTESIAN_POINT('Ctrl Pts',(108.753156703682,-7.79634378044959,-9.17264673778085));
#57587=CARTESIAN_POINT('Ctrl Pts',(108.843549110953,-4.45036163137592,-10.9662005008345));
#57588=CARTESIAN_POINT('Ctrl Pts',(108.902670614213,-2.1172167588623,-11.4024697825115));
#57589=CARTESIAN_POINT('',(107.482029246699,-0.87623857414724,12.583168122964));
#57590=CARTESIAN_POINT('Ctrl Pts',(107.482029246699,-0.87623857414724,12.583168122964));
#57591=CARTESIAN_POINT('Ctrl Pts',(107.482394382578,-0.877079479290065,
12.5825107576108));
#57592=CARTESIAN_POINT('Ctrl Pts',(107.482759857299,-0.877919727242279,
12.5818527375208));
#57593=CARTESIAN_POINT('Ctrl Pts',(107.483125668906,-0.87875931790496,12.5811940664401));
#57594=CARTESIAN_POINT('Ctrl Pts',(107.50706618734,-0.933706277910721,12.5380873775059));
#57595=CARTESIAN_POINT('Ctrl Pts',(107.532594415577,-0.986211055902737,
12.491930905356));
#57596=CARTESIAN_POINT('Ctrl Pts',(107.559298891057,-1.03624927992292,12.4435191439929));
#57597=CARTESIAN_POINT('Ctrl Pts',(107.586988876219,-1.08813412902446,12.3933207809964));
#57598=CARTESIAN_POINT('Ctrl Pts',(107.615943527723,-1.13736712243412,12.3406977585454));
#57599=CARTESIAN_POINT('Ctrl Pts',(107.645704126984,-1.18397787806622,12.2865272927665));
#57600=CARTESIAN_POINT('Ctrl Pts',(107.671575494813,-1.22449735797087,12.2394360351848));
#57601=CARTESIAN_POINT('Ctrl Pts',(107.698055925798,-1.2630362708689,12.19117525119));
#57602=CARTESIAN_POINT('Ctrl Pts',(107.724844064182,-1.29964537358992,12.1423150531443));
#57603=CARTESIAN_POINT('Ctrl Pts',(107.762653981563,-1.35131701756271,12.0733516923896));
#57604=CARTESIAN_POINT('Ctrl Pts',(107.801780392181,-1.40010211706753,12.0019112292348));
#57605=CARTESIAN_POINT('Ctrl Pts',(107.841816435641,-1.44606245484022,11.9287853832026));
#57606=CARTESIAN_POINT('Ctrl Pts',(107.883429900903,-1.49383363186028,11.8527783757514));
#57607=CARTESIAN_POINT('Ctrl Pts',(107.926026090234,-1.53855319806583,11.7749507224119));
#57608=CARTESIAN_POINT('Ctrl Pts',(107.969148132621,-1.58034682115879,11.6961777693696));
#57609=CARTESIAN_POINT('Ctrl Pts',(108.009349694466,-1.61930993214651,11.6227397880442));
#57610=CARTESIAN_POINT('Ctrl Pts',(108.050008293574,-1.65573088360539,11.5484801021652));
#57611=CARTESIAN_POINT('Ctrl Pts',(108.090753740172,-1.68975055635671,11.4740963971942));
#57612=CARTESIAN_POINT('Ctrl Pts',(108.326343655004,-1.86078767833722,-12.47563157783));
#57613=CARTESIAN_POINT('Ctrl Pts',(108.263801846982,-4.56292341074069,-12.0725978039739));
#57614=CARTESIAN_POINT('Ctrl Pts',(108.201260038959,-7.11575393062732,-10.7578107113292));
#57615=CARTESIAN_POINT('Ctrl Pts',(108.138718230937,-9.02927368304341,-8.80539603771879));
#57616=CARTESIAN_POINT('Ctrl Pts',(108.107447326925,-9.98603355925145,-7.82918870091359));
#57617=CARTESIAN_POINT('Ctrl Pts',(108.076176422914,-10.7829657435919,-6.69357446886696));
#57618=CARTESIAN_POINT('Ctrl Pts',(108.044905518903,-11.3724323332148,-5.46173634297509));
#57619=CARTESIAN_POINT('Ctrl Pts',(107.98236371088,-12.5513655124606,-2.99806009119129));
#57620=CARTESIAN_POINT('Ctrl Pts',(107.919821902858,-12.9004363128364,-0.149488264026472));
#57621=CARTESIAN_POINT('Ctrl Pts',(107.857280094835,-12.3590846387935,2.52866392373924));
#57622=CARTESIAN_POINT('Ctrl Pts',(107.826009190824,-12.088408801772,3.86774001762206));
#57623=CARTESIAN_POINT('Ctrl Pts',(107.794738286812,-11.5951273461459,5.16421120165511));
#57624=CARTESIAN_POINT('Ctrl Pts',(107.763467382801,-10.9063357466975,6.34390013524507));
#57625=CARTESIAN_POINT('Ctrl Pts',(107.700925574779,-9.52875254780069,8.703278002425));
#57626=CARTESIAN_POINT('Ctrl Pts',(107.638383766756,-7.36912877361468,10.5955268678326));
#57627=CARTESIAN_POINT('Ctrl Pts',(107.575841958733,-4.84909213365347,11.646997915129));
#57628=CARTESIAN_POINT('Ctrl Pts',(107.544571054722,-3.58907381367288,12.1727334387771));
#57629=CARTESIAN_POINT('Ctrl Pts',(107.513300150711,-2.23895227724849,12.4882745078976));
#57630=CARTESIAN_POINT('Ctrl Pts',(107.482029246699,-0.876238574147329,
12.583168122964));
#57631=CARTESIAN_POINT('Origin',(93.0806848796603,0.,0.));
#57632=CARTESIAN_POINT('Ctrl Pts',(110.814071804302,1.76443058609261,-11.4626366197512));
#57633=CARTESIAN_POINT('Ctrl Pts',(110.901035745034,1.69966359360912,-11.472606129062));
#57634=CARTESIAN_POINT('Ctrl Pts',(110.98193435915,1.62933547807125,-11.4828589976618));
#57635=CARTESIAN_POINT('Ctrl Pts',(111.100478831822,1.5107910053991,-11.4989048142971));
#57636=CARTESIAN_POINT('Ctrl Pts',(111.144081499747,1.46329723353908,-11.5050660129585));
#57637=CARTESIAN_POINT('Ctrl Pts',(111.185928218469,1.41338106757117,-11.5111948783535));
#57638=CARTESIAN_POINT('Ctrl Pts',(111.683757644765,-0.266838057499402,
11.5945698937334));
#57639=CARTESIAN_POINT('Ctrl Pts',(111.694737994272,-0.176976729613362,
11.5966379671848));
#57640=CARTESIAN_POINT('Ctrl Pts',(111.7,-0.0875694530144953,11.59764));
#57641=CARTESIAN_POINT('Ctrl Pts',(111.7,0.122714157654495,11.59764));
#57642=CARTESIAN_POINT('Ctrl Pts',(111.689602674459,0.249054699568216,11.5956523517617));
#57643=CARTESIAN_POINT('Ctrl Pts',(111.667770384747,0.375195361129816,11.5915694369049));
#57644=CARTESIAN_POINT('Origin',(93.0806848796603,0.,0.));
#57645=CARTESIAN_POINT('Origin',(96.446025,0.,0.));
#57646=CARTESIAN_POINT('Origin',(93.0806848796603,0.,0.));
#57647=CARTESIAN_POINT('Ctrl Pts',(109.916925613585,-2.16013264239418,11.3946952805621));
#57648=CARTESIAN_POINT('Ctrl Pts',(110.044752529268,-2.13546086335257,11.3993723968817));
#57649=CARTESIAN_POINT('Ctrl Pts',(110.171957681553,-2.09901013524074,11.4062154433825));
#57650=CARTESIAN_POINT('Ctrl Pts',(110.294852708433,-2.05139200834394,11.4147730769255));
#57651=CARTESIAN_POINT('Ctrl Pts',(111.113306560609,-1.49574126823374,-11.5007830876033));
#57652=CARTESIAN_POINT('Ctrl Pts',(111.094345708019,-1.51619244420004,-11.4981232976009));
#57653=CARTESIAN_POINT('Ctrl Pts',(111.075107334507,-1.5361625027139,-11.4954706061514));
#57654=CARTESIAN_POINT('Ctrl Pts',(110.957135649226,-1.6541341879949,-11.4795023202626));
#57655=CARTESIAN_POINT('Ctrl Pts',(110.845701752448,-1.74655296335327,-11.465670048636));
#57656=CARTESIAN_POINT('Ctrl Pts',(110.724270236999,-1.82788467546432,-11.4526892554894));
#57657=CARTESIAN_POINT('Origin',(93.0806848796603,0.,0.));
#57658=CARTESIAN_POINT('Ctrl Pts',(109.281532350295,-2.18912582690723,-11.3891607102353));
#57659=CARTESIAN_POINT('Ctrl Pts',(109.155412564872,-2.17653948181738,-11.3915799484745));
#57660=CARTESIAN_POINT('Ctrl Pts',(109.027830981515,-2.15266538708709,-11.3961649260526));
#57661=CARTESIAN_POINT('Ctrl Pts',(108.902670614213,-2.1173562772654,-11.4027214280068));
#57662=CARTESIAN_POINT('Ctrl Pts',(108.090753740172,-1.68938597696385,11.4739369263753));
#57663=CARTESIAN_POINT('Ctrl Pts',(108.20790113293,-1.78710759140999,11.4595487066952));
#57664=CARTESIAN_POINT('Ctrl Pts',(108.33848779035,-1.87501865749023,11.44530766719));
#57665=CARTESIAN_POINT('Ctrl Pts',(108.477958351107,-1.94818655881029,11.4328396604549));
#57666=CARTESIAN_POINT('Origin',(93.0806848796603,0.,0.));
#57667=CARTESIAN_POINT('',(109.009389146813,2.14465603270175,-11.397646135533));
#57668=CARTESIAN_POINT('Ctrl Pts',(109.009389146813,2.14459809538638,-11.3976292525624));
#57669=CARTESIAN_POINT('Ctrl Pts',(109.136652663705,2.17371164479049,-11.3921511955719));
#57670=CARTESIAN_POINT('Ctrl Pts',(109.265320582609,2.19108690692555,-11.3887853615113));
#57671=CARTESIAN_POINT('Ctrl Pts',(109.391405608182,2.19731819681761,-11.3875829881294));
#57672=CARTESIAN_POINT('',(109.808269534075,2.1782830168169,11.391215608372));
#57673=CARTESIAN_POINT('Ctrl Pts',(109.009389146813,2.14467064967058,-11.3976503949269));
#57674=CARTESIAN_POINT('Ctrl Pts',(109.036249487207,3.2052865345203,-11.1982841745728));
#57675=CARTESIAN_POINT('Ctrl Pts',(109.12332934527,6.55809015436484,-10.0745075843251));
#57676=CARTESIAN_POINT('Ctrl Pts',(109.240518962169,10.069373101794,-6.61415923889863));
#57677=CARTESIAN_POINT('Ctrl Pts',(109.391067756344,12.0167660168964,-0.799058821012281));
#57678=CARTESIAN_POINT('Ctrl Pts',(109.511506791684,11.2878420523094,4.21258051924178));
#57679=CARTESIAN_POINT('Ctrl Pts',(109.660610637206,7.77769110684894,9.17022383928472));
#57680=CARTESIAN_POINT('Ctrl Pts',(109.749494965058,4.49625225668538,10.9466376677334));
#57681=CARTESIAN_POINT('Ctrl Pts',(109.808269534075,2.17827022429556,11.3911929596074));
#57682=CARTESIAN_POINT('Ctrl Pts',(110.191221970063,2.0885909575843,11.4080253059632));
#57683=CARTESIAN_POINT('Ctrl Pts',(110.065692123374,2.13013522819152,11.4004193456324));
#57684=CARTESIAN_POINT('Ctrl Pts',(109.936720884488,2.16011691071928,11.3947132932223));
#57685=CARTESIAN_POINT('Ctrl Pts',(109.808269534075,2.1782951807231,11.3912371441928));
#57686=CARTESIAN_POINT('Origin',(117.38636,1.35008033100152E-15,0.));
#57687=CARTESIAN_POINT('',(117.38636,-12.6136400000002,-1.54472538515972E-15));
#57688=CARTESIAN_POINT('Origin',(117.38636,0.,0.));
#57689=CARTESIAN_POINT('Origin',(117.38636,0.,0.));
#57690=CARTESIAN_POINT('Origin',(96.446025,-1.35008033100152E-15,0.));
#57691=CARTESIAN_POINT('',(96.446025,1.68935314532052,-12.4999999999999));
#57692=CARTESIAN_POINT('',(96.4460250000001,-1.68935314532052,-12.4999999999999));
#57693=CARTESIAN_POINT('',(96.446025,-1.35,-12.5));
#57694=CARTESIAN_POINT('Origin',(96.446025,0.,0.));
#57695=CARTESIAN_POINT('',(96.4460250000001,-12.6136400000002,-1.54472538515972E-15));
#57696=CARTESIAN_POINT('Origin',(96.446025,0.,0.));
#57697=CARTESIAN_POINT('Origin',(96.446025,0.,0.));
#57698=CARTESIAN_POINT('Ctrl Pts',(108.413053017993,1.91273266775695,-12.4677731689061));
#57699=CARTESIAN_POINT('Ctrl Pts',(108.443162776828,3.21281350456061,-12.2683223885951));
#57700=CARTESIAN_POINT('Ctrl Pts',(108.533492053333,7.02671572005891,-11.0614285744525));
#57701=CARTESIAN_POINT('Ctrl Pts',(108.653931088672,10.9514907629236,-7.19358624186833));
#57702=CARTESIAN_POINT('Ctrl Pts',(108.804479882847,13.0694831449644,-0.86905959376855));
#57703=CARTESIAN_POINT('Ctrl Pts',(108.924918918187,12.2767025036725,4.58161954852267));
#57704=CARTESIAN_POINT('Ctrl Pts',(109.075467712362,8.42205173022918,10.0258252123201));
#57705=CARTESIAN_POINT('Ctrl Pts',(109.165796988867,4.77376444645626,11.9680846522454));
#57706=CARTESIAN_POINT('Ctrl Pts',(109.226016506537,2.18287265897621,12.4233240722559));
#57707=CARTESIAN_POINT('Ctrl Pts',(108.608582309158,1.86137724641834,-12.1330229160156));
#57708=CARTESIAN_POINT('Ctrl Pts',(108.638692067993,3.12655189885353,-11.9389272378743));
#57709=CARTESIAN_POINT('Ctrl Pts',(108.729021344498,6.83805373267649,-10.7644376072233));
#57710=CARTESIAN_POINT('Ctrl Pts',(108.849460379838,10.6574515425471,-7.0004439075451));
#57711=CARTESIAN_POINT('Ctrl Pts',(109.000009174013,12.7185774356084,-0.845726002849796));
#57712=CARTESIAN_POINT('Ctrl Pts',(109.120448209353,11.9470823532181,4.45860653876238));
#57713=CARTESIAN_POINT('Ctrl Pts',(109.270997003527,8.19592602932356,9.75663940986822));
#57714=CARTESIAN_POINT('Ctrl Pts',(109.361326280032,4.64559249192662,11.646750657018));
#57715=CARTESIAN_POINT('Ctrl Pts',(109.421545797702,2.12426418377211,12.0897672438963));
#57716=CARTESIAN_POINT('Ctrl Pts',(108.804111600324,1.81002182507974,-11.7982726631251));
#57717=CARTESIAN_POINT('Ctrl Pts',(108.834221359159,3.04029029314645,-11.6095320871536));
#57718=CARTESIAN_POINT('Ctrl Pts',(108.924550635664,6.64939174529407,-10.467446639994));
#57719=CARTESIAN_POINT('Ctrl Pts',(109.044989671003,10.3634123221706,-6.80730157322186));
#57720=CARTESIAN_POINT('Ctrl Pts',(109.195538465178,12.3676717262524,-0.822392411931035));
#57721=CARTESIAN_POINT('Ctrl Pts',(109.315977500518,11.6174622027638,4.33559352900208));
#57722=CARTESIAN_POINT('Ctrl Pts',(109.466526294693,7.96980032841795,9.48745360741635));
#57723=CARTESIAN_POINT('Ctrl Pts',(109.556855571198,4.51742053739697,11.3254166617906));
#57724=CARTESIAN_POINT('Ctrl Pts',(109.617075088868,2.06565570856801,11.7562104155366));
#57725=CARTESIAN_POINT('Ctrl Pts',(108.999640891489,1.75866640374113,-11.4635224102347));
#57726=CARTESIAN_POINT('Ctrl Pts',(109.029750650324,2.95402868743937,-11.2801369364328));
#57727=CARTESIAN_POINT('Ctrl Pts',(109.120079926829,6.46072975791164,-10.1704556727648));
#57728=CARTESIAN_POINT('Ctrl Pts',(109.240518962169,10.069373101794,-6.61415923889863));
#57729=CARTESIAN_POINT('Ctrl Pts',(109.391067756344,12.0167660168964,-0.799058821012281));
#57730=CARTESIAN_POINT('Ctrl Pts',(109.511506791684,11.2878420523094,4.21258051924178));
#57731=CARTESIAN_POINT('Ctrl Pts',(109.662055585858,7.74367462751234,9.21826780496448));
#57732=CARTESIAN_POINT('Ctrl Pts',(109.752384862363,4.38924858286732,11.0040826665632));
#57733=CARTESIAN_POINT('Ctrl Pts',(109.812604380033,2.00704723336391,11.4226535871769));
#57734=CARTESIAN_POINT('',(108.413053017993,1.91273266775704,-12.4677731689061));
#57735=CARTESIAN_POINT('Ctrl Pts',(108.413053017993,1.91273266775695,-12.4677731689061));
#57736=CARTESIAN_POINT('Ctrl Pts',(108.413855852925,1.9131888940879,-12.4663232667956));
#57737=CARTESIAN_POINT('Ctrl Pts',(108.414658783089,1.91364450647225,-12.4648732233092));
#57738=CARTESIAN_POINT('Ctrl Pts',(108.415461807794,1.91409950547309,-12.4634230398033));
#57739=CARTESIAN_POINT('Ctrl Pts',(108.479752286689,1.9505269073821,-12.3473207685653));
#57740=CARTESIAN_POINT('Ctrl Pts',(108.544861582718,1.98314984730452,-12.229936946399));
#57741=CARTESIAN_POINT('Ctrl Pts',(108.610394801366,2.01212814785511,-12.1120411801108));
#57742=CARTESIAN_POINT('Ctrl Pts',(108.644839096371,2.02735915822723,-12.0500751018714));
#57743=CARTESIAN_POINT('Ctrl Pts',(108.679400502512,2.04158417778305,-11.9879672915395));
#57744=CARTESIAN_POINT('Ctrl Pts',(108.714021681,2.05483173131018,-11.9258274377091));
#57745=CARTESIAN_POINT('Ctrl Pts',(108.782570306368,2.08106138678214,-11.8027928748588));
#57746=CARTESIAN_POINT('Ctrl Pts',(108.85175216169,2.10360807176127,-11.6789176806214));
#57747=CARTESIAN_POINT('Ctrl Pts',(108.921251264686,2.12256886627832,-11.5548280565426));
#57748=CARTESIAN_POINT('Ctrl Pts',(108.950581971157,2.13057089039742,-11.5024585124332));
#57749=CARTESIAN_POINT('Ctrl Pts',(108.979969182396,2.1379348534859,-11.4500505742848));
#57750=CARTESIAN_POINT('Ctrl Pts',(109.009389146813,2.1446706496705,-11.397650394927));
#57751=CARTESIAN_POINT('',(109.226016506537,2.1828726589771,12.4233240722558));
#57752=CARTESIAN_POINT('Ctrl Pts',(109.226016506537,2.18287265897622,12.4233240722559));
#57753=CARTESIAN_POINT('Ctrl Pts',(109.165796988867,4.77376444645624,11.9680846522455));
#57754=CARTESIAN_POINT('Ctrl Pts',(109.105577471197,7.20595596897156,10.6732450256285));
#57755=CARTESIAN_POINT('Ctrl Pts',(109.045357953527,9.04459334939484,8.7898436397436));
#57756=CARTESIAN_POINT('Ctrl Pts',(109.015248194692,9.96391203960649,7.84814294680113));
#57757=CARTESIAN_POINT('Ctrl Pts',(108.985138435857,10.7348421942951,6.75930181404173));
#57758=CARTESIAN_POINT('Ctrl Pts',(108.955028677022,11.3148606841952,5.57918446367781));
#57759=CARTESIAN_POINT('Ctrl Pts',(108.894809159352,12.4748976639954,3.21894976294992));
#57760=CARTESIAN_POINT('Ctrl Pts',(108.834589641682,12.8712879846414,0.493610191804197));
#57761=CARTESIAN_POINT('Ctrl Pts',(108.774370124012,12.4386201229791,-2.10137677140434));
#57762=CARTESIAN_POINT('Ctrl Pts',(108.744260365177,12.222286192148,-3.39887025300854));
#57763=CARTESIAN_POINT('Ctrl Pts',(108.714150606342,11.7986877157399,-4.66377558262845));
#57764=CARTESIAN_POINT('Ctrl Pts',(108.684040847507,11.1892241445624,-5.82936599675708));
#57765=CARTESIAN_POINT('Ctrl Pts',(108.623821329837,9.9702970022074,-8.16054682501441));
#57766=CARTESIAN_POINT('Ctrl Pts',(108.563601812167,8.00790948077504,-10.0944679913065));
#57767=CARTESIAN_POINT('Ctrl Pts',(108.503382294498,5.65871265563164,-11.2755056308006));
#57768=CARTESIAN_POINT('Ctrl Pts',(108.473272535663,4.48411424306014,-11.8660244505475));
#57769=CARTESIAN_POINT('Ctrl Pts',(108.443162776828,3.21281350456093,-12.268322388595));
#57770=CARTESIAN_POINT('Ctrl Pts',(108.413053017993,1.91273266775748,-12.467773168906));
#57771=CARTESIAN_POINT('Ctrl Pts',(109.808269534075,2.17827022429548,11.3911929596074));
#57772=CARTESIAN_POINT('Ctrl Pts',(109.743176121344,2.18748537356643,11.5047642900023));
#57773=CARTESIAN_POINT('Ctrl Pts',(109.678142238689,2.19372201690515,11.6188991359825));
#57774=CARTESIAN_POINT('Ctrl Pts',(109.613368850412,2.19706582260749,11.7331774438013));
#57775=CARTESIAN_POINT('Ctrl Pts',(109.581094983429,2.1987319009666,11.7901175391662));
#57776=CARTESIAN_POINT('Ctrl Pts',(109.548885787082,2.1996805463104,11.8470929825011));
#57777=CARTESIAN_POINT('Ctrl Pts',(109.516766120282,2.19992700252409,11.9040503705732));
#57778=CARTESIAN_POINT('Ctrl Pts',(109.447893339496,2.20045546768175,12.0261815784489));
#57779=CARTESIAN_POINT('Ctrl Pts',(109.379164341258,2.19775214763542,12.1487063361486));
#57780=CARTESIAN_POINT('Ctrl Pts',(109.310802500265,2.1918507117029,12.2711579454467));
#57781=CARTESIAN_POINT('Ctrl Pts',(109.28247214663,2.18940505247996,12.3219040538631));
#57782=CARTESIAN_POINT('Ctrl Pts',(109.254204849311,2.18641072181222,12.3726374129757));
#57783=CARTESIAN_POINT('Ctrl Pts',(109.226016506537,2.18287265897719,12.4233240722558));
#57784=CARTESIAN_POINT('Origin',(118.5,-2.7,-12.5));
#57785=CARTESIAN_POINT('',(108.090714382958,-1.68935314531923,-12.5));
#57786=CARTESIAN_POINT('Origin',(109.5,0.,-12.5));
#57787=CARTESIAN_POINT('',(106.9,-1.68935314531923,-12.5));
#57788=CARTESIAN_POINT('Origin',(118.5,-2.7,-12.5));
#57789=CARTESIAN_POINT('',(106.9,-1.68935314531923,-12.5));
#57790=CARTESIAN_POINT('',(106.9,1.68935314531923,-12.5));
#57791=CARTESIAN_POINT('Origin',(118.5,-2.7,-12.5));
#57792=CARTESIAN_POINT('',(106.9,1.68935314531923,-12.5));
#57793=CARTESIAN_POINT('',(106.9,-1.68935314531923,-12.5));
#57794=CARTESIAN_POINT('Origin',(118.5,-2.7,-12.5));
#57795=CARTESIAN_POINT('',(106.9,1.68935314531923,-12.5));
#57796=CARTESIAN_POINT('',(106.9,-1.68935314531923,-12.5));
#57797=CARTESIAN_POINT('Origin',(118.5,-2.7,-12.5));
#57798=CARTESIAN_POINT('',(106.9,1.68935314531923,-12.5));
#57799=CARTESIAN_POINT('',(106.9,-1.68935314531923,-12.5));
#57800=CARTESIAN_POINT('Origin',(118.5,-2.7,-12.5));
#57801=CARTESIAN_POINT('',(106.9,1.68935314531923,-12.5));
#57802=CARTESIAN_POINT('',(106.9,-1.68935314531923,-12.5));
#57803=CARTESIAN_POINT('Origin',(118.5,-2.7,-12.5));
#57804=CARTESIAN_POINT('',(106.9,1.68935314531923,-12.5));
#57805=CARTESIAN_POINT('',(106.9,-1.68935314531923,-12.5));
#57806=CARTESIAN_POINT('Origin',(118.5,-2.7,-12.5));
#57807=CARTESIAN_POINT('',(106.9,-1.68935314531923,-12.5));
#57808=CARTESIAN_POINT('',(106.9,1.68935314531923,-12.5));
#57809=CARTESIAN_POINT('Origin',(118.5,-2.7,-12.5));
#57810=CARTESIAN_POINT('',(106.9,-1.68935314531923,-12.5));
#57811=CARTESIAN_POINT('',(106.9,1.68935314531923,-12.5));
#57812=CARTESIAN_POINT('Origin',(118.5,-2.7,-12.5));
#57813=CARTESIAN_POINT('',(117.38636,1.68935314532054,-12.4999999999999));
#57814=CARTESIAN_POINT('',(106.9,1.68935314531923,-12.5));
#57815=CARTESIAN_POINT('',(117.38636,-1.68935314532053,-12.4999999999999));
#57816=CARTESIAN_POINT('Ctrl Pts',(117.38636,-1.68935314532052,-12.5));
#57817=CARTESIAN_POINT('Ctrl Pts',(117.61261618375,-5.55111512312578E-16,
-12.5));
#57818=CARTESIAN_POINT('Ctrl Pts',(117.38636,1.68935314532052,-12.5));
#57819=CARTESIAN_POINT('',(106.9,-1.68935314531923,-12.5));
#57820=CARTESIAN_POINT('Origin',(118.5,-2.7,-12.5));
#57821=CARTESIAN_POINT('Origin',(109.5,0.,-12.5));
#57822=CARTESIAN_POINT('',(106.9,1.68935314531923,-12.5));
#57823=CARTESIAN_POINT('',(106.9,-1.68935314531923,-12.5));
#57824=CARTESIAN_POINT('Origin',(106.9,0.,0.));
#57825=CARTESIAN_POINT('Origin',(106.9,0.,0.));
#57826=CARTESIAN_POINT('Ctrl Pts',(110.869631627566,-1.72165885261004,12.4955914163688));
#57827=CARTESIAN_POINT('Ctrl Pts',(110.935695199159,-1.66910328566579,12.5028325908013));
#57828=CARTESIAN_POINT('Ctrl Pts',(110.997867695831,-1.61340214138951,12.5101653135727));
#57829=CARTESIAN_POINT('Ctrl Pts',(111.078972847973,-1.53229698924803,12.5202449280198));
#57830=CARTESIAN_POINT('Ctrl Pts',(111.101974334193,-1.50824419914058,12.5231678926488));
#57831=CARTESIAN_POINT('Ctrl Pts',(111.124564900463,-1.48350560638761,12.5260977628875));
#57832=CARTESIAN_POINT('Origin',(106.9,0.,0.));
#57833=CARTESIAN_POINT('Origin',(106.9,0.,0.));
#57834=CARTESIAN_POINT('Origin',(117.38636,0.,0.));
#57835=CARTESIAN_POINT('Origin',(106.9,0.,0.));
#57836=CARTESIAN_POINT('Origin',(117.38636,0.,0.));
#57837=CARTESIAN_POINT('Origin',(106.9,0.,0.));
#57838=CARTESIAN_POINT('Ctrl Pts',(111.05480378529,1.55646560811611,12.5172412639667));
#57839=CARTESIAN_POINT('Ctrl Pts',(110.974324957434,1.63685850952933,12.5072447492757));
#57840=CARTESIAN_POINT('Ctrl Pts',(110.885269102117,1.71321337314212,12.4969493815617));
#57841=CARTESIAN_POINT('Ctrl Pts',(110.7891485355,1.78272152996985,12.4870259868466));
#57842=CARTESIAN_POINT('Ctrl Pts',(110.231099956476,2.07496815725955,-12.4418013645918));
#57843=CARTESIAN_POINT('Ctrl Pts',(110.146193941075,2.10488417498088,-12.4368121526325));
#57844=CARTESIAN_POINT('Ctrl Pts',(110.059563366867,2.12952031953925,-12.4325956901));
#57845=CARTESIAN_POINT('Ctrl Pts',(109.972381969055,2.14868687232742,-12.4292823113118));
#57846=CARTESIAN_POINT('Origin',(106.9,0.,0.));
#57847=CARTESIAN_POINT('Origin',(106.9,0.,0.));
#57848=CARTESIAN_POINT('Origin',(106.9,0.,0.));
#57849=CARTESIAN_POINT('Origin',(106.9,0.,0.));
#57850=CARTESIAN_POINT('Origin',(106.9,0.,0.));
#57851=CARTESIAN_POINT('Origin',(106.9,0.,0.));
#57852=CARTESIAN_POINT('Origin',(96.446025,0.,0.));
#57853=CARTESIAN_POINT('Origin',(106.9,0.,0.));
#57854=CARTESIAN_POINT('',(107.3,2.69422295812418E-16,12.61364));
#57855=CARTESIAN_POINT('Ctrl Pts',(107.3,2.08166817117217E-16,12.61364));
#57856=CARTESIAN_POINT('Ctrl Pts',(107.3,-0.276841916654518,12.61364));
#57857=CARTESIAN_POINT('Ctrl Pts',(107.35544265574,-0.571753236528152,12.6036005699437));
#57858=CARTESIAN_POINT('Ctrl Pts',(107.472444208643,-0.853911663388667,
12.5847079999432));
#57859=CARTESIAN_POINT('Ctrl Pts',(107.477190873565,-0.865095837719748,
12.583944055971));
#57860=CARTESIAN_POINT('Ctrl Pts',(107.482029246699,-0.876238574147231,
12.583168122964));
#57861=CARTESIAN_POINT('Ctrl Pts',(107.444020192937,0.782909338907701,12.5893195613048));
#57862=CARTESIAN_POINT('Ctrl Pts',(107.347281269023,0.528865525353306,12.6051181335116));
#57863=CARTESIAN_POINT('Ctrl Pts',(107.3,0.256601073912259,12.61364));
#57864=CARTESIAN_POINT('Ctrl Pts',(107.3,1.17961196366423E-15,12.61364));
#57865=CARTESIAN_POINT('Ctrl Pts',(108.090714382958,-1.68935314531923,-12.5));
#57866=CARTESIAN_POINT('Ctrl Pts',(108.164345299838,-1.75077724271102,-12.4916986406298));
#57867=CARTESIAN_POINT('Ctrl Pts',(108.243231824376,-1.80836647601685,-12.4834503986049));
#57868=CARTESIAN_POINT('Ctrl Pts',(108.326343655004,-1.86078767833678,-12.47563157783));
#57869=CARTESIAN_POINT('Origin',(106.9,0.,0.));
#57870=CARTESIAN_POINT('Ctrl Pts',(109.873072103706,-2.1681368050555,-12.4259042666586));
#57871=CARTESIAN_POINT('Ctrl Pts',(109.960853831938,-2.15303217054067,-12.428539802336));
#57872=CARTESIAN_POINT('Ctrl Pts',(110.048551732082,-2.13242381263147,-12.4321108515432));
#57873=CARTESIAN_POINT('Ctrl Pts',(110.134936209547,-2.10638458259799,-12.4365211389598));
#57874=CARTESIAN_POINT('Ctrl Pts',(109.065424143322,-2.156651067,12.4279028892572));
#57875=CARTESIAN_POINT('Ctrl Pts',(109.152578695929,-2.17421314041195,12.4248552902616));
#57876=CARTESIAN_POINT('Ctrl Pts',(109.240090470105,-2.18632008331947,12.4227197843719));
#57877=CARTESIAN_POINT('Ctrl Pts',(109.326702434851,-2.19316391405513,12.4215114255748));
#57878=CARTESIAN_POINT('Origin',(109.5,0.,15.));
#57879=CARTESIAN_POINT('Ctrl Pts',(109.226016506445,2.1828726589656,12.4233240722578));
#57880=CARTESIAN_POINT('Ctrl Pts',(109.139566669173,2.17202189846165,12.4252306335207));
#57881=CARTESIAN_POINT('Ctrl Pts',(109.05272927934,2.15587790155921,12.4280561642703));
#57882=CARTESIAN_POINT('Ctrl Pts',(108.966713351646,2.13438641081873,12.4317460036357));
#57883=CARTESIAN_POINT('',(107.3,2.69422295812418E-16,15.));
#57884=CARTESIAN_POINT('Ctrl Pts',(108.413053017994,1.91273266775782,-12.467773168906));
#57885=CARTESIAN_POINT('Ctrl Pts',(108.319914928113,1.85980516387165,-12.4758929962669));
#57886=CARTESIAN_POINT('Ctrl Pts',(108.23126343941,1.80036107420324,-12.4846642863292));
#57887=CARTESIAN_POINT('Ctrl Pts',(108.14853343171,1.73595452555452,-12.4936134058489));
#57888=CARTESIAN_POINT('Origin',(-13.25,0.,0.));
#57889=CARTESIAN_POINT('',(-12.5,-21.8313,-2.67356316662256E-15));
#57890=CARTESIAN_POINT('Origin',(-12.5,0.,0.));
#57891=CARTESIAN_POINT('',(-13.25,-23.61565,-2.89208301822842E-15));
#57892=CARTESIAN_POINT('Origin',(1.7825,0.,0.));
#57893=CARTESIAN_POINT('',(16.065,-21.8313,-2.67356316662256E-15));
#57894=CARTESIAN_POINT('Origin',(16.065,0.,0.));
#57895=CARTESIAN_POINT('',(1.7825,-21.8313,-2.67356316662256E-15));
#57896=CARTESIAN_POINT('Origin',(16.065,17.97,0.));
#57897=CARTESIAN_POINT('',(16.065,-17.97,-2.20069029806779E-15));
#57898=CARTESIAN_POINT('Origin',(16.065,0.,0.));
#57899=CARTESIAN_POINT('Origin',(16.315,0.,0.));
#57900=CARTESIAN_POINT('',(16.565,-17.47,-2.13945795811043E-15));
#57901=CARTESIAN_POINT('Origin',(16.565,0.,0.));
#57902=CARTESIAN_POINT('',(16.315,-17.72,-2.17007412808911E-15));
#57903=CARTESIAN_POINT('Origin',(25.7825,0.,0.));
#57904=CARTESIAN_POINT('',(35.,-17.47,-2.13945795811043E-15));
#57905=CARTESIAN_POINT('Origin',(35.,0.,0.));
#57906=CARTESIAN_POINT('',(25.7825,-17.47,-2.13945795811043E-15));
#57907=CARTESIAN_POINT('Origin',(37.5,0.,0.));
#57908=CARTESIAN_POINT('',(40.,-13.97,-1.71083157840885E-15));
#57909=CARTESIAN_POINT('Origin',(40.,0.,0.));
#57910=CARTESIAN_POINT('',(37.5,-15.72,-1.92514476825964E-15));
#57911=CARTESIAN_POINT('Origin',(40.25,0.,0.));
#57912=CARTESIAN_POINT('',(40.5,-13.47,-1.64959923845148E-15));
#57913=CARTESIAN_POINT('Origin',(40.5,0.,0.));
#57914=CARTESIAN_POINT('',(40.25,-13.72,-1.68021540843017E-15));
#57915=CARTESIAN_POINT('Origin',(86.,0.,-14.25));
#57916=CARTESIAN_POINT('',(86.,2.7,-13.1966245684266));
#57917=CARTESIAN_POINT('',(86.,-2.7,-13.1966245684266));
#57918=CARTESIAN_POINT('Origin',(86.,0.,0.));
#57919=CARTESIAN_POINT('',(86.,2.7,-12.5));
#57920=CARTESIAN_POINT('',(86.,-2.7,-16.));
#57921=CARTESIAN_POINT('Origin',(118.5,-2.7,-16.));
#57922=CARTESIAN_POINT('',(95.,-2.7,-13.1966245684266));
#57923=CARTESIAN_POINT('',(95.,-2.7,-8.));
#57924=CARTESIAN_POINT('',(67.75,-2.7,-13.1966245684266));
#57925=CARTESIAN_POINT('Origin',(67.75,0.,0.));
#57926=CARTESIAN_POINT('',(95.,2.7,-13.1966245684266));
#57927=CARTESIAN_POINT('',(67.75,2.7,-13.1966245684266));
#57928=CARTESIAN_POINT('',(95.,-13.47,-1.64959923845148E-15));
#57929=CARTESIAN_POINT('Origin',(95.,0.,0.));
#57930=CARTESIAN_POINT('',(67.75,-13.47,-1.64959923845148E-15));
#57931=CARTESIAN_POINT('Origin',(95.,0.,0.));
#57932=CARTESIAN_POINT('Origin',(118.5,2.7,-12.5));
#57933=CARTESIAN_POINT('',(95.,2.7,-6.25));
#57934=CARTESIAN_POINT('Origin',(95.,11.9,0.));
#57935=CARTESIAN_POINT('',(95.,-11.9,-1.45732969098535E-15));
#57936=CARTESIAN_POINT('Origin',(95.,0.,0.));
#57937=CARTESIAN_POINT('Origin',(95.5,0.,0.));
#57938=CARTESIAN_POINT('',(96.,-11.9,-1.45732969098535E-15));
#57939=CARTESIAN_POINT('Origin',(96.,0.,0.));
#57940=CARTESIAN_POINT('',(95.5,-11.9,-1.45732969098535E-15));
#57941=CARTESIAN_POINT('Origin',(96.25,0.,0.));
#57942=CARTESIAN_POINT('Ctrl Pts',(96.4460250000001,1.68935314532052,-12.5));
#57943=CARTESIAN_POINT('Ctrl Pts',(96.3046148851559,1.94289029309402E-15,
-12.5));
#57944=CARTESIAN_POINT('Ctrl Pts',(96.4460250000001,-1.68935314532052,-12.5));
#57945=CARTESIAN_POINT('',(96.25,-12.3,-1.50631556295124E-15));
#57946=CARTESIAN_POINT('Origin',(117.65,0.,0.));
#57947=CARTESIAN_POINT('',(117.65,-12.35,-1.51243879694698E-15));
#57948=CARTESIAN_POINT('Origin',(118.5,-2.7,-12.5));
#57949=CARTESIAN_POINT('Origin',(106.9,0.,0.));
#71601=UNCERTAINTY_MEASURE_WITH_UNIT(LENGTH_MEASURE(0.01),#71629,
'DISTANCE_ACCURACY_VALUE',
'Maximum model space distance between geometric entities at asserted c
onnectivities');
#71613=UNCERTAINTY_MEASURE_WITH_UNIT(LENGTH_MEASURE(0.01),#71629,
'DISTANCE_ACCURACY_VALUE',
'Maximum model space distance between geometric entities at asserted c
onnectivities');
#71616=(
GEOMETRIC_REPRESENTATION_CONTEXT(3)
GLOBAL_UNCERTAINTY_ASSIGNED_CONTEXT((#71601))
GLOBAL_UNIT_ASSIGNED_CONTEXT((#71629,#71631,#71632))
REPRESENTATION_CONTEXT('','3D')
);
#71628=(
GEOMETRIC_REPRESENTATION_CONTEXT(3)
GLOBAL_UNCERTAINTY_ASSIGNED_CONTEXT((#71613))
GLOBAL_UNIT_ASSIGNED_CONTEXT((#71629,#71631,#71632))
REPRESENTATION_CONTEXT('','3D')
);
#71629=(
LENGTH_UNIT()
NAMED_UNIT(*)
SI_UNIT(.MILLI.,.METRE.)
);
#71631=(
NAMED_UNIT(*)
PLANE_ANGLE_UNIT()
SI_UNIT($,.RADIAN.)
);
#71632=(
NAMED_UNIT(*)
SI_UNIT($,.STERADIAN.)
SOLID_ANGLE_UNIT()
);
#71635=SHAPE_DEFINITION_REPRESENTATION(#71649,#71684);
#71649=PRODUCT_DEFINITION_SHAPE('',$,#71699);
#71684=SHAPE_REPRESENTATION('',(#36166),#71616);
#71696=PRODUCT_DEFINITION_CONTEXT('part definition',#71740,'design');
#71699=PRODUCT_DEFINITION('2026-10-25-00-23-52-849',
'10_Spindle_84_3500lb',#71713,#71696);
#71713=PRODUCT_DEFINITION_FORMATION('',$,#71744);
#71740=APPLICATION_CONTEXT(
'Core Data for Automotive Mechanical Design Process');
#71741=PRODUCT_CONTEXT('part definition',#71740,'mechanical');
#71744=PRODUCT('2026-10-25-00-23-52-849','10_Spindle_84_3500lb',$,(#71741));
#71798=COLOUR_RGB('Light Blue',0.38,0.62,0.78);
#71799=FILL_AREA_STYLE_COLOUR('',#71798);
#71800=FILL_AREA_STYLE('',(#71799));
#71801=SURFACE_STYLE_FILL_AREA(#71800);
#71802=SURFACE_SIDE_STYLE('',(#71801));
#71803=SURFACE_STYLE_USAGE(.BOTH.,#71802);
#71804=PRESENTATION_STYLE_ASSIGNMENT((#71803));
ENDSEC;
END-ISO-10303-21;
